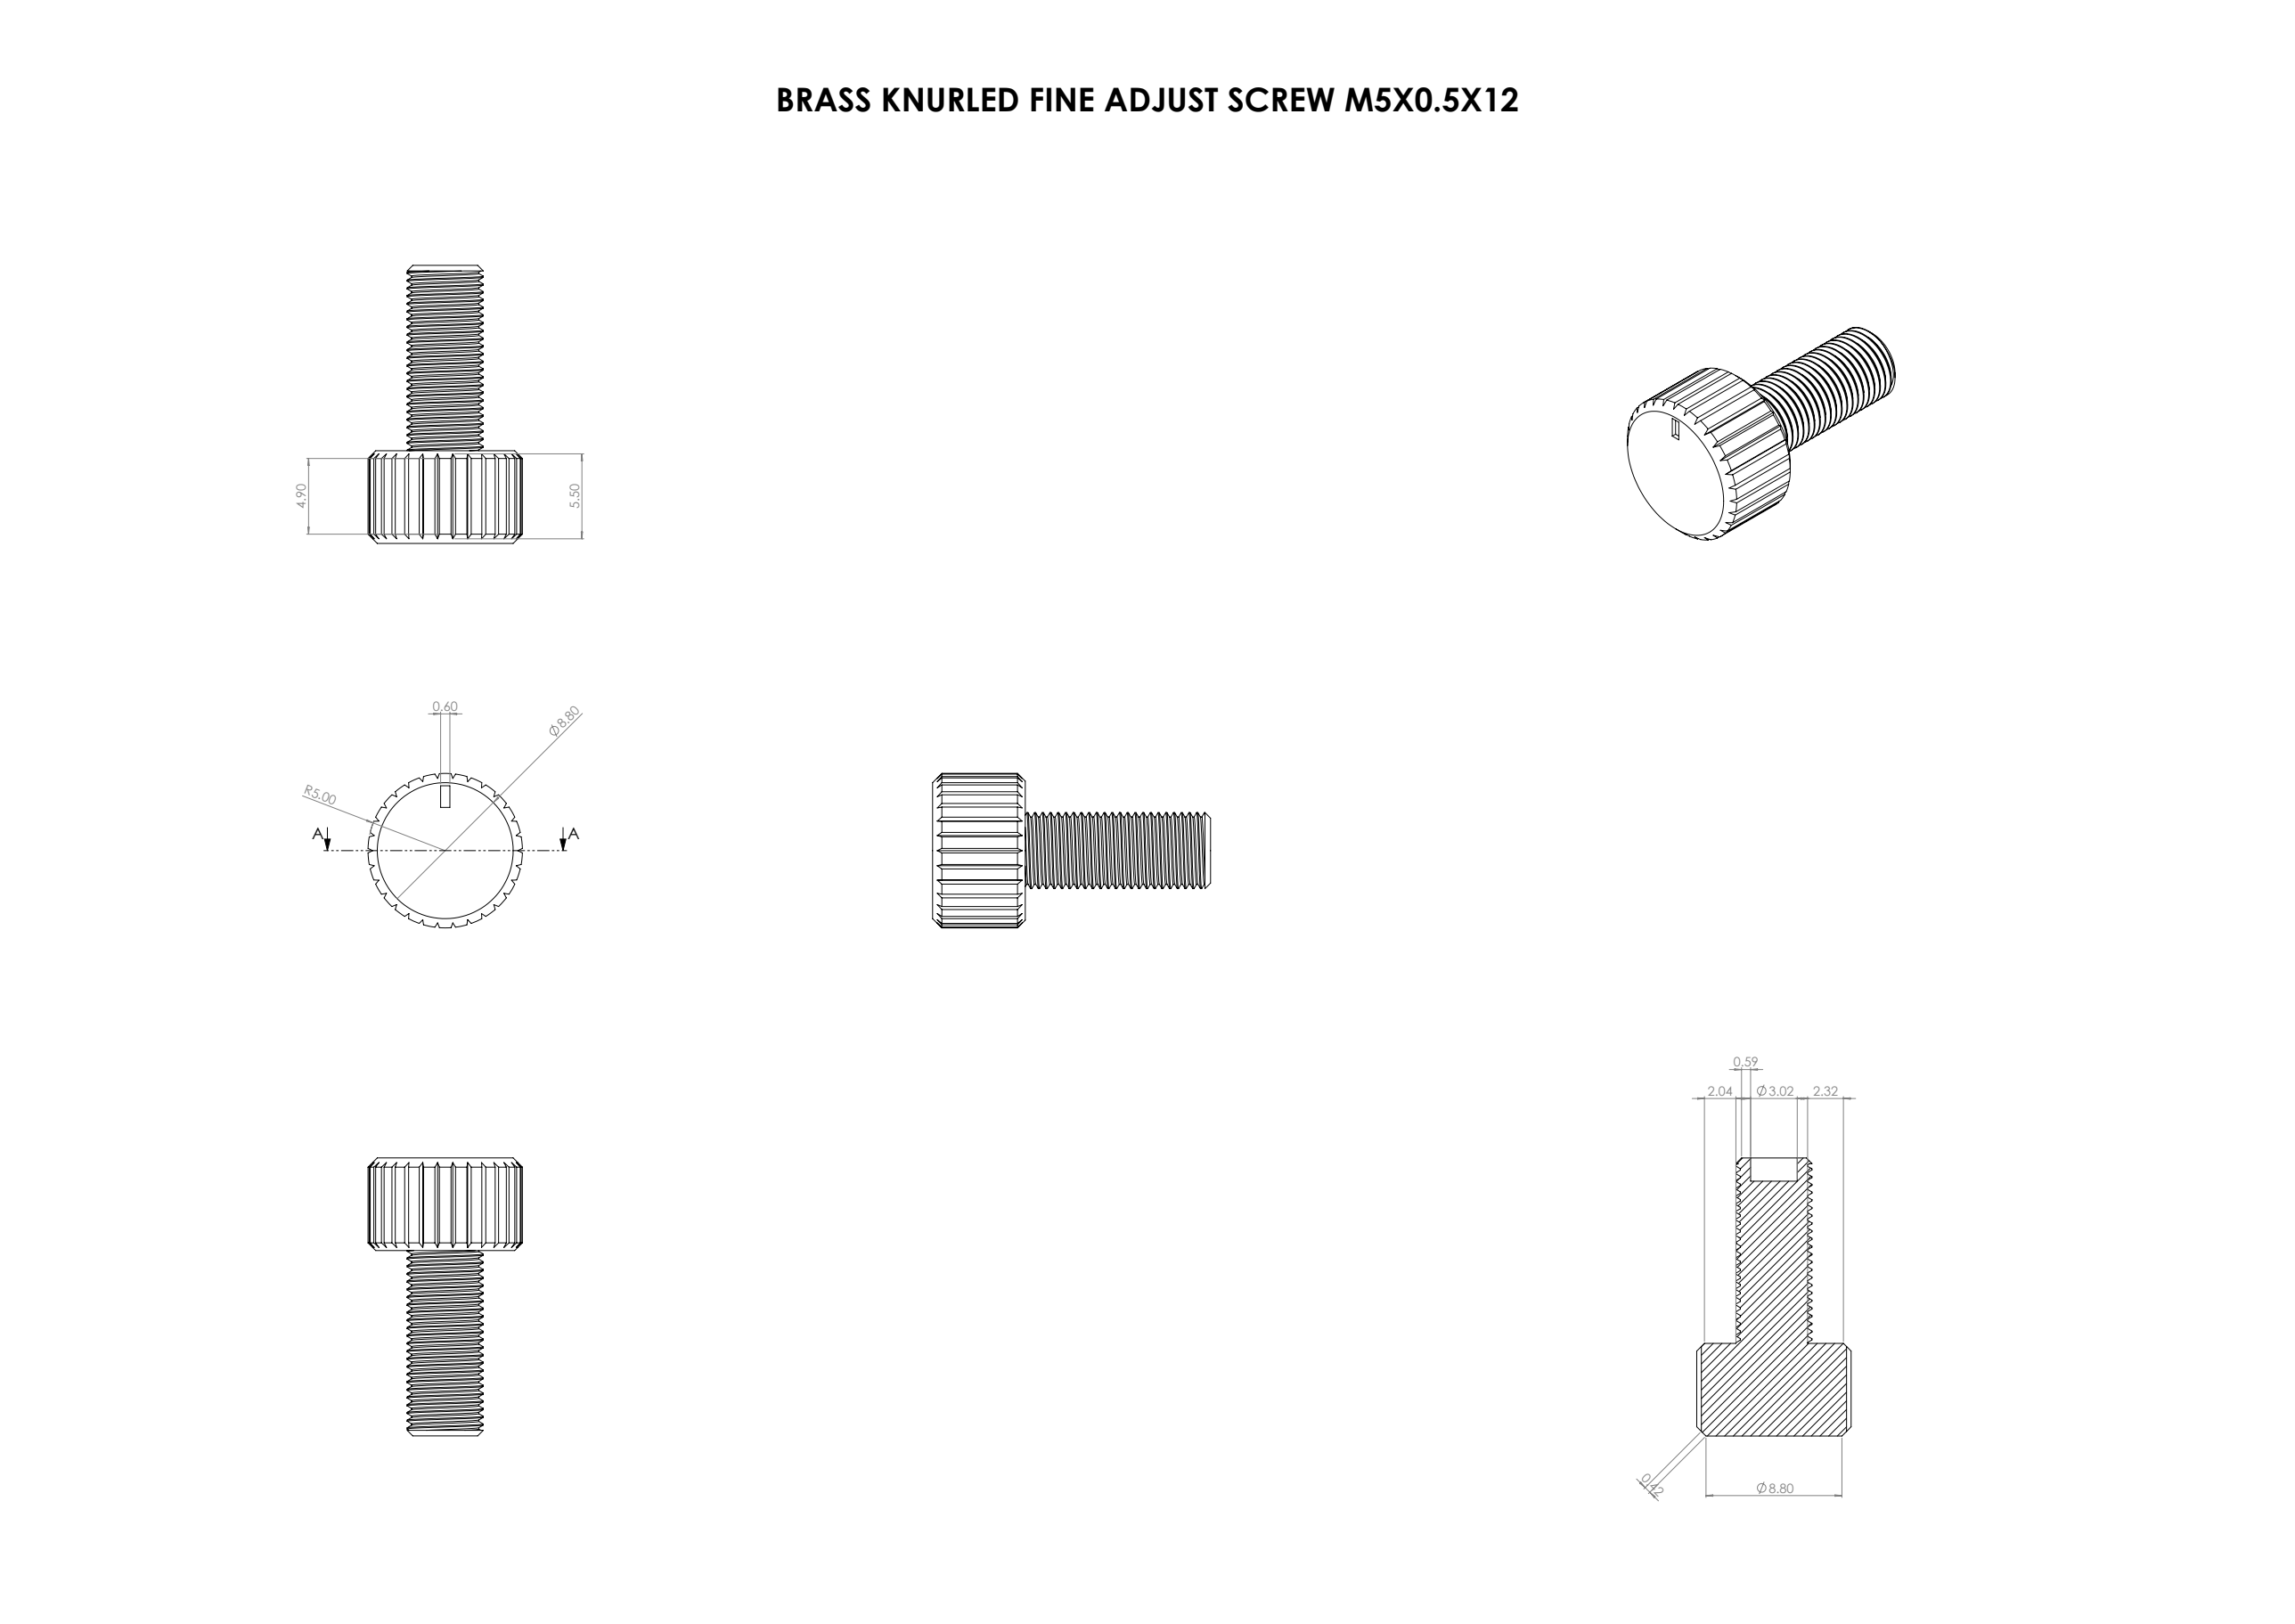
ISO-10303-21;
HEADER;
/* Generated by software containing ST-Developer
 * from STEP Tools, Inc. (www.steptools.com) 
 */

FILE_DESCRIPTION(
/* description */ (''),
/* implementation_level */ '2;1');

FILE_NAME(
/* name */ 
'08_Brass_Knurled_Fine_Adjust_Screw_M5x0.5x12.step',
/* time_stamp */ '2026-10-20T10:06:23-07:00',
/* author */ (''),
/* organization */ (''),
/* preprocessor_version */ 'ST-DEVELOPER v20.2',
/* originating_system */ 'Autodesk Translation Framework v15.15.0.0',
/* authorisation */ '');

FILE_SCHEMA (('AUTOMOTIVE_DESIGN { 1 0 10303 214 3 1 1 }'));
ENDSEC;

DATA;
#10=MECHANICAL_DESIGN_GEOMETRIC_PRESENTATION_REPRESENTATION('',(#469),#38611);
#132=(
BOUNDED_CURVE()
B_SPLINE_CURVE(2,(#30814,#30815,#30816),.UNSPECIFIED.,.F.,.F.)
B_SPLINE_CURVE_WITH_KNOTS((3,3),(0.0467199500563867,0.0898699663113549),
 .UNSPECIFIED.)
CURVE()
GEOMETRIC_REPRESENTATION_ITEM()
RATIONAL_B_SPLINE_CURVE((1.00126937543075,1.00122087809448,1.))
REPRESENTATION_ITEM('')
);
#133=(
BOUNDED_CURVE()
B_SPLINE_CURVE(2,(#30820,#30821,#30822),.UNSPECIFIED.,.F.,.F.)
B_SPLINE_CURVE_WITH_KNOTS((3,3),(0.,0.0436887632258073),.UNSPECIFIED.)
CURVE()
GEOMETRIC_REPRESENTATION_ITEM()
RATIONAL_B_SPLINE_CURVE((1.,1.00100330533763,1.00083425612165))
REPRESENTATION_ITEM('')
);
#134=(
BOUNDED_CURVE()
B_SPLINE_CURVE(2,(#30826,#30827,#30828),.UNSPECIFIED.,.F.,.F.)
B_SPLINE_CURVE_WITH_KNOTS((3,3),(0.,0.0431500162549626),.UNSPECIFIED.)
CURVE()
GEOMETRIC_REPRESENTATION_ITEM()
RATIONAL_B_SPLINE_CURVE((1.,1.00122087809439,1.00126937543066))
REPRESENTATION_ITEM('')
);
#135=(
BOUNDED_CURVE()
B_SPLINE_CURVE(2,(#30831,#30832,#30833),.UNSPECIFIED.,.F.,.F.)
B_SPLINE_CURVE_WITH_KNOTS((3,3),(0.0310892451912064,0.0747780084169829),
 .UNSPECIFIED.)
CURVE()
GEOMETRIC_REPRESENTATION_ITEM()
RATIONAL_B_SPLINE_CURVE((1.00083425612186,1.00100330533789,1.))
REPRESENTATION_ITEM('')
);
#136=(
BOUNDED_CURVE()
B_SPLINE_CURVE(2,(#30837,#30838,#30839),.UNSPECIFIED.,.F.,.F.)
B_SPLINE_CURVE_WITH_KNOTS((3,3),(0.0467199500564158,0.089869966311355),
 .UNSPECIFIED.)
CURVE()
GEOMETRIC_REPRESENTATION_ITEM()
RATIONAL_B_SPLINE_CURVE((1.00126937543096,1.00122087809468,1.))
REPRESENTATION_ITEM('')
);
#137=(
BOUNDED_CURVE()
B_SPLINE_CURVE(2,(#30843,#30844,#30845),.UNSPECIFIED.,.F.,.F.)
B_SPLINE_CURVE_WITH_KNOTS((3,3),(0.,0.043688763225805),.UNSPECIFIED.)
CURVE()
GEOMETRIC_REPRESENTATION_ITEM()
RATIONAL_B_SPLINE_CURVE((1.,1.00100330533789,1.00083425612186))
REPRESENTATION_ITEM('')
);
#138=(
BOUNDED_CURVE()
B_SPLINE_CURVE(2,(#30849,#30850,#30851),.UNSPECIFIED.,.F.,.F.)
B_SPLINE_CURVE_WITH_KNOTS((3,3),(0.,0.0431500162549483),.UNSPECIFIED.)
CURVE()
GEOMETRIC_REPRESENTATION_ITEM()
RATIONAL_B_SPLINE_CURVE((1.,1.00122087809469,1.00126937543097))
REPRESENTATION_ITEM('')
);
#139=(
BOUNDED_CURVE()
B_SPLINE_CURVE(2,(#30854,#30855,#30856),.UNSPECIFIED.,.F.,.F.)
B_SPLINE_CURVE_WITH_KNOTS((3,3),(0.0310892451911987,0.0747780084169828),
 .UNSPECIFIED.)
CURVE()
GEOMETRIC_REPRESENTATION_ITEM()
RATIONAL_B_SPLINE_CURVE((1.00083425612161,1.00100330533758,1.))
REPRESENTATION_ITEM('')
);
#140=(
BOUNDED_CURVE()
B_SPLINE_CURVE(2,(#30860,#30861,#30862),.UNSPECIFIED.,.F.,.F.)
B_SPLINE_CURVE_WITH_KNOTS((3,3),(0.0467199500563958,0.089869966311355),
 .UNSPECIFIED.)
CURVE()
GEOMETRIC_REPRESENTATION_ITEM()
RATIONAL_B_SPLINE_CURVE((1.00126937543073,1.00122087809446,1.))
REPRESENTATION_ITEM('')
);
#141=(
BOUNDED_CURVE()
B_SPLINE_CURVE(2,(#30866,#30867,#30868),.UNSPECIFIED.,.F.,.F.)
B_SPLINE_CURVE_WITH_KNOTS((3,3),(0.,0.0436887632258068),.UNSPECIFIED.)
CURVE()
GEOMETRIC_REPRESENTATION_ITEM()
RATIONAL_B_SPLINE_CURVE((1.,1.0010033053375,1.00083425612154))
REPRESENTATION_ITEM('')
);
#142=(
BOUNDED_CURVE()
B_SPLINE_CURVE(2,(#30872,#30873,#30874),.UNSPECIFIED.,.F.,.F.)
B_SPLINE_CURVE_WITH_KNOTS((3,3),(0.,0.0431500162549413),.UNSPECIFIED.)
CURVE()
GEOMETRIC_REPRESENTATION_ITEM()
RATIONAL_B_SPLINE_CURVE((1.,1.00122087809486,1.00126937543114))
REPRESENTATION_ITEM('')
);
#143=(
BOUNDED_CURVE()
B_SPLINE_CURVE(2,(#30877,#30878,#30879),.UNSPECIFIED.,.F.,.F.)
B_SPLINE_CURVE_WITH_KNOTS((3,3),(0.0310892451911471,0.0747780084169828),
 .UNSPECIFIED.)
CURVE()
GEOMETRIC_REPRESENTATION_ITEM()
RATIONAL_B_SPLINE_CURVE((1.00083425612202,1.00100330533808,1.))
REPRESENTATION_ITEM('')
);
#144=(
BOUNDED_CURVE()
B_SPLINE_CURVE(2,(#30883,#30884,#30885),.UNSPECIFIED.,.F.,.F.)
B_SPLINE_CURVE_WITH_KNOTS((3,3),(0.046719950056407,0.089869966311355),
 .UNSPECIFIED.)
CURVE()
GEOMETRIC_REPRESENTATION_ITEM()
RATIONAL_B_SPLINE_CURVE((1.00126937543088,1.0012208780946,1.))
REPRESENTATION_ITEM('')
);
#145=(
BOUNDED_CURVE()
B_SPLINE_CURVE(2,(#30889,#30890,#30891),.UNSPECIFIED.,.F.,.F.)
B_SPLINE_CURVE_WITH_KNOTS((3,3),(0.,0.0436887632257949),.UNSPECIFIED.)
CURVE()
GEOMETRIC_REPRESENTATION_ITEM()
RATIONAL_B_SPLINE_CURVE((1.,1.00100330533737,1.00083425612143))
REPRESENTATION_ITEM('')
);
#146=(
BOUNDED_CURVE()
B_SPLINE_CURVE(2,(#30895,#30896,#30897),.UNSPECIFIED.,.F.,.F.)
B_SPLINE_CURVE_WITH_KNOTS((3,3),(0.,0.0431500162549611),.UNSPECIFIED.)
CURVE()
GEOMETRIC_REPRESENTATION_ITEM()
RATIONAL_B_SPLINE_CURVE((1.,1.00122087809444,1.00126937543071))
REPRESENTATION_ITEM('')
);
#147=(
BOUNDED_CURVE()
B_SPLINE_CURVE(2,(#30900,#30901,#30902),.UNSPECIFIED.,.F.,.F.)
B_SPLINE_CURVE_WITH_KNOTS((3,3),(0.0310892451911564,0.0747780084169829),
 .UNSPECIFIED.)
CURVE()
GEOMETRIC_REPRESENTATION_ITEM()
RATIONAL_B_SPLINE_CURVE((1.00083425612184,1.00100330533786,1.))
REPRESENTATION_ITEM('')
);
#148=(
BOUNDED_CURVE()
B_SPLINE_CURVE(2,(#30906,#30907,#30908),.UNSPECIFIED.,.F.,.F.)
B_SPLINE_CURVE_WITH_KNOTS((3,3),(0.0467199500563991,0.089869966311355),
 .UNSPECIFIED.)
CURVE()
GEOMETRIC_REPRESENTATION_ITEM()
RATIONAL_B_SPLINE_CURVE((1.00126937543067,1.0012208780944,1.))
REPRESENTATION_ITEM('')
);
#149=(
BOUNDED_CURVE()
B_SPLINE_CURVE(2,(#30912,#30913,#30914),.UNSPECIFIED.,.F.,.F.)
B_SPLINE_CURVE_WITH_KNOTS((3,3),(0.,0.0436887632258358),.UNSPECIFIED.)
CURVE()
GEOMETRIC_REPRESENTATION_ITEM()
RATIONAL_B_SPLINE_CURVE((1.,1.0010033053379,1.00083425612187))
REPRESENTATION_ITEM('')
);
#150=(
BOUNDED_CURVE()
B_SPLINE_CURVE(2,(#30918,#30919,#30920),.UNSPECIFIED.,.F.,.F.)
B_SPLINE_CURVE_WITH_KNOTS((3,3),(0.,0.0431500162549541),.UNSPECIFIED.)
CURVE()
GEOMETRIC_REPRESENTATION_ITEM()
RATIONAL_B_SPLINE_CURVE((1.,1.00122087809508,1.00126937543137))
REPRESENTATION_ITEM('')
);
#151=(
BOUNDED_CURVE()
B_SPLINE_CURVE(2,(#30923,#30924,#30925),.UNSPECIFIED.,.F.,.F.)
B_SPLINE_CURVE_WITH_KNOTS((3,3),(0.0310892451911811,0.0747780084169827),
 .UNSPECIFIED.)
CURVE()
GEOMETRIC_REPRESENTATION_ITEM()
RATIONAL_B_SPLINE_CURVE((1.0008342561216,1.00100330533758,1.))
REPRESENTATION_ITEM('')
);
#152=(
BOUNDED_CURVE()
B_SPLINE_CURVE(2,(#30929,#30930,#30931),.UNSPECIFIED.,.F.,.F.)
B_SPLINE_CURVE_WITH_KNOTS((3,3),(0.0467199500563772,0.0898699663113549),
 .UNSPECIFIED.)
CURVE()
GEOMETRIC_REPRESENTATION_ITEM()
RATIONAL_B_SPLINE_CURVE((1.00126937543116,1.00122087809487,1.))
REPRESENTATION_ITEM('')
);
#153=(
BOUNDED_CURVE()
B_SPLINE_CURVE(2,(#30935,#30936,#30937),.UNSPECIFIED.,.F.,.F.)
B_SPLINE_CURVE_WITH_KNOTS((3,3),(0.,0.0436887632258276),.UNSPECIFIED.)
CURVE()
GEOMETRIC_REPRESENTATION_ITEM()
RATIONAL_B_SPLINE_CURVE((1.,1.00100330533759,1.00083425612161))
REPRESENTATION_ITEM('')
);
#154=(
BOUNDED_CURVE()
B_SPLINE_CURVE(2,(#30941,#30942,#30943),.UNSPECIFIED.,.F.,.F.)
B_SPLINE_CURVE_WITH_KNOTS((3,3),(0.,0.0431500162549563),.UNSPECIFIED.)
CURVE()
GEOMETRIC_REPRESENTATION_ITEM()
RATIONAL_B_SPLINE_CURVE((1.,1.00122087809465,1.00126937543093))
REPRESENTATION_ITEM('')
);
#155=(
BOUNDED_CURVE()
B_SPLINE_CURVE(2,(#30946,#30947,#30948),.UNSPECIFIED.,.F.,.F.)
B_SPLINE_CURVE_WITH_KNOTS((3,3),(0.0310892451911613,0.0747780084169828),
 .UNSPECIFIED.)
CURVE()
GEOMETRIC_REPRESENTATION_ITEM()
RATIONAL_B_SPLINE_CURVE((1.00083425612131,1.00100330533723,1.))
REPRESENTATION_ITEM('')
);
#156=(
BOUNDED_CURVE()
B_SPLINE_CURVE(2,(#30952,#30953,#30954),.UNSPECIFIED.,.F.,.F.)
B_SPLINE_CURVE_WITH_KNOTS((3,3),(0.0467199500563946,0.0898699663113547),
 .UNSPECIFIED.)
CURVE()
GEOMETRIC_REPRESENTATION_ITEM()
RATIONAL_B_SPLINE_CURVE((1.00126937543097,1.00122087809469,1.))
REPRESENTATION_ITEM('')
);
#157=(
BOUNDED_CURVE()
B_SPLINE_CURVE(2,(#30958,#30959,#30960),.UNSPECIFIED.,.F.,.F.)
B_SPLINE_CURVE_WITH_KNOTS((3,3),(0.,0.0436887632258045),.UNSPECIFIED.)
CURVE()
GEOMETRIC_REPRESENTATION_ITEM()
RATIONAL_B_SPLINE_CURVE((1.,1.00100330533793,1.00083425612189))
REPRESENTATION_ITEM('')
);
#158=(
BOUNDED_CURVE()
B_SPLINE_CURVE(2,(#30964,#30965,#30966),.UNSPECIFIED.,.F.,.F.)
B_SPLINE_CURVE_WITH_KNOTS((3,3),(0.,0.0431500162549573),.UNSPECIFIED.)
CURVE()
GEOMETRIC_REPRESENTATION_ITEM()
RATIONAL_B_SPLINE_CURVE((1.,1.00122087809474,1.00126937543102))
REPRESENTATION_ITEM('')
);
#159=(
BOUNDED_CURVE()
B_SPLINE_CURVE(2,(#30969,#30970,#30971),.UNSPECIFIED.,.F.,.F.)
B_SPLINE_CURVE_WITH_KNOTS((3,3),(0.0310892451911831,0.074778008416983),
 .UNSPECIFIED.)
CURVE()
GEOMETRIC_REPRESENTATION_ITEM()
RATIONAL_B_SPLINE_CURVE((1.00083425612233,1.00100330533846,1.))
REPRESENTATION_ITEM('')
);
#160=(
BOUNDED_CURVE()
B_SPLINE_CURVE(2,(#30975,#30976,#30977),.UNSPECIFIED.,.F.,.F.)
B_SPLINE_CURVE_WITH_KNOTS((3,3),(0.0467199500564136,0.0898699663113549),
 .UNSPECIFIED.)
CURVE()
GEOMETRIC_REPRESENTATION_ITEM()
RATIONAL_B_SPLINE_CURVE((1.00126937543068,1.00122087809441,1.))
REPRESENTATION_ITEM('')
);
#161=(
BOUNDED_CURVE()
B_SPLINE_CURVE(2,(#30981,#30982,#30983),.UNSPECIFIED.,.F.,.F.)
B_SPLINE_CURVE_WITH_KNOTS((3,3),(0.,0.0436887632258141),.UNSPECIFIED.)
CURVE()
GEOMETRIC_REPRESENTATION_ITEM()
RATIONAL_B_SPLINE_CURVE((1.,1.00100330533752,1.00083425612155))
REPRESENTATION_ITEM('')
);
#162=(
BOUNDED_CURVE()
B_SPLINE_CURVE(2,(#30987,#30988,#30989),.UNSPECIFIED.,.F.,.F.)
B_SPLINE_CURVE_WITH_KNOTS((3,3),(0.,0.0431500162549441),.UNSPECIFIED.)
CURVE()
GEOMETRIC_REPRESENTATION_ITEM()
RATIONAL_B_SPLINE_CURVE((1.,1.00122087809436,1.00126937543063))
REPRESENTATION_ITEM('')
);
#163=(
BOUNDED_CURVE()
B_SPLINE_CURVE(2,(#30992,#30993,#30994),.UNSPECIFIED.,.F.,.F.)
B_SPLINE_CURVE_WITH_KNOTS((3,3),(0.0310892451911682,0.0747780084169828),
 .UNSPECIFIED.)
CURVE()
GEOMETRIC_REPRESENTATION_ITEM()
RATIONAL_B_SPLINE_CURVE((1.00083425612141,1.00100330533735,1.))
REPRESENTATION_ITEM('')
);
#164=(
BOUNDED_CURVE()
B_SPLINE_CURVE(2,(#30998,#30999,#31000),.UNSPECIFIED.,.F.,.F.)
B_SPLINE_CURVE_WITH_KNOTS((3,3),(0.0467199500564218,0.0898699663113548),
 .UNSPECIFIED.)
CURVE()
GEOMETRIC_REPRESENTATION_ITEM()
RATIONAL_B_SPLINE_CURVE((1.00126937543122,1.00122087809493,1.))
REPRESENTATION_ITEM('')
);
#165=(
BOUNDED_CURVE()
B_SPLINE_CURVE(2,(#31004,#31005,#31006),.UNSPECIFIED.,.F.,.F.)
B_SPLINE_CURVE_WITH_KNOTS((3,3),(0.,0.0436887632257843),.UNSPECIFIED.)
CURVE()
GEOMETRIC_REPRESENTATION_ITEM()
RATIONAL_B_SPLINE_CURVE((1.,1.00100330533799,1.00083425612195))
REPRESENTATION_ITEM('')
);
#166=(
BOUNDED_CURVE()
B_SPLINE_CURVE(2,(#31010,#31011,#31012),.UNSPECIFIED.,.F.,.F.)
B_SPLINE_CURVE_WITH_KNOTS((3,3),(0.,0.0431500162549522),.UNSPECIFIED.)
CURVE()
GEOMETRIC_REPRESENTATION_ITEM()
RATIONAL_B_SPLINE_CURVE((1.,1.00122087809455,1.00126937543082))
REPRESENTATION_ITEM('')
);
#167=(
BOUNDED_CURVE()
B_SPLINE_CURVE(2,(#31015,#31016,#31017),.UNSPECIFIED.,.F.,.F.)
B_SPLINE_CURVE_WITH_KNOTS((3,3),(0.0310892451912127,0.0747780084169828),
 .UNSPECIFIED.)
CURVE()
GEOMETRIC_REPRESENTATION_ITEM()
RATIONAL_B_SPLINE_CURVE((1.000834256122,1.00100330533806,1.))
REPRESENTATION_ITEM('')
);
#168=(
BOUNDED_CURVE()
B_SPLINE_CURVE(2,(#31021,#31022,#31023),.UNSPECIFIED.,.F.,.F.)
B_SPLINE_CURVE_WITH_KNOTS((3,3),(0.046719950056375,0.0898699663113549),
 .UNSPECIFIED.)
CURVE()
GEOMETRIC_REPRESENTATION_ITEM()
RATIONAL_B_SPLINE_CURVE((1.00126937543081,1.00122087809453,1.))
REPRESENTATION_ITEM('')
);
#169=(
BOUNDED_CURVE()
B_SPLINE_CURVE(2,(#31027,#31028,#31029),.UNSPECIFIED.,.F.,.F.)
B_SPLINE_CURVE_WITH_KNOTS((3,3),(0.,0.043688763225798),.UNSPECIFIED.)
CURVE()
GEOMETRIC_REPRESENTATION_ITEM()
RATIONAL_B_SPLINE_CURVE((1.,1.00100330533766,1.00083425612167))
REPRESENTATION_ITEM('')
);
#170=(
BOUNDED_CURVE()
B_SPLINE_CURVE(2,(#31033,#31034,#31035),.UNSPECIFIED.,.F.,.F.)
B_SPLINE_CURVE_WITH_KNOTS((3,3),(0.,0.0431500162549388),.UNSPECIFIED.)
CURVE()
GEOMETRIC_REPRESENTATION_ITEM()
RATIONAL_B_SPLINE_CURVE((1.,1.00122087809441,1.00126937543068))
REPRESENTATION_ITEM('')
);
#171=(
BOUNDED_CURVE()
B_SPLINE_CURVE(2,(#31038,#31039,#31040),.UNSPECIFIED.,.F.,.F.)
B_SPLINE_CURVE_WITH_KNOTS((3,3),(0.031089245191172,0.0747780084169828),
 .UNSPECIFIED.)
CURVE()
GEOMETRIC_REPRESENTATION_ITEM()
RATIONAL_B_SPLINE_CURVE((1.00083425612203,1.00100330533809,1.))
REPRESENTATION_ITEM('')
);
#172=(
BOUNDED_CURVE()
B_SPLINE_CURVE(2,(#31044,#31045,#31046),.UNSPECIFIED.,.F.,.F.)
B_SPLINE_CURVE_WITH_KNOTS((3,3),(0.0467199500564012,0.0898699663113549),
 .UNSPECIFIED.)
CURVE()
GEOMETRIC_REPRESENTATION_ITEM()
RATIONAL_B_SPLINE_CURVE((1.00126937543067,1.00122087809441,1.))
REPRESENTATION_ITEM('')
);
#173=(
BOUNDED_CURVE()
B_SPLINE_CURVE(2,(#31050,#31051,#31052),.UNSPECIFIED.,.F.,.F.)
B_SPLINE_CURVE_WITH_KNOTS((3,3),(0.,0.0436887632258383),.UNSPECIFIED.)
CURVE()
GEOMETRIC_REPRESENTATION_ITEM()
RATIONAL_B_SPLINE_CURVE((1.,1.00100330533736,1.00083425612142))
REPRESENTATION_ITEM('')
);
#174=(
BOUNDED_CURVE()
B_SPLINE_CURVE(2,(#31056,#31057,#31058),.UNSPECIFIED.,.F.,.F.)
B_SPLINE_CURVE_WITH_KNOTS((3,3),(0.,0.0431500162549534),.UNSPECIFIED.)
CURVE()
GEOMETRIC_REPRESENTATION_ITEM()
RATIONAL_B_SPLINE_CURVE((1.,1.00122087809426,1.00126937543052))
REPRESENTATION_ITEM('')
);
#175=(
BOUNDED_CURVE()
B_SPLINE_CURVE(2,(#31061,#31062,#31063),.UNSPECIFIED.,.F.,.F.)
B_SPLINE_CURVE_WITH_KNOTS((3,3),(0.0310892451911742,0.074778008416983),
 .UNSPECIFIED.)
CURVE()
GEOMETRIC_REPRESENTATION_ITEM()
RATIONAL_B_SPLINE_CURVE((1.00083425612157,1.00100330533753,1.))
REPRESENTATION_ITEM('')
);
#176=(
BOUNDED_CURVE()
B_SPLINE_CURVE(2,(#31067,#31068,#31069),.UNSPECIFIED.,.F.,.F.)
B_SPLINE_CURVE_WITH_KNOTS((3,3),(0.0467199500564228,0.0898699663113548),
 .UNSPECIFIED.)
CURVE()
GEOMETRIC_REPRESENTATION_ITEM()
RATIONAL_B_SPLINE_CURVE((1.00126937543075,1.00122087809448,1.))
REPRESENTATION_ITEM('')
);
#177=(
BOUNDED_CURVE()
B_SPLINE_CURVE(2,(#31073,#31074,#31075),.UNSPECIFIED.,.F.,.F.)
B_SPLINE_CURVE_WITH_KNOTS((3,3),(0.,0.0436887632258167),.UNSPECIFIED.)
CURVE()
GEOMETRIC_REPRESENTATION_ITEM()
RATIONAL_B_SPLINE_CURVE((1.,1.0010033053373,1.00083425612137))
REPRESENTATION_ITEM('')
);
#178=(
BOUNDED_CURVE()
B_SPLINE_CURVE(2,(#31079,#31080,#31081),.UNSPECIFIED.,.F.,.F.)
B_SPLINE_CURVE_WITH_KNOTS((3,3),(0.,0.0431500162549855),.UNSPECIFIED.)
CURVE()
GEOMETRIC_REPRESENTATION_ITEM()
RATIONAL_B_SPLINE_CURVE((1.,1.00122087809442,1.00126937543069))
REPRESENTATION_ITEM('')
);
#179=(
BOUNDED_CURVE()
B_SPLINE_CURVE(2,(#31084,#31085,#31086),.UNSPECIFIED.,.F.,.F.)
B_SPLINE_CURVE_WITH_KNOTS((3,3),(0.0310892451911962,0.0747780084169828),
 .UNSPECIFIED.)
CURVE()
GEOMETRIC_REPRESENTATION_ITEM()
RATIONAL_B_SPLINE_CURVE((1.00083425612222,1.00100330533831,1.))
REPRESENTATION_ITEM('')
);
#180=(
BOUNDED_CURVE()
B_SPLINE_CURVE(2,(#31090,#31091,#31092),.UNSPECIFIED.,.F.,.F.)
B_SPLINE_CURVE_WITH_KNOTS((3,3),(0.0467199500564075,0.0898699663113548),
 .UNSPECIFIED.)
CURVE()
GEOMETRIC_REPRESENTATION_ITEM()
RATIONAL_B_SPLINE_CURVE((1.00126937543101,1.00122087809473,1.))
REPRESENTATION_ITEM('')
);
#181=(
BOUNDED_CURVE()
B_SPLINE_CURVE(2,(#31096,#31097,#31098),.UNSPECIFIED.,.F.,.F.)
B_SPLINE_CURVE_WITH_KNOTS((3,3),(0.,0.0436887632257957),.UNSPECIFIED.)
CURVE()
GEOMETRIC_REPRESENTATION_ITEM()
RATIONAL_B_SPLINE_CURVE((1.,1.00100330533777,1.00083425612177))
REPRESENTATION_ITEM('')
);
#182=(
BOUNDED_CURVE()
B_SPLINE_CURVE(2,(#31102,#31103,#31104),.UNSPECIFIED.,.F.,.F.)
B_SPLINE_CURVE_WITH_KNOTS((3,3),(0.,0.0431500162549319),.UNSPECIFIED.)
CURVE()
GEOMETRIC_REPRESENTATION_ITEM()
RATIONAL_B_SPLINE_CURVE((1.,1.00122087809489,1.00126937543118))
REPRESENTATION_ITEM('')
);
#183=(
BOUNDED_CURVE()
B_SPLINE_CURVE(2,(#31107,#31108,#31109),.UNSPECIFIED.,.F.,.F.)
B_SPLINE_CURVE_WITH_KNOTS((3,3),(0.0310892451911674,0.0747780084169828),
 .UNSPECIFIED.)
CURVE()
GEOMETRIC_REPRESENTATION_ITEM()
RATIONAL_B_SPLINE_CURVE((1.00083425612107,1.00100330533693,1.))
REPRESENTATION_ITEM('')
);
#184=(
BOUNDED_CURVE()
B_SPLINE_CURVE(2,(#31113,#31114,#31115),.UNSPECIFIED.,.F.,.F.)
B_SPLINE_CURVE_WITH_KNOTS((3,3),(0.0467199500564182,0.0898699663113548),
 .UNSPECIFIED.)
CURVE()
GEOMETRIC_REPRESENTATION_ITEM()
RATIONAL_B_SPLINE_CURVE((1.00126937543111,1.00122087809482,1.))
REPRESENTATION_ITEM('')
);
#185=(
BOUNDED_CURVE()
B_SPLINE_CURVE(2,(#31119,#31120,#31121),.UNSPECIFIED.,.F.,.F.)
B_SPLINE_CURVE_WITH_KNOTS((3,3),(0.,0.0436887632258121),.UNSPECIFIED.)
CURVE()
GEOMETRIC_REPRESENTATION_ITEM()
RATIONAL_B_SPLINE_CURVE((1.,1.00100330533764,1.00083425612165))
REPRESENTATION_ITEM('')
);
#186=(
BOUNDED_CURVE()
B_SPLINE_CURVE(2,(#31125,#31126,#31127),.UNSPECIFIED.,.F.,.F.)
B_SPLINE_CURVE_WITH_KNOTS((3,3),(0.,0.0431500162549636),.UNSPECIFIED.)
CURVE()
GEOMETRIC_REPRESENTATION_ITEM()
RATIONAL_B_SPLINE_CURVE((1.,1.0012208780943,1.00126937543056))
REPRESENTATION_ITEM('')
);
#187=(
BOUNDED_CURVE()
B_SPLINE_CURVE(2,(#31130,#31131,#31132),.UNSPECIFIED.,.F.,.F.)
B_SPLINE_CURVE_WITH_KNOTS((3,3),(0.0310892451911629,0.0747780084169827),
 .UNSPECIFIED.)
CURVE()
GEOMETRIC_REPRESENTATION_ITEM()
RATIONAL_B_SPLINE_CURVE((1.00083425612137,1.0010033053373,1.))
REPRESENTATION_ITEM('')
);
#188=(
BOUNDED_CURVE()
B_SPLINE_CURVE(2,(#31136,#31137,#31138),.UNSPECIFIED.,.F.,.F.)
B_SPLINE_CURVE_WITH_KNOTS((3,3),(0.0467199500564021,0.0898699663113548),
 .UNSPECIFIED.)
CURVE()
GEOMETRIC_REPRESENTATION_ITEM()
RATIONAL_B_SPLINE_CURVE((1.00126937543099,1.00122087809471,1.))
REPRESENTATION_ITEM('')
);
#189=(
BOUNDED_CURVE()
B_SPLINE_CURVE(2,(#31142,#31143,#31144),.UNSPECIFIED.,.F.,.F.)
B_SPLINE_CURVE_WITH_KNOTS((3,3),(0.,0.0436887632258091),.UNSPECIFIED.)
CURVE()
GEOMETRIC_REPRESENTATION_ITEM()
RATIONAL_B_SPLINE_CURVE((1.,1.00100330533755,1.00083425612158))
REPRESENTATION_ITEM('')
);
#190=(
BOUNDED_CURVE()
B_SPLINE_CURVE(2,(#31148,#31149,#31150),.UNSPECIFIED.,.F.,.F.)
B_SPLINE_CURVE_WITH_KNOTS((3,3),(0.,0.0431500162549568),.UNSPECIFIED.)
CURVE()
GEOMETRIC_REPRESENTATION_ITEM()
RATIONAL_B_SPLINE_CURVE((1.,1.00122087809472,1.00126937543101))
REPRESENTATION_ITEM('')
);
#191=(
BOUNDED_CURVE()
B_SPLINE_CURVE(2,(#31153,#31154,#31155),.UNSPECIFIED.,.F.,.F.)
B_SPLINE_CURVE_WITH_KNOTS((3,3),(0.0310892451911866,0.0747780084169829),
 .UNSPECIFIED.)
CURVE()
GEOMETRIC_REPRESENTATION_ITEM()
RATIONAL_B_SPLINE_CURVE((1.0008342561218,1.00100330533782,1.))
REPRESENTATION_ITEM('')
);
#192=(
BOUNDED_CURVE()
B_SPLINE_CURVE(2,(#31159,#31160,#31161),.UNSPECIFIED.,.F.,.F.)
B_SPLINE_CURVE_WITH_KNOTS((3,3),(0.0467199500564191,0.0898699663113548),
 .UNSPECIFIED.)
CURVE()
GEOMETRIC_REPRESENTATION_ITEM()
RATIONAL_B_SPLINE_CURVE((1.00126937543092,1.00122087809464,1.))
REPRESENTATION_ITEM('')
);
#193=(
BOUNDED_CURVE()
B_SPLINE_CURVE(2,(#31165,#31166,#31167),.UNSPECIFIED.,.F.,.F.)
B_SPLINE_CURVE_WITH_KNOTS((3,3),(0.,0.0436887632257914),.UNSPECIFIED.)
CURVE()
GEOMETRIC_REPRESENTATION_ITEM()
RATIONAL_B_SPLINE_CURVE((1.,1.00100330533698,1.0008342561211))
REPRESENTATION_ITEM('')
);
#194=(
BOUNDED_CURVE()
B_SPLINE_CURVE(2,(#31171,#31172,#31173),.UNSPECIFIED.,.F.,.F.)
B_SPLINE_CURVE_WITH_KNOTS((3,3),(0.,0.0431500162549322),.UNSPECIFIED.)
CURVE()
GEOMETRIC_REPRESENTATION_ITEM()
RATIONAL_B_SPLINE_CURVE((1.,1.00122087809449,1.00126937543076))
REPRESENTATION_ITEM('')
);
#195=(
BOUNDED_CURVE()
B_SPLINE_CURVE(2,(#31176,#31177,#31178),.UNSPECIFIED.,.F.,.F.)
B_SPLINE_CURVE_WITH_KNOTS((3,3),(0.0310892451911953,0.0747780084169828),
 .UNSPECIFIED.)
CURVE()
GEOMETRIC_REPRESENTATION_ITEM()
RATIONAL_B_SPLINE_CURVE((1.0008342561224,1.00100330533854,1.))
REPRESENTATION_ITEM('')
);
#196=(
BOUNDED_CURVE()
B_SPLINE_CURVE(2,(#31182,#31183,#31184),.UNSPECIFIED.,.F.,.F.)
B_SPLINE_CURVE_WITH_KNOTS((3,3),(0.0467199500564009,0.0898699663113548),
 .UNSPECIFIED.)
CURVE()
GEOMETRIC_REPRESENTATION_ITEM()
RATIONAL_B_SPLINE_CURVE((1.00126937543082,1.00122087809454,1.))
REPRESENTATION_ITEM('')
);
#197=(
BOUNDED_CURVE()
B_SPLINE_CURVE(2,(#31188,#31189,#31190),.UNSPECIFIED.,.F.,.F.)
B_SPLINE_CURVE_WITH_KNOTS((3,3),(0.,0.04368876322581),.UNSPECIFIED.)
CURVE()
GEOMETRIC_REPRESENTATION_ITEM()
RATIONAL_B_SPLINE_CURVE((1.,1.00100330533771,1.00083425612171))
REPRESENTATION_ITEM('')
);
#198=(
BOUNDED_CURVE()
B_SPLINE_CURVE(2,(#31194,#31195,#31196),.UNSPECIFIED.,.F.,.F.)
B_SPLINE_CURVE_WITH_KNOTS((3,3),(0.,0.0431500162549717),.UNSPECIFIED.)
CURVE()
GEOMETRIC_REPRESENTATION_ITEM()
RATIONAL_B_SPLINE_CURVE((1.,1.00122087809461,1.00126937543088))
REPRESENTATION_ITEM('')
);
#199=(
BOUNDED_CURVE()
B_SPLINE_CURVE(2,(#31199,#31200,#31201),.UNSPECIFIED.,.F.,.F.)
B_SPLINE_CURVE_WITH_KNOTS((3,3),(0.0310892451911806,0.0747780084169829),
 .UNSPECIFIED.)
CURVE()
GEOMETRIC_REPRESENTATION_ITEM()
RATIONAL_B_SPLINE_CURVE((1.00083425612159,1.00100330533756,1.))
REPRESENTATION_ITEM('')
);
#200=(
BOUNDED_CURVE()
B_SPLINE_CURVE(2,(#31205,#31206,#31207),.UNSPECIFIED.,.F.,.F.)
B_SPLINE_CURVE_WITH_KNOTS((3,3),(0.0467199500564204,0.0898699663113548),
 .UNSPECIFIED.)
CURVE()
GEOMETRIC_REPRESENTATION_ITEM()
RATIONAL_B_SPLINE_CURVE((1.00126937543083,1.00122087809455,1.))
REPRESENTATION_ITEM('')
);
#201=(
BOUNDED_CURVE()
B_SPLINE_CURVE(2,(#31211,#31212,#31213),.UNSPECIFIED.,.F.,.F.)
B_SPLINE_CURVE_WITH_KNOTS((3,3),(0.,0.0436887632258064),.UNSPECIFIED.)
CURVE()
GEOMETRIC_REPRESENTATION_ITEM()
RATIONAL_B_SPLINE_CURVE((1.,1.00100330533703,1.00083425612115))
REPRESENTATION_ITEM('')
);
#202=(
BOUNDED_CURVE()
B_SPLINE_CURVE(2,(#31217,#31218,#31219),.UNSPECIFIED.,.F.,.F.)
B_SPLINE_CURVE_WITH_KNOTS((3,3),(0.,0.0431500162549232),.UNSPECIFIED.)
CURVE()
GEOMETRIC_REPRESENTATION_ITEM()
RATIONAL_B_SPLINE_CURVE((1.,1.00122087809502,1.00126937543132))
REPRESENTATION_ITEM('')
);
#203=(
BOUNDED_CURVE()
B_SPLINE_CURVE(2,(#31222,#31223,#31224),.UNSPECIFIED.,.F.,.F.)
B_SPLINE_CURVE_WITH_KNOTS((3,3),(0.0310892451911708,0.0747780084169828),
 .UNSPECIFIED.)
CURVE()
GEOMETRIC_REPRESENTATION_ITEM()
RATIONAL_B_SPLINE_CURVE((1.00083425612115,1.00100330533704,1.))
REPRESENTATION_ITEM('')
);
#204=(
BOUNDED_CURVE()
B_SPLINE_CURVE(2,(#31228,#31229,#31230),.UNSPECIFIED.,.F.,.F.)
B_SPLINE_CURVE_WITH_KNOTS((3,3),(0.04671995005641,0.0898699663113547),
 .UNSPECIFIED.)
CURVE()
GEOMETRIC_REPRESENTATION_ITEM()
RATIONAL_B_SPLINE_CURVE((1.00126937543045,1.00122087809419,1.))
REPRESENTATION_ITEM('')
);
#205=(
BOUNDED_CURVE()
B_SPLINE_CURVE(2,(#31234,#31235,#31236),.UNSPECIFIED.,.F.,.F.)
B_SPLINE_CURVE_WITH_KNOTS((3,3),(0.,0.0436887632258215),.UNSPECIFIED.)
CURVE()
GEOMETRIC_REPRESENTATION_ITEM()
RATIONAL_B_SPLINE_CURVE((1.,1.00100330533736,1.00083425612143))
REPRESENTATION_ITEM('')
);
#206=(
BOUNDED_CURVE()
B_SPLINE_CURVE(2,(#31240,#31241,#31242),.UNSPECIFIED.,.F.,.F.)
B_SPLINE_CURVE_WITH_KNOTS((3,3),(0.,0.0431500162549405),.UNSPECIFIED.)
CURVE()
GEOMETRIC_REPRESENTATION_ITEM()
RATIONAL_B_SPLINE_CURVE((1.,1.00122087809483,1.00126937543112))
REPRESENTATION_ITEM('')
);
#207=(
BOUNDED_CURVE()
B_SPLINE_CURVE(2,(#31245,#31246,#31247),.UNSPECIFIED.,.F.,.F.)
B_SPLINE_CURVE_WITH_KNOTS((3,3),(0.0310892451911933,0.0747780084169829),
 .UNSPECIFIED.)
CURVE()
GEOMETRIC_REPRESENTATION_ITEM()
RATIONAL_B_SPLINE_CURVE((1.00083425612156,1.00100330533752,1.))
REPRESENTATION_ITEM('')
);
#208=(
BOUNDED_CURVE()
B_SPLINE_CURVE(2,(#31251,#31252,#31253),.UNSPECIFIED.,.F.,.F.)
B_SPLINE_CURVE_WITH_KNOTS((3,3),(0.0467199500564031,0.0898699663113549),
 .UNSPECIFIED.)
CURVE()
GEOMETRIC_REPRESENTATION_ITEM()
RATIONAL_B_SPLINE_CURVE((1.00126937543121,1.00122087809492,1.))
REPRESENTATION_ITEM('')
);
#209=(
BOUNDED_CURVE()
B_SPLINE_CURVE(2,(#31257,#31258,#31259),.UNSPECIFIED.,.F.,.F.)
B_SPLINE_CURVE_WITH_KNOTS((3,3),(0.,0.0436887632258158),.UNSPECIFIED.)
CURVE()
GEOMETRIC_REPRESENTATION_ITEM()
RATIONAL_B_SPLINE_CURVE((1.,1.0010033053384,1.00083425612229))
REPRESENTATION_ITEM('')
);
#210=(
BOUNDED_CURVE()
B_SPLINE_CURVE(2,(#31263,#31264,#31265),.UNSPECIFIED.,.F.,.F.)
B_SPLINE_CURVE_WITH_KNOTS((3,3),(0.,0.0431500162549452),.UNSPECIFIED.)
CURVE()
GEOMETRIC_REPRESENTATION_ITEM()
RATIONAL_B_SPLINE_CURVE((1.,1.00122087809455,1.00126937543082))
REPRESENTATION_ITEM('')
);
#211=(
BOUNDED_CURVE()
B_SPLINE_CURVE(2,(#31268,#31269,#31270),.UNSPECIFIED.,.F.,.F.)
B_SPLINE_CURVE_WITH_KNOTS((3,3),(0.0310892451911938,0.0747780084169828),
 .UNSPECIFIED.)
CURVE()
GEOMETRIC_REPRESENTATION_ITEM()
RATIONAL_B_SPLINE_CURVE((1.00083425612169,1.00100330533769,1.))
REPRESENTATION_ITEM('')
);
#212=(
BOUNDED_CURVE()
B_SPLINE_CURVE(2,(#31274,#31275,#31276),.UNSPECIFIED.,.F.,.F.)
B_SPLINE_CURVE_WITH_KNOTS((3,3),(0.0467199500564215,0.0898699663113548),
 .UNSPECIFIED.)
CURVE()
GEOMETRIC_REPRESENTATION_ITEM()
RATIONAL_B_SPLINE_CURVE((1.00126937543076,1.00122087809448,1.))
REPRESENTATION_ITEM('')
);
#213=(
BOUNDED_CURVE()
B_SPLINE_CURVE(2,(#31280,#31281,#31282),.UNSPECIFIED.,.F.,.F.)
B_SPLINE_CURVE_WITH_KNOTS((3,3),(0.,0.0436887632258074),.UNSPECIFIED.)
CURVE()
GEOMETRIC_REPRESENTATION_ITEM()
RATIONAL_B_SPLINE_CURVE((1.,1.00100330533774,1.00083425612174))
REPRESENTATION_ITEM('')
);
#214=(
BOUNDED_CURVE()
B_SPLINE_CURVE(2,(#31286,#31287,#31288),.UNSPECIFIED.,.F.,.F.)
B_SPLINE_CURVE_WITH_KNOTS((3,3),(0.,0.0431500162549509),.UNSPECIFIED.)
CURVE()
GEOMETRIC_REPRESENTATION_ITEM()
RATIONAL_B_SPLINE_CURVE((1.,1.00122087809425,1.00126937543051))
REPRESENTATION_ITEM('')
);
#215=(
BOUNDED_CURVE()
B_SPLINE_CURVE(2,(#31291,#31292,#31293),.UNSPECIFIED.,.F.,.F.)
B_SPLINE_CURVE_WITH_KNOTS((3,3),(0.0310892451912129,0.0747780084169828),
 .UNSPECIFIED.)
CURVE()
GEOMETRIC_REPRESENTATION_ITEM()
RATIONAL_B_SPLINE_CURVE((1.00083425612163,1.00100330533761,1.))
REPRESENTATION_ITEM('')
);
#216=(
BOUNDED_CURVE()
B_SPLINE_CURVE(2,(#31297,#31298,#31299),.UNSPECIFIED.,.F.,.F.)
B_SPLINE_CURVE_WITH_KNOTS((3,3),(0.0467199500564181,0.0898699663113547),
 .UNSPECIFIED.)
CURVE()
GEOMETRIC_REPRESENTATION_ITEM()
RATIONAL_B_SPLINE_CURVE((1.00126937543066,1.0012208780944,1.))
REPRESENTATION_ITEM('')
);
#217=(
BOUNDED_CURVE()
B_SPLINE_CURVE(2,(#31303,#31304,#31305),.UNSPECIFIED.,.F.,.F.)
B_SPLINE_CURVE_WITH_KNOTS((3,3),(0.,0.0436887632258064),.UNSPECIFIED.)
CURVE()
GEOMETRIC_REPRESENTATION_ITEM()
RATIONAL_B_SPLINE_CURVE((1.,1.00100330533711,1.00083425612121))
REPRESENTATION_ITEM('')
);
#218=(
BOUNDED_CURVE()
B_SPLINE_CURVE(2,(#31309,#31310,#31311),.UNSPECIFIED.,.F.,.F.)
B_SPLINE_CURVE_WITH_KNOTS((3,3),(0.,0.0431500162549468),.UNSPECIFIED.)
CURVE()
GEOMETRIC_REPRESENTATION_ITEM()
RATIONAL_B_SPLINE_CURVE((1.,1.00122087809451,1.00126937543078))
REPRESENTATION_ITEM('')
);
#219=(
BOUNDED_CURVE()
B_SPLINE_CURVE(2,(#31314,#31315,#31316),.UNSPECIFIED.,.F.,.F.)
B_SPLINE_CURVE_WITH_KNOTS((3,3),(0.0310892451911651,0.0747780084169829),
 .UNSPECIFIED.)
CURVE()
GEOMETRIC_REPRESENTATION_ITEM()
RATIONAL_B_SPLINE_CURVE((1.00083425612205,1.00100330533812,1.))
REPRESENTATION_ITEM('')
);
#220=(
BOUNDED_CURVE()
B_SPLINE_CURVE(2,(#31320,#31321,#31322),.UNSPECIFIED.,.F.,.F.)
B_SPLINE_CURVE_WITH_KNOTS((3,3),(0.0467199500563987,0.0898699663113548),
 .UNSPECIFIED.)
CURVE()
GEOMETRIC_REPRESENTATION_ITEM()
RATIONAL_B_SPLINE_CURVE((1.00126937543082,1.00122087809454,1.))
REPRESENTATION_ITEM('')
);
#221=(
BOUNDED_CURVE()
B_SPLINE_CURVE(2,(#31326,#31327,#31328),.UNSPECIFIED.,.F.,.F.)
B_SPLINE_CURVE_WITH_KNOTS((3,3),(0.,0.0436887632257942),.UNSPECIFIED.)
CURVE()
GEOMETRIC_REPRESENTATION_ITEM()
RATIONAL_B_SPLINE_CURVE((1.,1.0010033053377,1.0008342561217))
REPRESENTATION_ITEM('')
);
#222=(
BOUNDED_CURVE()
B_SPLINE_CURVE(2,(#31332,#31333,#31334),.UNSPECIFIED.,.F.,.F.)
B_SPLINE_CURVE_WITH_KNOTS((3,3),(0.,0.0431500162549576),.UNSPECIFIED.)
CURVE()
GEOMETRIC_REPRESENTATION_ITEM()
RATIONAL_B_SPLINE_CURVE((1.,1.00122087809465,1.00126937543093))
REPRESENTATION_ITEM('')
);
#223=(
BOUNDED_CURVE()
B_SPLINE_CURVE(2,(#31337,#31338,#31339),.UNSPECIFIED.,.F.,.F.)
B_SPLINE_CURVE_WITH_KNOTS((3,3),(0.0310892451911712,0.0747780084169828),
 .UNSPECIFIED.)
CURVE()
GEOMETRIC_REPRESENTATION_ITEM()
RATIONAL_B_SPLINE_CURVE((1.00083425612158,1.00100330533755,1.))
REPRESENTATION_ITEM('')
);
#224=(
BOUNDED_CURVE()
B_SPLINE_CURVE(2,(#31343,#31344,#31345),.UNSPECIFIED.,.F.,.F.)
B_SPLINE_CURVE_WITH_KNOTS((3,3),(0.0467199500563997,0.0898699663113548),
 .UNSPECIFIED.)
CURVE()
GEOMETRIC_REPRESENTATION_ITEM()
RATIONAL_B_SPLINE_CURVE((1.00126937543088,1.0012208780946,1.))
REPRESENTATION_ITEM('')
);
#225=(
BOUNDED_CURVE()
B_SPLINE_CURVE(2,(#31349,#31350,#31351),.UNSPECIFIED.,.F.,.F.)
B_SPLINE_CURVE_WITH_KNOTS((3,3),(0.,0.0436887632257912),.UNSPECIFIED.)
CURVE()
GEOMETRIC_REPRESENTATION_ITEM()
RATIONAL_B_SPLINE_CURVE((1.,1.00100330533807,1.00083425612201))
REPRESENTATION_ITEM('')
);
#226=(
BOUNDED_CURVE()
B_SPLINE_CURVE(2,(#31355,#31356,#31357),.UNSPECIFIED.,.F.,.F.)
B_SPLINE_CURVE_WITH_KNOTS((3,3),(0.,0.0431500162549322),.UNSPECIFIED.)
CURVE()
GEOMETRIC_REPRESENTATION_ITEM()
RATIONAL_B_SPLINE_CURVE((1.,1.00122087809449,1.00126937543076))
REPRESENTATION_ITEM('')
);
#227=(
BOUNDED_CURVE()
B_SPLINE_CURVE(2,(#31360,#31361,#31362),.UNSPECIFIED.,.F.,.F.)
B_SPLINE_CURVE_WITH_KNOTS((3,3),(0.0310892451911953,0.0747780084169828),
 .UNSPECIFIED.)
CURVE()
GEOMETRIC_REPRESENTATION_ITEM()
RATIONAL_B_SPLINE_CURVE((1.0008342561224,1.00100330533854,1.))
REPRESENTATION_ITEM('')
);
#228=(
BOUNDED_CURVE()
B_SPLINE_CURVE(2,(#31366,#31367,#31368),.UNSPECIFIED.,.F.,.F.)
B_SPLINE_CURVE_WITH_KNOTS((3,3),(0.0467199500563888,0.0898699663113548),
 .UNSPECIFIED.)
CURVE()
GEOMETRIC_REPRESENTATION_ITEM()
RATIONAL_B_SPLINE_CURVE((1.0012693754306,1.00122087809433,1.))
REPRESENTATION_ITEM('')
);
#229=(
BOUNDED_CURVE()
B_SPLINE_CURVE(2,(#31372,#31373,#31374),.UNSPECIFIED.,.F.,.F.)
B_SPLINE_CURVE_WITH_KNOTS((3,3),(0.,0.0436887632258443),.UNSPECIFIED.)
CURVE()
GEOMETRIC_REPRESENTATION_ITEM()
RATIONAL_B_SPLINE_CURVE((1.,1.00100330533721,1.0008342561213))
REPRESENTATION_ITEM('')
);
#230=(
BOUNDED_CURVE()
B_SPLINE_CURVE(2,(#31378,#31379,#31380),.UNSPECIFIED.,.F.,.F.)
B_SPLINE_CURVE_WITH_KNOTS((3,3),(0.,0.0431500162549717),.UNSPECIFIED.)
CURVE()
GEOMETRIC_REPRESENTATION_ITEM()
RATIONAL_B_SPLINE_CURVE((1.,1.00122087809461,1.00126937543088))
REPRESENTATION_ITEM('')
);
#231=(
BOUNDED_CURVE()
B_SPLINE_CURVE(2,(#31383,#31384,#31385),.UNSPECIFIED.,.F.,.F.)
B_SPLINE_CURVE_WITH_KNOTS((3,3),(0.0310892451911806,0.0747780084169829),
 .UNSPECIFIED.)
CURVE()
GEOMETRIC_REPRESENTATION_ITEM()
RATIONAL_B_SPLINE_CURVE((1.00083425612159,1.00100330533756,1.))
REPRESENTATION_ITEM('')
);
#232=(
BOUNDED_CURVE()
B_SPLINE_CURVE(2,(#31389,#31390,#31391),.UNSPECIFIED.,.F.,.F.)
B_SPLINE_CURVE_WITH_KNOTS((3,3),(0.0467199500563954,0.0898699663113548),
 .UNSPECIFIED.)
CURVE()
GEOMETRIC_REPRESENTATION_ITEM()
RATIONAL_B_SPLINE_CURVE((1.00126937543089,1.00122087809461,1.))
REPRESENTATION_ITEM('')
);
#233=(
BOUNDED_CURVE()
B_SPLINE_CURVE(2,(#31395,#31396,#31397),.UNSPECIFIED.,.F.,.F.)
B_SPLINE_CURVE_WITH_KNOTS((3,3),(0.,0.0436887632258089),.UNSPECIFIED.)
CURVE()
GEOMETRIC_REPRESENTATION_ITEM()
RATIONAL_B_SPLINE_CURVE((1.,1.00100330533773,1.00083425612173))
REPRESENTATION_ITEM('')
);
#234=(
BOUNDED_CURVE()
B_SPLINE_CURVE(2,(#31401,#31402,#31403),.UNSPECIFIED.,.F.,.F.)
B_SPLINE_CURVE_WITH_KNOTS((3,3),(0.,0.0431500162549499),.UNSPECIFIED.)
CURVE()
GEOMETRIC_REPRESENTATION_ITEM()
RATIONAL_B_SPLINE_CURVE((1.,1.00122087809471,1.00126937543099))
REPRESENTATION_ITEM('')
);
#235=(
BOUNDED_CURVE()
B_SPLINE_CURVE(2,(#31406,#31407,#31408),.UNSPECIFIED.,.F.,.F.)
B_SPLINE_CURVE_WITH_KNOTS((3,3),(0.0310892451911691,0.0747780084169828),
 .UNSPECIFIED.)
CURVE()
GEOMETRIC_REPRESENTATION_ITEM()
RATIONAL_B_SPLINE_CURVE((1.0008342561213,1.00100330533722,1.))
REPRESENTATION_ITEM('')
);
#236=(
BOUNDED_CURVE()
B_SPLINE_CURVE(2,(#31412,#31413,#31414),.UNSPECIFIED.,.F.,.F.)
B_SPLINE_CURVE_WITH_KNOTS((3,3),(0.0467199500563946,0.0898699663113549),
 .UNSPECIFIED.)
CURVE()
GEOMETRIC_REPRESENTATION_ITEM()
RATIONAL_B_SPLINE_CURVE((1.00126937543091,1.00122087809463,1.))
REPRESENTATION_ITEM('')
);
#237=(
BOUNDED_CURVE()
B_SPLINE_CURVE(2,(#31418,#31419,#31420),.UNSPECIFIED.,.F.,.F.)
B_SPLINE_CURVE_WITH_KNOTS((3,3),(0.,0.0436887632258018),.UNSPECIFIED.)
CURVE()
GEOMETRIC_REPRESENTATION_ITEM()
RATIONAL_B_SPLINE_CURVE((1.,1.00100330533801,1.00083425612196))
REPRESENTATION_ITEM('')
);
#238=(
BOUNDED_CURVE()
B_SPLINE_CURVE(2,(#31424,#31425,#31426),.UNSPECIFIED.,.F.,.F.)
B_SPLINE_CURVE_WITH_KNOTS((3,3),(0.,0.0431500162549446),.UNSPECIFIED.)
CURVE()
GEOMETRIC_REPRESENTATION_ITEM()
RATIONAL_B_SPLINE_CURVE((1.,1.00122087809491,1.00126937543119))
REPRESENTATION_ITEM('')
);
#239=(
BOUNDED_CURVE()
B_SPLINE_CURVE(2,(#31429,#31430,#31431),.UNSPECIFIED.,.F.,.F.)
B_SPLINE_CURVE_WITH_KNOTS((3,3),(0.0310892451912006,0.0747780084169829),
 .UNSPECIFIED.)
CURVE()
GEOMETRIC_REPRESENTATION_ITEM()
RATIONAL_B_SPLINE_CURVE((1.00083425612167,1.00100330533765,1.))
REPRESENTATION_ITEM('')
);
#240=(
BOUNDED_CURVE()
B_SPLINE_CURVE(2,(#31435,#31436,#31437),.UNSPECIFIED.,.F.,.F.)
B_SPLINE_CURVE_WITH_KNOTS((3,3),(0.0467199500564005,0.0898699663113549),
 .UNSPECIFIED.)
CURVE()
GEOMETRIC_REPRESENTATION_ITEM()
RATIONAL_B_SPLINE_CURVE((1.00126937543091,1.00122087809463,1.))
REPRESENTATION_ITEM('')
);
#241=(
BOUNDED_CURVE()
B_SPLINE_CURVE(2,(#31441,#31442,#31443),.UNSPECIFIED.,.F.,.F.)
B_SPLINE_CURVE_WITH_KNOTS((3,3),(0.,0.0436887632257904),.UNSPECIFIED.)
CURVE()
GEOMETRIC_REPRESENTATION_ITEM()
RATIONAL_B_SPLINE_CURVE((1.,1.00100330533768,1.00083425612169))
REPRESENTATION_ITEM('')
);
#242=(
BOUNDED_CURVE()
B_SPLINE_CURVE(2,(#31447,#31448,#31449),.UNSPECIFIED.,.F.,.F.)
B_SPLINE_CURVE_WITH_KNOTS((3,3),(0.,0.0431500162549576),.UNSPECIFIED.)
CURVE()
GEOMETRIC_REPRESENTATION_ITEM()
RATIONAL_B_SPLINE_CURVE((1.,1.00122087809446,1.00126937543073))
REPRESENTATION_ITEM('')
);
#243=(
BOUNDED_CURVE()
B_SPLINE_CURVE(2,(#31452,#31453,#31454),.UNSPECIFIED.,.F.,.F.)
B_SPLINE_CURVE_WITH_KNOTS((3,3),(0.0310892451911633,0.0747780084169828),
 .UNSPECIFIED.)
CURVE()
GEOMETRIC_REPRESENTATION_ITEM()
RATIONAL_B_SPLINE_CURVE((1.00083425612268,1.00100330533887,1.))
REPRESENTATION_ITEM('')
);
#244=(
BOUNDED_CURVE()
B_SPLINE_CURVE(2,(#31458,#31459,#31460),.UNSPECIFIED.,.F.,.F.)
B_SPLINE_CURVE_WITH_KNOTS((3,3),(0.0467199500564166,0.089869966311355),
 .UNSPECIFIED.)
CURVE()
GEOMETRIC_REPRESENTATION_ITEM()
RATIONAL_B_SPLINE_CURVE((1.00126937543126,1.00122087809497,1.))
REPRESENTATION_ITEM('')
);
#245=(
BOUNDED_CURVE()
B_SPLINE_CURVE(2,(#31464,#31465,#31466),.UNSPECIFIED.,.F.,.F.)
B_SPLINE_CURVE_WITH_KNOTS((3,3),(0.,0.0436887632258151),.UNSPECIFIED.)
CURVE()
GEOMETRIC_REPRESENTATION_ITEM()
RATIONAL_B_SPLINE_CURVE((1.,1.00100330533817,1.00083425612209))
REPRESENTATION_ITEM('')
);
#246=(
BOUNDED_CURVE()
B_SPLINE_CURVE(2,(#31470,#31471,#31472),.UNSPECIFIED.,.F.,.F.)
B_SPLINE_CURVE_WITH_KNOTS((3,3),(0.,0.0431500162549457),.UNSPECIFIED.)
CURVE()
GEOMETRIC_REPRESENTATION_ITEM()
RATIONAL_B_SPLINE_CURVE((1.,1.00122087809449,1.00126937543076))
REPRESENTATION_ITEM('')
);
#247=(
BOUNDED_CURVE()
B_SPLINE_CURVE(2,(#31475,#31476,#31477),.UNSPECIFIED.,.F.,.F.)
B_SPLINE_CURVE_WITH_KNOTS((3,3),(0.0310892451911691,0.0747780084169829),
 .UNSPECIFIED.)
CURVE()
GEOMETRIC_REPRESENTATION_ITEM()
RATIONAL_B_SPLINE_CURVE((1.00083425612148,1.00100330533743,1.))
REPRESENTATION_ITEM('')
);
#248=(
BOUNDED_CURVE()
B_SPLINE_CURVE(2,(#31481,#31482,#31483),.UNSPECIFIED.,.F.,.F.)
B_SPLINE_CURVE_WITH_KNOTS((3,3),(0.0467199500564313,0.089869966311355),
 .UNSPECIFIED.)
CURVE()
GEOMETRIC_REPRESENTATION_ITEM()
RATIONAL_B_SPLINE_CURVE((1.00126937543075,1.00122087809448,1.))
REPRESENTATION_ITEM('')
);
#249=(
BOUNDED_CURVE()
B_SPLINE_CURVE(2,(#31487,#31488,#31489),.UNSPECIFIED.,.F.,.F.)
B_SPLINE_CURVE_WITH_KNOTS((3,3),(0.,0.0436887632257837),.UNSPECIFIED.)
CURVE()
GEOMETRIC_REPRESENTATION_ITEM()
RATIONAL_B_SPLINE_CURVE((1.,1.00100330533754,1.00083425612157))
REPRESENTATION_ITEM('')
);
#250=(
BOUNDED_CURVE()
B_SPLINE_CURVE(2,(#31493,#31494,#31495),.UNSPECIFIED.,.F.,.F.)
B_SPLINE_CURVE_WITH_KNOTS((3,3),(0.,0.043150016254948),.UNSPECIFIED.)
CURVE()
GEOMETRIC_REPRESENTATION_ITEM()
RATIONAL_B_SPLINE_CURVE((1.,1.00122087809439,1.00126937543066))
REPRESENTATION_ITEM('')
);
#251=(
BOUNDED_CURVE()
B_SPLINE_CURVE(2,(#31498,#31499,#31500),.UNSPECIFIED.,.F.,.F.)
B_SPLINE_CURVE_WITH_KNOTS((3,3),(0.0310892451912077,0.0747780084169828),
 .UNSPECIFIED.)
CURVE()
GEOMETRIC_REPRESENTATION_ITEM()
RATIONAL_B_SPLINE_CURVE((1.00083425612152,1.00100330533748,1.))
REPRESENTATION_ITEM('')
);
#441=SHAPE_REPRESENTATION_RELATIONSHIP('SRR','None',#38677,#455);
#455=ADVANCED_BREP_SHAPE_REPRESENTATION('',(#483),#38606);
#469=STYLED_ITEM('',(#38885),#483);
#483=MANIFOLD_SOLID_BREP('Adjuster',#16243);
#503=B_SPLINE_SURFACE_WITH_KNOTS('',3,3,((#29345,#29346,#29347,#29348,#29349,
#29350,#29351,#29352,#29353,#29354,#29355,#29356,#29357,#29358,#29359,#29360,
#29361,#29362,#29363,#29364,#29365,#29366,#29367,#29368,#29369,#29370,#29371,
#29372,#29373,#29374,#29375,#29376,#29377,#29378,#29379,#29380,#29381,#29382,
#29383,#29384,#29385,#29386,#29387,#29388,#29389,#29390,#29391,#29392,#29393,
#29394,#29395,#29396,#29397,#29398,#29399,#29400,#29401,#29402,#29403,#29404,
#29405,#29406,#29407,#29408,#29409,#29410,#29411,#29412,#29413,#29414,#29415,
#29416,#29417,#29418,#29419,#29420,#29421,#29422,#29423,#29424,#29425,#29426,
#29427,#29428,#29429,#29430,#29431,#29432,#29433,#29434,#29435,#29436,#29437,
#29438,#29439,#29440,#29441,#29442,#29443,#29444,#29445,#29446,#29447,#29448,
#29449,#29450,#29451,#29452,#29453,#29454,#29455,#29456,#29457,#29458,#29459,
#29460,#29461,#29462,#29463,#29464,#29465,#29466,#29467,#29468,#29469,#29470,
#29471,#29472,#29473,#29474,#29475,#29476,#29477,#29478,#29479,#29480,#29481,
#29482,#29483,#29484,#29485,#29486,#29487,#29488,#29489,#29490,#29491,#29492,
#29493,#29494,#29495,#29496),(#29497,#29498,#29499,#29500,#29501,#29502,
#29503,#29504,#29505,#29506,#29507,#29508,#29509,#29510,#29511,#29512,#29513,
#29514,#29515,#29516,#29517,#29518,#29519,#29520,#29521,#29522,#29523,#29524,
#29525,#29526,#29527,#29528,#29529,#29530,#29531,#29532,#29533,#29534,#29535,
#29536,#29537,#29538,#29539,#29540,#29541,#29542,#29543,#29544,#29545,#29546,
#29547,#29548,#29549,#29550,#29551,#29552,#29553,#29554,#29555,#29556,#29557,
#29558,#29559,#29560,#29561,#29562,#29563,#29564,#29565,#29566,#29567,#29568,
#29569,#29570,#29571,#29572,#29573,#29574,#29575,#29576,#29577,#29578,#29579,
#29580,#29581,#29582,#29583,#29584,#29585,#29586,#29587,#29588,#29589,#29590,
#29591,#29592,#29593,#29594,#29595,#29596,#29597,#29598,#29599,#29600,#29601,
#29602,#29603,#29604,#29605,#29606,#29607,#29608,#29609,#29610,#29611,#29612,
#29613,#29614,#29615,#29616,#29617,#29618,#29619,#29620,#29621,#29622,#29623,
#29624,#29625,#29626,#29627,#29628,#29629,#29630,#29631,#29632,#29633,#29634,
#29635,#29636,#29637,#29638,#29639,#29640,#29641,#29642,#29643,#29644,#29645,
#29646,#29647,#29648),(#29649,#29650,#29651,#29652,#29653,#29654,#29655,
#29656,#29657,#29658,#29659,#29660,#29661,#29662,#29663,#29664,#29665,#29666,
#29667,#29668,#29669,#29670,#29671,#29672,#29673,#29674,#29675,#29676,#29677,
#29678,#29679,#29680,#29681,#29682,#29683,#29684,#29685,#29686,#29687,#29688,
#29689,#29690,#29691,#29692,#29693,#29694,#29695,#29696,#29697,#29698,#29699,
#29700,#29701,#29702,#29703,#29704,#29705,#29706,#29707,#29708,#29709,#29710,
#29711,#29712,#29713,#29714,#29715,#29716,#29717,#29718,#29719,#29720,#29721,
#29722,#29723,#29724,#29725,#29726,#29727,#29728,#29729,#29730,#29731,#29732,
#29733,#29734,#29735,#29736,#29737,#29738,#29739,#29740,#29741,#29742,#29743,
#29744,#29745,#29746,#29747,#29748,#29749,#29750,#29751,#29752,#29753,#29754,
#29755,#29756,#29757,#29758,#29759,#29760,#29761,#29762,#29763,#29764,#29765,
#29766,#29767,#29768,#29769,#29770,#29771,#29772,#29773,#29774,#29775,#29776,
#29777,#29778,#29779,#29780,#29781,#29782,#29783,#29784,#29785,#29786,#29787,
#29788,#29789,#29790,#29791,#29792,#29793,#29794,#29795,#29796,#29797,#29798,
#29799,#29800),(#29801,#29802,#29803,#29804,#29805,#29806,#29807,#29808,
#29809,#29810,#29811,#29812,#29813,#29814,#29815,#29816,#29817,#29818,#29819,
#29820,#29821,#29822,#29823,#29824,#29825,#29826,#29827,#29828,#29829,#29830,
#29831,#29832,#29833,#29834,#29835,#29836,#29837,#29838,#29839,#29840,#29841,
#29842,#29843,#29844,#29845,#29846,#29847,#29848,#29849,#29850,#29851,#29852,
#29853,#29854,#29855,#29856,#29857,#29858,#29859,#29860,#29861,#29862,#29863,
#29864,#29865,#29866,#29867,#29868,#29869,#29870,#29871,#29872,#29873,#29874,
#29875,#29876,#29877,#29878,#29879,#29880,#29881,#29882,#29883,#29884,#29885,
#29886,#29887,#29888,#29889,#29890,#29891,#29892,#29893,#29894,#29895,#29896,
#29897,#29898,#29899,#29900,#29901,#29902,#29903,#29904,#29905,#29906,#29907,
#29908,#29909,#29910,#29911,#29912,#29913,#29914,#29915,#29916,#29917,#29918,
#29919,#29920,#29921,#29922,#29923,#29924,#29925,#29926,#29927,#29928,#29929,
#29930,#29931,#29932,#29933,#29934,#29935,#29936,#29937,#29938,#29939,#29940,
#29941,#29942,#29943,#29944,#29945,#29946,#29947,#29948,#29949,#29950,#29951,
#29952)),.UNSPECIFIED.,.F.,.F.,.F.,(4,4),(4,1,1,1,1,1,1,1,1,1,1,1,1,1,1,
1,1,1,1,1,1,1,1,1,1,1,1,1,1,1,1,1,1,1,1,1,1,1,1,1,1,1,1,1,1,1,1,1,1,1,1,
1,1,1,1,1,1,1,1,1,1,1,1,1,1,1,1,1,1,1,1,1,1,1,1,1,1,1,1,1,1,1,1,1,1,1,1,
1,1,1,1,1,1,1,1,1,1,1,1,1,1,1,1,1,1,1,1,1,1,1,1,1,1,1,1,1,1,1,1,1,1,1,1,
1,1,1,1,1,1,1,1,1,1,1,1,1,1,1,1,1,1,1,1,1,1,1,1,1,1,4),(0.,0.0329955678841871),
(8.30276167405409,9.29807539437161,10.2933891146891,11.2887028350066,12.2840165553242,
13.2793302756417,14.2746439959592,15.2699577162767,16.2652714365942,17.2605851569118,
18.2558988772293,19.2512125975468,20.2465263178643,21.2418400381818,22.2371537584993,
23.2324674788169,24.2277811991344,25.2230949194519,26.2184086397694,27.2137223600869,
28.2090360804045,29.204349800722,30.1996635210395,31.194977241357,32.1902909616745,
33.185604681992,34.1809184023096,35.1762321226271,36.1715458429446,37.1668595632621,
38.1621732835796,39.1574870038972,40.1528007242147,41.1481144445322,42.1434281648497,
43.1387418851672,44.1340556054847,45.1293693258023,46.1246830461198,47.1199967664373,
48.1153104867548,49.1106242070723,50.1059379273898,51.1012516477074,52.0965653680249,
53.0918790883424,54.0871928086599,55.0825065289774,56.077820249295,57.0731339696125,
58.06844768993,59.0637614102475,60.059075130565,61.0543888508825,62.0497025712001,
63.0450162915176,64.0403300118351,65.0356437321526,66.0309574524701,67.0262711727877,
68.0215848931052,69.0168986134227,70.0122123337402,71.0075260540577,72.0028397743752,
72.9981534946928,73.9934672150103,74.9887809353278,75.9840946556453,76.9794083759628,
77.9747220962804,78.9700358165979,79.9653495369154,80.9606632572329,81.9559769775504,
82.9512906978679,83.9466044181855,84.941918138503,85.9372318588205,86.932545579138,
87.9278592994555,88.9231730197731,89.9184867400906,90.9138004604081,91.9091141807256,
92.9044279010431,93.8997416213606,94.8950553416782,95.8903690619957,96.8856827823132,
97.8809965026307,98.8763102229482,99.8716239432658,100.866937663583,101.862251383901,
102.857565104218,103.852878824536,104.848192544853,105.843506265171,106.838819985488,
107.834133705806,108.829447426123,109.824761146441,110.820074866758,111.815388587076,
112.810702307393,113.806016027711,114.801329748029,115.796643468346,116.791957188664,
117.787270908981,118.782584629299,119.777898349616,120.773212069934,121.768525790251,
122.763839510569,123.759153230886,124.754466951204,125.749780671521,126.745094391839,
127.740408112156,128.735721832474,129.731035552791,130.726349273109,131.721662993426,
132.716976713744,133.712290434061,134.707604154379,135.702917874696,136.698231595014,
137.693545315331,138.688859035649,139.684172755966,140.679486476284,141.674800196602,
142.670113916919,143.665427637237,144.660741357554,145.656055077872,146.651368798189,
147.646682518507,148.641996238824,149.637309959142,150.632623679459,151.627937399777,
152.623251120094,153.618564840412,154.613878560729,155.609192281047,156.604506001364),
 .UNSPECIFIED.);
#504=B_SPLINE_SURFACE_WITH_KNOTS('',3,3,((#30148,#30149,#30150,#30151,#30152,
#30153,#30154,#30155,#30156,#30157,#30158,#30159,#30160,#30161,#30162,#30163,
#30164,#30165,#30166,#30167,#30168,#30169,#30170,#30171,#30172,#30173,#30174,
#30175,#30176,#30177,#30178,#30179,#30180,#30181,#30182,#30183,#30184,#30185,
#30186,#30187,#30188,#30189,#30190,#30191,#30192,#30193,#30194,#30195,#30196,
#30197,#30198,#30199,#30200,#30201,#30202,#30203,#30204,#30205,#30206,#30207,
#30208,#30209,#30210,#30211,#30212,#30213,#30214,#30215,#30216,#30217,#30218,
#30219,#30220,#30221,#30222,#30223,#30224,#30225,#30226,#30227,#30228,#30229,
#30230,#30231,#30232,#30233,#30234,#30235,#30236,#30237,#30238,#30239,#30240,
#30241,#30242,#30243,#30244,#30245,#30246,#30247,#30248,#30249,#30250,#30251,
#30252,#30253,#30254,#30255,#30256,#30257,#30258,#30259,#30260,#30261,#30262,
#30263,#30264,#30265,#30266,#30267,#30268,#30269,#30270,#30271,#30272,#30273,
#30274,#30275,#30276,#30277,#30278,#30279,#30280,#30281,#30282,#30283,#30284,
#30285,#30286,#30287,#30288,#30289,#30290,#30291,#30292,#30293,#30294,#30295,
#30296,#30297,#30298,#30299),(#30300,#30301,#30302,#30303,#30304,#30305,
#30306,#30307,#30308,#30309,#30310,#30311,#30312,#30313,#30314,#30315,#30316,
#30317,#30318,#30319,#30320,#30321,#30322,#30323,#30324,#30325,#30326,#30327,
#30328,#30329,#30330,#30331,#30332,#30333,#30334,#30335,#30336,#30337,#30338,
#30339,#30340,#30341,#30342,#30343,#30344,#30345,#30346,#30347,#30348,#30349,
#30350,#30351,#30352,#30353,#30354,#30355,#30356,#30357,#30358,#30359,#30360,
#30361,#30362,#30363,#30364,#30365,#30366,#30367,#30368,#30369,#30370,#30371,
#30372,#30373,#30374,#30375,#30376,#30377,#30378,#30379,#30380,#30381,#30382,
#30383,#30384,#30385,#30386,#30387,#30388,#30389,#30390,#30391,#30392,#30393,
#30394,#30395,#30396,#30397,#30398,#30399,#30400,#30401,#30402,#30403,#30404,
#30405,#30406,#30407,#30408,#30409,#30410,#30411,#30412,#30413,#30414,#30415,
#30416,#30417,#30418,#30419,#30420,#30421,#30422,#30423,#30424,#30425,#30426,
#30427,#30428,#30429,#30430,#30431,#30432,#30433,#30434,#30435,#30436,#30437,
#30438,#30439,#30440,#30441,#30442,#30443,#30444,#30445,#30446,#30447,#30448,
#30449,#30450,#30451),(#30452,#30453,#30454,#30455,#30456,#30457,#30458,
#30459,#30460,#30461,#30462,#30463,#30464,#30465,#30466,#30467,#30468,#30469,
#30470,#30471,#30472,#30473,#30474,#30475,#30476,#30477,#30478,#30479,#30480,
#30481,#30482,#30483,#30484,#30485,#30486,#30487,#30488,#30489,#30490,#30491,
#30492,#30493,#30494,#30495,#30496,#30497,#30498,#30499,#30500,#30501,#30502,
#30503,#30504,#30505,#30506,#30507,#30508,#30509,#30510,#30511,#30512,#30513,
#30514,#30515,#30516,#30517,#30518,#30519,#30520,#30521,#30522,#30523,#30524,
#30525,#30526,#30527,#30528,#30529,#30530,#30531,#30532,#30533,#30534,#30535,
#30536,#30537,#30538,#30539,#30540,#30541,#30542,#30543,#30544,#30545,#30546,
#30547,#30548,#30549,#30550,#30551,#30552,#30553,#30554,#30555,#30556,#30557,
#30558,#30559,#30560,#30561,#30562,#30563,#30564,#30565,#30566,#30567,#30568,
#30569,#30570,#30571,#30572,#30573,#30574,#30575,#30576,#30577,#30578,#30579,
#30580,#30581,#30582,#30583,#30584,#30585,#30586,#30587,#30588,#30589,#30590,
#30591,#30592,#30593,#30594,#30595,#30596,#30597,#30598,#30599,#30600,#30601,
#30602,#30603),(#30604,#30605,#30606,#30607,#30608,#30609,#30610,#30611,
#30612,#30613,#30614,#30615,#30616,#30617,#30618,#30619,#30620,#30621,#30622,
#30623,#30624,#30625,#30626,#30627,#30628,#30629,#30630,#30631,#30632,#30633,
#30634,#30635,#30636,#30637,#30638,#30639,#30640,#30641,#30642,#30643,#30644,
#30645,#30646,#30647,#30648,#30649,#30650,#30651,#30652,#30653,#30654,#30655,
#30656,#30657,#30658,#30659,#30660,#30661,#30662,#30663,#30664,#30665,#30666,
#30667,#30668,#30669,#30670,#30671,#30672,#30673,#30674,#30675,#30676,#30677,
#30678,#30679,#30680,#30681,#30682,#30683,#30684,#30685,#30686,#30687,#30688,
#30689,#30690,#30691,#30692,#30693,#30694,#30695,#30696,#30697,#30698,#30699,
#30700,#30701,#30702,#30703,#30704,#30705,#30706,#30707,#30708,#30709,#30710,
#30711,#30712,#30713,#30714,#30715,#30716,#30717,#30718,#30719,#30720,#30721,
#30722,#30723,#30724,#30725,#30726,#30727,#30728,#30729,#30730,#30731,#30732,
#30733,#30734,#30735,#30736,#30737,#30738,#30739,#30740,#30741,#30742,#30743,
#30744,#30745,#30746,#30747,#30748,#30749,#30750,#30751,#30752,#30753,#30754,
#30755)),.UNSPECIFIED.,.F.,.F.,.F.,(4,4),(4,1,1,1,1,1,1,1,1,1,1,1,1,1,1,
1,1,1,1,1,1,1,1,1,1,1,1,1,1,1,1,1,1,1,1,1,1,1,1,1,1,1,1,1,1,1,1,1,1,1,1,
1,1,1,1,1,1,1,1,1,1,1,1,1,1,1,1,1,1,1,1,1,1,1,1,1,1,1,1,1,1,1,1,1,1,1,1,
1,1,1,1,1,1,1,1,1,1,1,1,1,1,1,1,1,1,1,1,1,1,1,1,1,1,1,1,1,1,1,1,1,1,1,1,
1,1,1,1,1,1,1,1,1,1,1,1,1,1,1,1,1,1,1,1,1,1,1,1,1,1,4),(0.,0.0329955678841871),
(11.6152142277548,12.6105279480723,13.6058416683898,14.6011553887073,15.5964691090248,
16.5917828293423,17.5870965496599,18.5824102699774,19.5777239902949,20.5730377106124,
21.5683514309299,22.5636651512475,23.558978871565,24.5542925918825,25.5496063122,
26.5449200325175,27.540233752835,28.5355474731526,29.5308611934701,30.5261749137876,
31.5214886341051,32.5168023544226,33.5121160747401,34.5074297950577,35.5027435153752,
36.4980572356927,37.4933709560102,38.4886846763277,39.4839983966453,40.4793121169628,
41.4746258372803,42.4699395575978,43.4652532779153,44.4605669982328,45.4558807185504,
46.4511944388679,47.4465081591854,48.4418218795029,49.4371355998204,50.432449320138,
51.4277630404555,52.423076760773,53.4183904810905,54.413704201408,55.4090179217255,
56.4043316420431,57.3996453623606,58.3949590826781,59.3902728029956,60.3855865233131,
61.3809002436307,62.3762139639482,63.3715276842657,64.3668414045832,65.3621551249007,
66.3574688452182,67.3527825655358,68.3480962858533,69.3434100061708,70.3387237264883,
71.3340374468058,72.3293511671233,73.3246648874409,74.3199786077584,75.3152923280759,
76.3106060483934,77.3059197687109,78.3012334890285,79.296547209346,80.2918609296635,
81.287174649981,82.2824883702986,83.2778020906161,84.2731158109336,85.2684295312511,
86.2637432515686,87.2590569718861,88.2543706922037,89.2496844125212,90.2449981328387,
91.2403118531562,92.2356255734737,93.2309392937912,94.2262530141087,95.2215667344263,
96.2168804547438,97.2121941750613,98.2075078953788,99.2028216156963,100.198135336014,
101.193449056331,102.188762776649,103.184076496966,104.179390217284,105.174703937601,
106.170017657919,107.165331378236,108.160645098554,109.155958818872,110.151272539189,
111.146586259507,112.141899979824,113.137213700142,114.132527420459,115.127841140777,
116.123154861094,117.118468581412,118.113782301729,119.109096022047,120.104409742364,
121.099723462682,122.095037182999,123.090350903317,124.085664623634,125.080978343952,
126.076292064269,127.071605784587,128.066919504904,129.062233225222,130.057546945539,
131.052860665857,132.048174386174,133.043488106492,134.038801826809,135.034115547127,
136.029429267445,137.024742987762,138.02005670808,139.015370428397,140.010684148715,
141.005997869032,142.00131158935,142.996625309667,143.991939029985,144.987252750302,
145.98256647062,146.977880190937,147.973193911255,148.968507631572,149.96382135189,
150.959135072207,151.954448792525,152.949762512842,153.94507623316,154.940389953477,
155.935703673795,156.931017394112,157.92633111443,158.921644834747,159.916958555065),
 .UNSPECIFIED.);
#627=B_SPLINE_CURVE_WITH_KNOTS('',3,(#27590,#27591,#27592,#27593,#27594,
#27595,#27596,#27597,#27598,#27599),.UNSPECIFIED.,.F.,.F.,(4,3,3,4),(-4.09274904019421,
-3.98125488127007,-2.98594116095255,-2.07317267331972),.UNSPECIFIED.);
#628=B_SPLINE_CURVE_WITH_KNOTS('',3,(#27602,#27603,#27604,#27605,#27606,
#27607,#27608),.UNSPECIFIED.,.F.,.F.,(4,3,4),(0.,0.995313720317508,1.12201628671524),
 .UNSPECIFIED.);
#629=B_SPLINE_CURVE_WITH_KNOTS('',3,(#27613,#27614,#27615,#27616,#27617,
#27618,#27619,#27620,#27621,#27622,#27623,#27624,#27625,#27626,#27627,#27628,
#27629,#27630,#27631,#27632,#27633,#27634),.UNSPECIFIED.,.F.,.F.,(4,3,3,
3,3,3,3,4),(-10.3759343473738,-9.95313720317518,-8.95782348285766,-7.96250976254015,
-6.96719604222263,-5.97188232190511,-4.9765686015876,-4.09274904019421),
 .UNSPECIFIED.);
#630=B_SPLINE_CURVE_WITH_KNOTS('',3,(#27635,#27636,#27637,#27638,#27639,
#27640,#27641,#27642,#27643,#27644,#27645,#27646,#27647,#27648,#27649,#27650,
#27651,#27652,#27653,#27654,#27655,#27656),.UNSPECIFIED.,.F.,.F.,(4,3,3,
3,3,3,3,4),(1.12201628671524,1.99062744063502,2.98594116095254,3.98125488127006,
4.97656860158758,5.9718823219051,6.96719604222262,7.40520159389483),
 .UNSPECIFIED.);
#631=B_SPLINE_CURVE_WITH_KNOTS('',3,(#27661,#27662,#27663,#27664,#27665,
#27666,#27667,#27668,#27669,#27670,#27671,#27672,#27673,#27674,#27675,#27676,
#27677,#27678,#27679,#27680,#27681,#27682),.UNSPECIFIED.,.F.,.F.,(4,3,3,
3,3,3,3,4),(-16.6591196545534,-15.9250195250803,-14.9297058047628,-13.9343920844453,
-12.9390783641277,-11.9437646438102,-10.9484509234927,-10.3759343473738),
 .UNSPECIFIED.);
#632=B_SPLINE_CURVE_WITH_KNOTS('',3,(#27683,#27684,#27685,#27686,#27687,
#27688,#27689,#27690,#27691,#27692,#27693,#27694,#27695,#27696,#27697,#27698,
#27699,#27700,#27701,#27702,#27703,#27704),.UNSPECIFIED.,.F.,.F.,(4,3,3,
3,3,3,3,4),(7.40520159389483,7.96250976254014,8.95782348285766,9.95313720317518,
10.9484509234927,11.9437646438102,12.9390783641277,13.6883869010744),
 .UNSPECIFIED.);
#633=B_SPLINE_CURVE_WITH_KNOTS('',3,(#27709,#27710,#27711,#27712,#27713,
#27714,#27715,#27716,#27717,#27718,#27719,#27720,#27721,#27722,#27723,#27724,
#27725,#27726,#27727,#27728,#27729,#27730,#27731,#27732,#27733),
 .UNSPECIFIED.,.F.,.F.,(4,3,3,3,3,3,3,3,4),(-22.942304961733,-22.8922155673029,
-21.8969018469854,-20.9015881266679,-19.9062744063504,-18.9109606860328,
-17.9156469657153,-16.9203332453978,-16.6591196545534),.UNSPECIFIED.);
#634=B_SPLINE_CURVE_WITH_KNOTS('',3,(#27734,#27735,#27736,#27737,#27738,
#27739,#27740,#27741,#27742,#27743,#27744,#27745,#27746,#27747,#27748,#27749,
#27750,#27751,#27752,#27753,#27754,#27755,#27756,#27757,#27758),
 .UNSPECIFIED.,.F.,.F.,(4,3,3,3,3,3,3,3,4),(13.6883869010744,13.9343920844453,
14.9297058047628,15.9250195250803,16.9203332453978,17.9156469657153,18.9109606860329,
19.9062744063504,19.971572208254),.UNSPECIFIED.);
#635=B_SPLINE_CURVE_WITH_KNOTS('',3,(#27763,#27764,#27765,#27766,#27767,
#27768,#27769,#27770,#27771,#27772,#27773,#27774,#27775,#27776,#27777,#27778,
#27779,#27780,#27781,#27782,#27783,#27784),.UNSPECIFIED.,.F.,.F.,(4,3,3,
3,3,3,3,4),(-29.2254902689126,-28.864097889208,-27.8687841688905,-26.873470448573,
-25.8781567282555,-24.882843007938,-23.8875292876204,-22.942304961733),
 .UNSPECIFIED.);
#636=B_SPLINE_CURVE_WITH_KNOTS('',3,(#27785,#27786,#27787,#27788,#27789,
#27790,#27791,#27792,#27793,#27794,#27795,#27796,#27797,#27798,#27799,#27800,
#27801,#27802,#27803,#27804,#27805,#27806),.UNSPECIFIED.,.F.,.F.,(4,3,3,
3,3,3,3,4),(19.971572208254,20.9015881266679,21.8969018469854,22.8922155673029,
23.8875292876204,24.882843007938,25.8781567282555,26.2547575154336),
 .UNSPECIFIED.);
#637=B_SPLINE_CURVE_WITH_KNOTS('',3,(#27811,#27812,#27813,#27814,#27815,
#27816,#27817,#27818,#27819,#27820,#27821,#27822,#27823,#27824,#27825,#27826,
#27827,#27828,#27829,#27830,#27831,#27832),.UNSPECIFIED.,.F.,.F.,(4,3,3,
3,3,3,3,4),(-35.5086755760921,-34.8359802111131,-33.8406664907956,-32.8453527704781,
-31.8500390501606,-30.8547253298431,-29.8594116095255,-29.2254902689126),
 .UNSPECIFIED.);
#638=B_SPLINE_CURVE_WITH_KNOTS('',3,(#27833,#27834,#27835,#27836,#27837,
#27838,#27839,#27840,#27841,#27842,#27843,#27844,#27845,#27846,#27847,#27848,
#27849,#27850,#27851,#27852,#27853,#27854),.UNSPECIFIED.,.F.,.F.,(4,3,3,
3,3,3,3,4),(26.2547575154336,26.873470448573,27.8687841688905,28.864097889208,
29.8594116095256,30.8547253298431,31.8500390501606,32.5379428226132),
 .UNSPECIFIED.);
#639=B_SPLINE_CURVE_WITH_KNOTS('',3,(#27859,#27860,#27861,#27862,#27863,
#27864,#27865,#27866,#27867,#27868,#27869,#27870,#27871,#27872,#27873,#27874,
#27875,#27876,#27877,#27878,#27879,#27880),.UNSPECIFIED.,.F.,.F.,(4,3,3,
3,3,3,3,4),(-41.7918608832717,-40.8078625330182,-39.8125488127007,-38.8172350923832,
-37.8219213720657,-36.8266076517482,-35.8312939314307,-35.5086755760921),
 .UNSPECIFIED.);
#640=B_SPLINE_CURVE_WITH_KNOTS('',3,(#27881,#27882,#27883,#27884,#27885,
#27886,#27887,#27888,#27889,#27890,#27891,#27892,#27893,#27894,#27895,#27896,
#27897,#27898,#27899,#27900,#27901,#27902),.UNSPECIFIED.,.F.,.F.,(4,3,3,
3,3,3,3,4),(32.5379428226132,32.8453527704781,33.8406664907956,34.8359802111131,
35.8312939314307,36.8266076517482,37.8219213720657,38.8211281297928),
 .UNSPECIFIED.);
#641=B_SPLINE_CURVE_WITH_KNOTS('',3,(#27907,#27908,#27909,#27910,#27911,
#27912,#27913,#27914,#27915,#27916,#27917,#27918,#27919,#27920,#27921,#27922,
#27923,#27924,#27925,#27926,#27927,#27928,#27929,#27930,#27931),
 .UNSPECIFIED.,.F.,.F.,(4,3,3,3,3,3,3,3,4),(-48.0750461904513,-47.7750585752409,
-46.7797448549234,-45.7844311346058,-44.7891174142883,-43.7938036939708,
-42.7984899736533,-41.8031762533358,-41.7918608832717),.UNSPECIFIED.);
#642=B_SPLINE_CURVE_WITH_KNOTS('',3,(#27932,#27933,#27934,#27935,#27936,
#27937,#27938,#27939,#27940,#27941,#27942,#27943,#27944,#27945,#27946,#27947,
#27948,#27949,#27950,#27951,#27952,#27953),.UNSPECIFIED.,.F.,.F.,(4,3,3,
3,3,3,3,4),(38.8211281297928,39.8125488127007,40.8078625330182,41.8031762533358,
42.7984899736533,43.7938036939708,44.7891174142883,45.1043134369724),
 .UNSPECIFIED.);
#643=B_SPLINE_CURVE_WITH_KNOTS('',3,(#27958,#27959,#27960,#27961,#27962,
#27963,#27964,#27965,#27966,#27967,#27968,#27969,#27970,#27971,#27972,#27973,
#27974,#27975,#27976,#27977,#27978,#27979),.UNSPECIFIED.,.F.,.F.,(4,3,3,
3,3,3,3,4),(-54.3582314976309,-53.746940897146,-52.7516271768285,-51.7563134565109,
-50.7609997361934,-49.7656860158759,-48.7703722955584,-48.0750461904513),
 .UNSPECIFIED.);
#644=B_SPLINE_CURVE_WITH_KNOTS('',3,(#27980,#27981,#27982,#27983,#27984,
#27985,#27986,#27987,#27988,#27989,#27990,#27991,#27992,#27993,#27994,#27995,
#27996,#27997,#27998,#27999,#28000,#28001),.UNSPECIFIED.,.F.,.F.,(4,3,3,
3,3,3,3,4),(45.1043134369724,45.7844311346058,46.7797448549234,47.7750585752409,
48.7703722955584,49.7656860158759,50.7609997361934,51.3874987441519),
 .UNSPECIFIED.);
#645=B_SPLINE_CURVE_WITH_KNOTS('',3,(#28006,#28007,#28008,#28009,#28010,
#28011,#28012,#28013,#28014,#28015,#28016,#28017,#28018,#28019,#28020,#28021,
#28022,#28023,#28024,#28025,#28026,#28027),.UNSPECIFIED.,.F.,.F.,(4,3,3,
3,3,3,3,4),(-60.6414168048105,-59.7188232190511,-58.7235094987336,-57.7281957784161,
-56.7328820580985,-55.737568337781,-54.7422546174635,-54.3582314976309),
 .UNSPECIFIED.);
#646=B_SPLINE_CURVE_WITH_KNOTS('',3,(#28028,#28029,#28030,#28031,#28032,
#28033,#28034,#28035,#28036,#28037,#28038,#28039,#28040,#28041,#28042,#28043,
#28044,#28045,#28046,#28047,#28048,#28049),.UNSPECIFIED.,.F.,.F.,(4,3,3,
3,3,3,3,4),(51.3874987441519,51.7563134565109,52.7516271768285,53.746940897146,
54.7422546174635,55.737568337781,56.7328820580986,57.6706840513315),
 .UNSPECIFIED.);
#647=B_SPLINE_CURVE_WITH_KNOTS('',3,(#28054,#28055,#28056,#28057,#28058,
#28059,#28060,#28061,#28062,#28063,#28064,#28065,#28066,#28067,#28068,#28069,
#28070,#28071,#28072,#28073,#28074,#28075,#28076,#28077,#28078),
 .UNSPECIFIED.,.F.,.F.,(4,3,3,3,3,3,3,3,4),(-66.9246021119901,-66.6860192612737,
-65.6907055409562,-64.6953918206387,-63.7000781003212,-62.7047643800036,
-61.7094506596861,-60.7141369393686,-60.6414168048105),.UNSPECIFIED.);
#648=B_SPLINE_CURVE_WITH_KNOTS('',3,(#28079,#28080,#28081,#28082,#28083,
#28084,#28085,#28086,#28087,#28088,#28089,#28090,#28091,#28092,#28093,#28094,
#28095,#28096,#28097,#28098,#28099,#28100,#28101,#28102,#28103),
 .UNSPECIFIED.,.F.,.F.,(4,3,3,3,3,3,3,3,4),(57.6706840513315,57.7281957784161,
58.7235094987336,59.7188232190511,60.7141369393686,61.7094506596861,62.7047643800037,
63.7000781003212,63.9538693585111),.UNSPECIFIED.);
#649=B_SPLINE_CURVE_WITH_KNOTS('',3,(#28108,#28109,#28110,#28111,#28112,
#28113,#28114,#28115,#28116,#28117,#28118,#28119,#28120,#28121,#28122,#28123,
#28124,#28125,#28126,#28127,#28128,#28129),.UNSPECIFIED.,.F.,.F.,(4,3,3,
3,3,3,3,4),(-73.2077874191697,-72.6579015831788,-71.6625878628613,-70.6672741425438,
-69.6719604222263,-68.6766467019087,-67.6813329815912,-66.9246021119901),
 .UNSPECIFIED.);
#650=B_SPLINE_CURVE_WITH_KNOTS('',3,(#28130,#28131,#28132,#28133,#28134,
#28135,#28136,#28137,#28138,#28139,#28140,#28141,#28142,#28143,#28144,#28145,
#28146,#28147,#28148,#28149,#28150,#28151),.UNSPECIFIED.,.F.,.F.,(4,3,3,
3,3,3,3,4),(63.9538693585111,64.6953918206387,65.6907055409562,66.6860192612737,
67.6813329815912,68.6766467019088,69.6719604222263,70.2370546656907),
 .UNSPECIFIED.);
#651=B_SPLINE_CURVE_WITH_KNOTS('',3,(#28156,#28157,#28158,#28159,#28160,
#28161,#28162,#28163,#28164,#28165,#28166,#28167,#28168,#28169,#28170,#28171,
#28172,#28173,#28174,#28175,#28176,#28177),.UNSPECIFIED.,.F.,.F.,(4,3,3,
3,3,3,3,4),(-79.4909727263493,-78.6297839050839,-77.6344701847664,-76.6391564644489,
-75.6438427441314,-74.6485290238139,-73.6532153034963,-73.2077874191697),
 .UNSPECIFIED.);
#652=B_SPLINE_CURVE_WITH_KNOTS('',3,(#28178,#28179,#28180,#28181,#28182,
#28183,#28184,#28185,#28186,#28187,#28188,#28189,#28190,#28191,#28192,#28193,
#28194,#28195,#28196,#28197,#28198,#28199),.UNSPECIFIED.,.F.,.F.,(4,3,3,
3,3,3,3,4),(70.2370546656907,70.6672741425438,71.6625878628613,72.6579015831788,
73.6532153034963,74.6485290238139,75.6438427441314,76.5202399728703),
 .UNSPECIFIED.);
#653=B_SPLINE_CURVE_WITH_KNOTS('',3,(#28204,#28205,#28206,#28207,#28208,
#28209,#28210,#28211,#28212,#28213,#28214,#28215,#28216,#28217,#28218,#28219,
#28220,#28221,#28222,#28223,#28224,#28225,#28226,#28227,#28228),
 .UNSPECIFIED.,.F.,.F.,(4,3,3,3,3,3,3,3,4),(-85.7741580335289,-85.5969799473066,
-84.601666226989,-83.6063525066715,-82.611038786354,-81.6157250660365,-80.620411345719,
-79.6250976254015,-79.4909727263493),.UNSPECIFIED.);
#654=B_SPLINE_CURVE_WITH_KNOTS('',3,(#28229,#28230,#28231,#28232,#28233,
#28234,#28235,#28236,#28237,#28238,#28239,#28240,#28241,#28242,#28243,#28244,
#28245,#28246,#28247,#28248,#28249,#28250,#28251,#28252,#28253),
 .UNSPECIFIED.,.F.,.F.,(4,3,3,3,3,3,3,3,4),(76.5202399728703,76.6391564644489,
77.6344701847664,78.6297839050839,79.6250976254015,80.620411345719,81.6157250660365,
82.611038786354,82.8034252800499),.UNSPECIFIED.);
#655=B_SPLINE_CURVE_WITH_KNOTS('',3,(#28258,#28259,#28260,#28261,#28262,
#28263,#28264,#28265,#28266,#28267,#28268,#28269,#28270,#28271,#28272,#28273,
#28274,#28275,#28276,#28277,#28278,#28279),.UNSPECIFIED.,.F.,.F.,(4,3,3,
3,3,3,3,4),(-92.0573433407085,-91.5688622692116,-90.5735485488942,-89.5782348285766,
-88.5829211082591,-87.5876073879416,-86.5922936676241,-85.7741580335289),
 .UNSPECIFIED.);
#656=B_SPLINE_CURVE_WITH_KNOTS('',3,(#28280,#28281,#28282,#28283,#28284,
#28285,#28286,#28287,#28288,#28289,#28290,#28291,#28292,#28293,#28294,#28295,
#28296,#28297,#28298,#28299,#28300,#28301),.UNSPECIFIED.,.F.,.F.,(4,3,3,
3,3,3,3,4),(82.8034252800499,83.6063525066715,84.6016662269891,85.5969799473066,
86.5922936676241,87.5876073879416,88.5829211082591,89.0866105872295),
 .UNSPECIFIED.);
#657=B_SPLINE_CURVE_WITH_KNOTS('',3,(#28306,#28307,#28308,#28309,#28310,
#28311,#28312,#28313,#28314,#28315,#28316,#28317,#28318,#28319,#28320,#28321,
#28322,#28323,#28324,#28325,#28326,#28327),.UNSPECIFIED.,.F.,.F.,(4,3,3,
3,3,3,3,4),(-98.3405286478881,-97.5407445911168,-96.5454308707993,-95.5501171504817,
-94.5548034301642,-93.5594897098467,-92.5641759895292,-92.0573433407085),
 .UNSPECIFIED.);
#658=B_SPLINE_CURVE_WITH_KNOTS('',3,(#28328,#28329,#28330,#28331,#28332,
#28333,#28334,#28335,#28336,#28337,#28338,#28339,#28340,#28341,#28342,#28343,
#28344,#28345,#28346,#28347,#28348,#28349),.UNSPECIFIED.,.F.,.F.,(4,3,3,
3,3,3,3,4),(89.0866105872295,89.5782348285766,90.5735485488942,91.5688622692117,
92.5641759895292,93.5594897098467,94.5548034301642,95.3697958944091),
 .UNSPECIFIED.);
#659=B_SPLINE_CURVE_WITH_KNOTS('',3,(#28354,#28355,#28356,#28357,#28358,
#28359,#28360,#28361,#28362,#28363,#28364,#28365,#28366,#28367,#28368,#28369,
#28370,#28371,#28372,#28373,#28374,#28375,#28376,#28377,#28378),
 .UNSPECIFIED.,.F.,.F.,(4,3,3,3,3,3,3,3,4),(-104.623713955068,-104.507940633339,
-103.512626913022,-102.517313192704,-101.521999472387,-100.526685752069,
-99.5313720317518,-98.5360583114343,-98.3405286478881),.UNSPECIFIED.);
#660=B_SPLINE_CURVE_WITH_KNOTS('',3,(#28379,#28380,#28381,#28382,#28383,
#28384,#28385,#28386,#28387,#28388,#28389,#28390,#28391,#28392,#28393,#28394,
#28395,#28396,#28397,#28398,#28399,#28400,#28401,#28402,#28403),
 .UNSPECIFIED.,.F.,.F.,(4,3,3,3,3,3,3,3,4),(95.3697958944091,95.5501171504818,
96.5454308707993,97.5407445911168,98.5360583114343,99.5313720317518,100.526685752069,
101.521999472387,101.652981201589),.UNSPECIFIED.);
#661=B_SPLINE_CURVE_WITH_KNOTS('',3,(#28408,#28409,#28410,#28411,#28412,
#28413,#28414,#28415,#28416,#28417,#28418,#28419,#28420,#28421,#28422,#28423,
#28424,#28425,#28426,#28427,#28428,#28429),.UNSPECIFIED.,.F.,.F.,(4,3,3,
3,3,3,3,4),(-110.906899262247,-110.479822955245,-109.484509234927,-108.489195514609,
-107.493881794292,-106.498568073974,-105.503254353657,-104.623713955068),
 .UNSPECIFIED.);
#662=B_SPLINE_CURVE_WITH_KNOTS('',3,(#28430,#28431,#28432,#28433,#28434,
#28435,#28436,#28437,#28438,#28439,#28440,#28441,#28442,#28443,#28444,#28445,
#28446,#28447,#28448,#28449,#28450,#28451),.UNSPECIFIED.,.F.,.F.,(4,3,3,
3,3,3,3,4),(101.652981201589,102.517313192704,103.512626913022,104.507940633339,
105.503254353657,106.498568073974,107.493881794292,107.936166508768),
 .UNSPECIFIED.);
#663=B_SPLINE_CURVE_WITH_KNOTS('',3,(#28456,#28457,#28458,#28459,#28460,
#28461,#28462,#28463,#28464,#28465,#28466,#28467,#28468,#28469,#28470,#28471,
#28472,#28473,#28474,#28475,#28476,#28477),.UNSPECIFIED.,.F.,.F.,(4,3,3,
3,3,3,3,4),(-117.190084569427,-116.45170527715,-115.456391556832,-114.461077836515,
-113.465764116197,-112.47045039588,-111.475136675562,-110.906899262247),
 .UNSPECIFIED.);
#664=B_SPLINE_CURVE_WITH_KNOTS('',3,(#28478,#28479,#28480,#28481,#28482,
#28483,#28484,#28485,#28486,#28487,#28488,#28489,#28490,#28491,#28492,#28493,
#28494,#28495,#28496,#28497,#28498,#28499),.UNSPECIFIED.,.F.,.F.,(4,3,3,
3,3,3,3,4),(107.936166508768,108.48919551461,109.484509234927,110.479822955245,
111.475136675562,112.47045039588,113.465764116197,114.219351815948),
 .UNSPECIFIED.);
#665=B_SPLINE_CURVE_WITH_KNOTS('',3,(#28504,#28505,#28506,#28507,#28508,
#28509,#28510,#28511,#28512,#28513,#28514,#28515,#28516,#28517,#28518,#28519,
#28520,#28521,#28522,#28523,#28524,#28525,#28526,#28527,#28528),
 .UNSPECIFIED.,.F.,.F.,(4,3,3,3,3,3,3,3,4),(-123.473269876606,-123.418901319372,
-122.423587599055,-121.428273878737,-120.43296015842,-119.437646438102,
-118.442332717785,-117.447018997467,-117.190084569427),.UNSPECIFIED.);
#666=B_SPLINE_CURVE_WITH_KNOTS('',3,(#28529,#28530,#28531,#28532,#28533,
#28534,#28535,#28536,#28537,#28538,#28539,#28540,#28541,#28542,#28543,#28544,
#28545,#28546,#28547,#28548,#28549,#28550,#28551,#28552,#28553),
 .UNSPECIFIED.,.F.,.F.,(4,3,3,3,3,3,3,3,4),(114.219351815948,114.461077836515,
115.456391556832,116.45170527715,117.447018997467,118.442332717785,119.437646438102,
120.43296015842,120.502537123127),.UNSPECIFIED.);
#667=B_SPLINE_CURVE_WITH_KNOTS('',3,(#28558,#28559,#28560,#28561,#28562,
#28563,#28564,#28565,#28566,#28567,#28568,#28569,#28570,#28571,#28572,#28573,
#28574,#28575,#28576,#28577,#28578,#28579),.UNSPECIFIED.,.F.,.F.,(4,3,3,
3,3,3,3,4),(-129.756455183786,-129.390783641277,-128.39546992096,-127.400156200642,
-126.404842480325,-125.409528760007,-124.41421503969,-123.473269876606),
 .UNSPECIFIED.);
#668=B_SPLINE_CURVE_WITH_KNOTS('',3,(#28580,#28581,#28582,#28583,#28584,
#28585,#28586,#28587,#28588,#28589,#28590,#28591,#28592,#28593,#28594,#28595,
#28596,#28597,#28598,#28599,#28600,#28601),.UNSPECIFIED.,.F.,.F.,(4,3,3,
3,3,3,3,4),(120.502537123127,121.428273878737,122.423587599055,123.418901319372,
124.41421503969,125.409528760007,126.404842480325,126.785722430307),
 .UNSPECIFIED.);
#669=B_SPLINE_CURVE_WITH_KNOTS('',3,(#28606,#28607,#28608,#28609,#28610,
#28611,#28612,#28613,#28614,#28615,#28616,#28617,#28618,#28619,#28620,#28621,
#28622,#28623,#28624,#28625,#28626,#28627),.UNSPECIFIED.,.F.,.F.,(4,3,3,
3,3,3,3,4),(-136.039640490966,-135.362665963182,-134.367352242865,-133.372038522547,
-132.37672480223,-131.381411081912,-130.386097361595,-129.756455183786),
 .UNSPECIFIED.);
#670=B_SPLINE_CURVE_WITH_KNOTS('',3,(#28628,#28629,#28630,#28631,#28632,
#28633,#28634,#28635,#28636,#28637,#28638,#28639,#28640,#28641,#28642,#28643,
#28644,#28645,#28646,#28647,#28648,#28649),.UNSPECIFIED.,.F.,.F.,(4,3,3,
3,3,3,3,4),(126.785722430307,127.400156200642,128.39546992096,129.390783641277,
130.386097361595,131.381411081912,132.37672480223,133.068907737487),
 .UNSPECIFIED.);
#671=B_SPLINE_CURVE_WITH_KNOTS('',3,(#28654,#28655,#28656,#28657,#28658,
#28659,#28660,#28661,#28662,#28663,#28664,#28665,#28666,#28667,#28668,#28669,
#28670,#28671,#28672,#28673,#28674,#28675),.UNSPECIFIED.,.F.,.F.,(4,3,3,
3,3,3,3,4),(-142.322825798145,-141.334548285088,-140.33923456477,-139.343920844453,
-138.348607124135,-137.353293403818,-136.3579796835,-136.039640490966),
 .UNSPECIFIED.);
#672=B_SPLINE_CURVE_WITH_KNOTS('',3,(#28676,#28677,#28678,#28679,#28680,
#28681,#28682,#28683,#28684,#28685,#28686,#28687,#28688,#28689,#28690,#28691,
#28692,#28693,#28694,#28695,#28696,#28697,#28698,#28699,#28700),
 .UNSPECIFIED.,.F.,.F.,(4,3,3,3,3,3,3,3,4),(133.068907737487,133.372038522547,
134.367352242865,135.362665963182,136.3579796835,137.353293403818,138.348607124135,
139.343920844453,139.352093044666),.UNSPECIFIED.);
#673=B_SPLINE_CURVE_WITH_KNOTS('',3,(#28707,#28708,#28709,#28710,#28711,
#28712,#28713,#28714,#28715,#28716,#28717,#28718,#28719,#28720,#28721,#28722,
#28723,#28724,#28725,#28726,#28727,#28728),.UNSPECIFIED.,.F.,.F.,(4,3,3,
3,3,3,3,4),(-148.30174432731,-147.306430606993,-146.311116886675,-145.315803166358,
-144.32048944604,-143.325175725723,-142.329862005405,-142.322825798145),
 .UNSPECIFIED.);
#674=B_SPLINE_CURVE_WITH_KNOTS('',3,(#28729,#28730,#28731,#28732,#28733,
#28734,#28735,#28736,#28737,#28738,#28739,#28740,#28741,#28742,#28743,#28744,
#28745,#28746,#28747,#28748,#28749,#28750),.UNSPECIFIED.,.F.,.F.,(4,3,3,
3,3,3,3,4),(139.352093044666,140.33923456477,141.334548285088,142.329862005405,
143.325175725723,144.32048944604,145.315803166358,145.635278351846),
 .UNSPECIFIED.);
#675=B_SPLINE_CURVE_WITH_KNOTS('',3,(#28756,#28757,#28758,#28759,#28760,
#28761,#28762,#28763),.UNSPECIFIED.,.F.,.F.,(4,1,1,1,1,4),(153.9380400259,
153.94507623316,154.940389953477,155.935703673795,156.931017394112,157.843785881745),
 .UNSPECIFIED.);
#676=B_SPLINE_CURVE_WITH_KNOTS('',3,(#28766,#28767,#28768,#28769,#28770,
#28771),.UNSPECIFIED.,.F.,.F.,(4,1,1,4),(153.9380400259,154.613878560729,
155.609192281047,156.604506001364),.UNSPECIFIED.);
#677=B_SPLINE_CURVE_WITH_KNOTS('',3,(#28776,#28777,#28778,#28779,#28780,
#28781,#28782,#28783,#28784,#28785),.UNSPECIFIED.,.F.,.F.,(4,1,1,1,1,1,
1,4),(147.65485471872,147.973193911255,148.968507631572,149.96382135189,
150.959135072207,151.954448792525,152.949762512842,153.9380400259),
 .UNSPECIFIED.);
#678=B_SPLINE_CURVE_WITH_KNOTS('',3,(#28786,#28787,#28788,#28789,#28790,
#28791,#28792,#28793,#28794,#28795),.UNSPECIFIED.,.F.,.F.,(4,1,1,1,1,1,
1,4),(147.65485471872,148.641996238824,149.637309959142,150.632623679459,
151.627937399777,152.623251120094,153.618564840412,153.9380400259),
 .UNSPECIFIED.);
#679=B_SPLINE_CURVE_WITH_KNOTS('',3,(#28800,#28801,#28802,#28803,#28804,
#28805,#28806,#28807,#28808,#28809),.UNSPECIFIED.,.F.,.F.,(4,1,1,1,1,1,
1,4),(141.371669411541,142.00131158935,142.996625309667,143.991939029985,
144.987252750302,145.98256647062,146.977880190937,147.65485471872),
 .UNSPECIFIED.);
#680=B_SPLINE_CURVE_WITH_KNOTS('',3,(#28810,#28811,#28812,#28813,#28814,
#28815,#28816,#28817,#28818,#28819,#28820),.UNSPECIFIED.,.F.,.F.,(4,1,1,
1,1,1,1,1,4),(141.371669411541,141.674800196602,142.670113916919,143.665427637237,
144.660741357554,145.656055077872,146.651368798189,147.646682518507,147.65485471872),
 .UNSPECIFIED.);
#681=B_SPLINE_CURVE_WITH_KNOTS('',3,(#28825,#28826,#28827,#28828,#28829,
#28830,#28831,#28832,#28833,#28834),.UNSPECIFIED.,.F.,.F.,(4,1,1,1,1,1,
1,4),(135.088484104361,136.029429267445,137.024742987762,138.02005670808,
139.015370428397,140.010684148715,141.005997869032,141.371669411541),
 .UNSPECIFIED.);
#682=B_SPLINE_CURVE_WITH_KNOTS('',3,(#28835,#28836,#28837,#28838,#28839,
#28840,#28841,#28842,#28843,#28844),.UNSPECIFIED.,.F.,.F.,(4,1,1,1,1,1,
1,4),(135.088484104361,135.702917874696,136.698231595014,137.693545315331,
138.688859035649,139.684172755966,140.679486476284,141.371669411541),
 .UNSPECIFIED.);
#683=B_SPLINE_CURVE_WITH_KNOTS('',3,(#28849,#28850,#28851,#28852,#28853,
#28854,#28855,#28856,#28857,#28858,#28859),.UNSPECIFIED.,.F.,.F.,(4,1,1,
1,1,1,1,1,4),(128.805298797182,129.062233225222,130.057546945539,131.052860665857,
132.048174386174,133.043488106492,134.038801826809,135.034115547127,135.088484104361),
 .UNSPECIFIED.);
#684=B_SPLINE_CURVE_WITH_KNOTS('',3,(#28860,#28861,#28862,#28863,#28864,
#28865,#28866,#28867,#28868,#28869),.UNSPECIFIED.,.F.,.F.,(4,1,1,1,1,1,
1,4),(128.805298797182,129.731035552791,130.726349273109,131.721662993426,
132.716976713744,133.712290434061,134.707604154379,135.088484104361),
 .UNSPECIFIED.);
#685=B_SPLINE_CURVE_WITH_KNOTS('',3,(#28874,#28875,#28876,#28877,#28878,
#28879,#28880,#28881,#28882,#28883),.UNSPECIFIED.,.F.,.F.,(4,1,1,1,1,1,
1,4),(122.522113490002,123.090350903317,124.085664623634,125.080978343952,
126.076292064269,127.071605784587,128.066919504904,128.805298797182),
 .UNSPECIFIED.);
#686=B_SPLINE_CURVE_WITH_KNOTS('',3,(#28884,#28885,#28886,#28887,#28888,
#28889,#28890,#28891,#28892,#28893,#28894),.UNSPECIFIED.,.F.,.F.,(4,1,1,
1,1,1,1,1,4),(122.522113490002,122.763839510569,123.759153230886,124.754466951204,
125.749780671521,126.745094391839,127.740408112156,128.735721832474,128.805298797182),
 .UNSPECIFIED.);
#687=B_SPLINE_CURVE_WITH_KNOTS('',3,(#28899,#28900,#28901,#28902,#28903,
#28904,#28905,#28906,#28907,#28908),.UNSPECIFIED.,.F.,.F.,(4,1,1,1,1,1,
1,4),(116.238928182822,117.118468581412,118.113782301729,119.109096022047,
120.104409742364,121.099723462682,122.095037182999,122.522113490002),
 .UNSPECIFIED.);
#688=B_SPLINE_CURVE_WITH_KNOTS('',3,(#28909,#28910,#28911,#28912,#28913,
#28914,#28915,#28916,#28917,#28918),.UNSPECIFIED.,.F.,.F.,(4,1,1,1,1,1,
1,4),(116.238928182822,116.791957188664,117.787270908981,118.782584629299,
119.777898349616,120.773212069934,121.768525790251,122.522113490002),
 .UNSPECIFIED.);
#689=B_SPLINE_CURVE_WITH_KNOTS('',3,(#28923,#28924,#28925,#28926,#28927,
#28928,#28929,#28930,#28931,#28932,#28933),.UNSPECIFIED.,.F.,.F.,(4,1,1,
1,1,1,1,1,4),(109.955742875643,110.151272539189,111.146586259507,112.141899979824,
113.137213700142,114.132527420459,115.127841140777,116.123154861094,116.238928182822),
 .UNSPECIFIED.);
#690=B_SPLINE_CURVE_WITH_KNOTS('',3,(#28934,#28935,#28936,#28937,#28938,
#28939,#28940,#28941,#28942,#28943),.UNSPECIFIED.,.F.,.F.,(4,1,1,1,1,1,
1,4),(109.955742875643,110.820074866758,111.815388587076,112.810702307393,
113.806016027711,114.801329748029,115.796643468346,116.238928182822),
 .UNSPECIFIED.);
#691=B_SPLINE_CURVE_WITH_KNOTS('',3,(#28948,#28949,#28950,#28951,#28952,
#28953,#28954,#28955,#28956,#28957),.UNSPECIFIED.,.F.,.F.,(4,1,1,1,1,1,
1,4),(103.672557568463,104.179390217284,105.174703937601,106.170017657919,
107.165331378236,108.160645098554,109.155958818872,109.955742875643),
 .UNSPECIFIED.);
#692=B_SPLINE_CURVE_WITH_KNOTS('',3,(#28958,#28959,#28960,#28961,#28962,
#28963,#28964,#28965,#28966,#28967,#28968),.UNSPECIFIED.,.F.,.F.,(4,1,1,
1,1,1,1,1,4),(103.672557568463,103.852878824536,104.848192544853,105.843506265171,
106.838819985488,107.834133705806,108.829447426123,109.824761146441,109.955742875643),
 .UNSPECIFIED.);
#693=B_SPLINE_CURVE_WITH_KNOTS('',3,(#28973,#28974,#28975,#28976,#28977,
#28978,#28979,#28980,#28981,#28982),.UNSPECIFIED.,.F.,.F.,(4,1,1,1,1,1,
1,4),(97.3893722612837,98.2075078953788,99.2028216156963,100.198135336014,
101.193449056331,102.188762776649,103.184076496966,103.672557568463),
 .UNSPECIFIED.);
#694=B_SPLINE_CURVE_WITH_KNOTS('',3,(#28983,#28984,#28985,#28986,#28987,
#28988,#28989,#28990,#28991,#28992),.UNSPECIFIED.,.F.,.F.,(4,1,1,1,1,1,
1,4),(97.3893722612836,97.8809965026307,98.8763102229482,99.8716239432658,
100.866937663583,101.862251383901,102.857565104218,103.672557568463),
 .UNSPECIFIED.);
#695=B_SPLINE_CURVE_WITH_KNOTS('',3,(#28997,#28998,#28999,#29000,#29001,
#29002,#29003,#29004,#29005,#29006,#29007),.UNSPECIFIED.,.F.,.F.,(4,1,1,
1,1,1,1,1,4),(91.106186954104,91.2403118531562,92.2356255734737,93.2309392937912,
94.2262530141087,95.2215667344263,96.2168804547438,97.2121941750613,97.3893722612837),
 .UNSPECIFIED.);
#696=B_SPLINE_CURVE_WITH_KNOTS('',3,(#29008,#29009,#29010,#29011,#29012,
#29013,#29014,#29015,#29016,#29017),.UNSPECIFIED.,.F.,.F.,(4,1,1,1,1,1,
1,4),(91.106186954104,91.9091141807256,92.9044279010431,93.8997416213606,
94.8950553416782,95.8903690619957,96.8856827823132,97.3893722612836),
 .UNSPECIFIED.);
#697=B_SPLINE_CURVE_WITH_KNOTS('',3,(#29022,#29023,#29024,#29025,#29026,
#29027,#29028,#29029,#29030,#29031),.UNSPECIFIED.,.F.,.F.,(4,1,1,1,1,1,
1,4),(84.8230016469244,85.2684295312511,86.2637432515686,87.2590569718861,
88.2543706922037,89.2496844125212,90.2449981328387,91.106186954104),
 .UNSPECIFIED.);
#698=B_SPLINE_CURVE_WITH_KNOTS('',3,(#29032,#29033,#29034,#29035,#29036,
#29037,#29038,#29039,#29040,#29041,#29042),.UNSPECIFIED.,.F.,.F.,(4,1,1,
1,1,1,1,1,4),(84.8230016469244,84.941918138503,85.9372318588205,86.932545579138,
87.9278592994555,88.9231730197731,89.9184867400906,90.9138004604081,91.106186954104),
 .UNSPECIFIED.);
#699=B_SPLINE_CURVE_WITH_KNOTS('',3,(#29047,#29048,#29049,#29050,#29051,
#29052,#29053,#29054,#29055,#29056),.UNSPECIFIED.,.F.,.F.,(4,1,1,1,1,1,
1,4),(78.5398163397449,79.296547209346,80.2918609296635,81.287174649981,
82.2824883702986,83.2778020906161,84.2731158109336,84.8230016469244),
 .UNSPECIFIED.);
#700=B_SPLINE_CURVE_WITH_KNOTS('',3,(#29057,#29058,#29059,#29060,#29061,
#29062,#29063,#29064,#29065,#29066),.UNSPECIFIED.,.F.,.F.,(4,1,1,1,1,1,
1,4),(78.5398163397448,78.9700358165979,79.9653495369154,80.9606632572329,
81.9559769775504,82.9512906978679,83.9466044181855,84.8230016469244),
 .UNSPECIFIED.);
#701=B_SPLINE_CURVE_WITH_KNOTS('',3,(#29071,#29072,#29073,#29074,#29075,
#29076,#29077,#29078,#29079,#29080,#29081),.UNSPECIFIED.,.F.,.F.,(4,1,1,
1,1,1,1,1,4),(72.2566310325653,72.3293511671233,73.3246648874409,74.3199786077584,
75.3152923280759,76.3106060483934,77.3059197687109,78.3012334890285,78.5398163397449),
 .UNSPECIFIED.);
#702=B_SPLINE_CURVE_WITH_KNOTS('',3,(#29082,#29083,#29084,#29085,#29086,
#29087,#29088,#29089,#29090,#29091),.UNSPECIFIED.,.F.,.F.,(4,1,1,1,1,1,
1,4),(72.2566310325653,72.9981534946928,73.9934672150103,74.9887809353278,
75.9840946556453,76.9794083759628,77.9747220962804,78.5398163397448),
 .UNSPECIFIED.);
#703=B_SPLINE_CURVE_WITH_KNOTS('',3,(#29096,#29097,#29098,#29099,#29100,
#29101,#29102,#29103,#29104,#29105),.UNSPECIFIED.,.F.,.F.,(4,1,1,1,1,1,
1,4),(65.9734457253857,66.3574688452182,67.3527825655358,68.3480962858533,
69.3434100061708,70.3387237264883,71.3340374468058,72.2566310325653),
 .UNSPECIFIED.);
#704=B_SPLINE_CURVE_WITH_KNOTS('',3,(#29106,#29107,#29108,#29109,#29110,
#29111,#29112,#29113,#29114,#29115,#29116),.UNSPECIFIED.,.F.,.F.,(4,1,1,
1,1,1,1,1,4),(65.9734457253856,66.0309574524701,67.0262711727877,68.0215848931052,
69.0168986134227,70.0122123337402,71.0075260540577,72.0028397743752,72.2566310325653),
 .UNSPECIFIED.);
#705=B_SPLINE_CURVE_WITH_KNOTS('',3,(#29121,#29122,#29123,#29124,#29125,
#29126,#29127,#29128,#29129,#29130),.UNSPECIFIED.,.F.,.F.,(4,1,1,1,1,1,
1,4),(59.6902604182061,60.3855865233131,61.3809002436307,62.3762139639482,
63.3715276842657,64.3668414045832,65.3621551249007,65.9734457253857),
 .UNSPECIFIED.);
#706=B_SPLINE_CURVE_WITH_KNOTS('',3,(#29131,#29132,#29133,#29134,#29135,
#29136,#29137,#29138,#29139,#29140),.UNSPECIFIED.,.F.,.F.,(4,1,1,1,1,1,
1,4),(59.6902604182061,60.059075130565,61.0543888508825,62.0497025712001,
63.0450162915176,64.0403300118351,65.0356437321526,65.9734457253856),
 .UNSPECIFIED.);
#707=B_SPLINE_CURVE_WITH_KNOTS('',3,(#29145,#29146,#29147,#29148,#29149,
#29150,#29151,#29152,#29153,#29154,#29155),.UNSPECIFIED.,.F.,.F.,(4,1,1,
1,1,1,1,1,4),(53.4070751110265,53.4183904810905,54.413704201408,55.4090179217255,
56.4043316420431,57.3996453623606,58.3949590826781,59.3902728029956,59.6902604182061),
 .UNSPECIFIED.);
#708=B_SPLINE_CURVE_WITH_KNOTS('',3,(#29156,#29157,#29158,#29159,#29160,
#29161,#29162,#29163,#29164,#29165),.UNSPECIFIED.,.F.,.F.,(4,1,1,1,1,1,
1,4),(53.4070751110265,54.0871928086599,55.0825065289774,56.077820249295,
57.0731339696125,58.06844768993,59.0637614102475,59.6902604182061),
 .UNSPECIFIED.);
#709=B_SPLINE_CURVE_WITH_KNOTS('',3,(#29170,#29171,#29172,#29173,#29174,
#29175,#29176,#29177,#29178,#29179),.UNSPECIFIED.,.F.,.F.,(4,1,1,1,1,1,
1,4),(47.1238898038469,47.4465081591854,48.4418218795029,49.4371355998204,
50.432449320138,51.4277630404555,52.423076760773,53.4070751110265),
 .UNSPECIFIED.);
#710=B_SPLINE_CURVE_WITH_KNOTS('',3,(#29180,#29181,#29182,#29183,#29184,
#29185,#29186,#29187,#29188,#29189),.UNSPECIFIED.,.F.,.F.,(4,1,1,1,1,1,
1,4),(47.1238898038469,48.1153104867548,49.1106242070723,50.1059379273898,
51.1012516477074,52.0965653680249,53.0918790883424,53.4070751110265),
 .UNSPECIFIED.);
#711=B_SPLINE_CURVE_WITH_KNOTS('',3,(#29194,#29195,#29196,#29197,#29198,
#29199,#29200,#29201,#29202,#29203),.UNSPECIFIED.,.F.,.F.,(4,1,1,1,1,1,
1,4),(40.8407044966673,41.4746258372803,42.4699395575978,43.4652532779153,
44.4605669982328,45.4558807185504,46.4511944388679,47.1238898038469),
 .UNSPECIFIED.);
#712=B_SPLINE_CURVE_WITH_KNOTS('',3,(#29204,#29205,#29206,#29207,#29208,
#29209,#29210,#29211,#29212,#29213,#29214),.UNSPECIFIED.,.F.,.F.,(4,1,1,
1,1,1,1,1,4),(40.8407044966673,41.1481144445322,42.1434281648497,43.1387418851672,
44.1340556054847,45.1293693258023,46.1246830461198,47.1199967664373,47.1238898038469),
 .UNSPECIFIED.);
#713=B_SPLINE_CURVE_WITH_KNOTS('',3,(#29219,#29220,#29221,#29222,#29223,
#29224,#29225,#29226,#29227,#29228),.UNSPECIFIED.,.F.,.F.,(4,1,1,1,1,1,
1,4),(34.5575191894877,35.5027435153752,36.4980572356927,37.4933709560102,
38.4886846763277,39.4839983966453,40.4793121169628,40.8407044966673),
 .UNSPECIFIED.);
#714=B_SPLINE_CURVE_WITH_KNOTS('',3,(#29229,#29230,#29231,#29232,#29233,
#29234,#29235,#29236,#29237,#29238),.UNSPECIFIED.,.F.,.F.,(4,1,1,1,1,1,
1,4),(34.5575191894877,35.1762321226271,36.1715458429446,37.1668595632621,
38.1621732835796,39.1574870038972,40.1528007242147,40.8407044966673),
 .UNSPECIFIED.);
#715=B_SPLINE_CURVE_WITH_KNOTS('',3,(#29243,#29244,#29245,#29246,#29247,
#29248,#29249,#29250,#29251,#29252,#29253),.UNSPECIFIED.,.F.,.F.,(4,1,1,
1,1,1,1,1,4),(28.2743338823081,28.5355474731526,29.5308611934701,30.5261749137876,
31.5214886341051,32.5168023544226,33.5121160747401,34.5074297950577,34.5575191894877),
 .UNSPECIFIED.);
#716=B_SPLINE_CURVE_WITH_KNOTS('',3,(#29254,#29255,#29256,#29257,#29258,
#29259,#29260,#29261,#29262,#29263),.UNSPECIFIED.,.F.,.F.,(4,1,1,1,1,1,
1,4),(28.2743338823081,29.204349800722,30.1996635210395,31.194977241357,
32.1902909616745,33.185604681992,34.1809184023096,34.5575191894877),
 .UNSPECIFIED.);
#717=B_SPLINE_CURVE_WITH_KNOTS('',3,(#29268,#29269,#29270,#29271,#29272,
#29273,#29274,#29275,#29276,#29277),.UNSPECIFIED.,.F.,.F.,(4,1,1,1,1,1,
1,4),(21.9911485751286,22.5636651512475,23.558978871565,24.5542925918825,
25.5496063122,26.5449200325175,27.540233752835,28.2743338823081),
 .UNSPECIFIED.);
#718=B_SPLINE_CURVE_WITH_KNOTS('',3,(#29278,#29279,#29280,#29281,#29282,
#29283,#29284,#29285,#29286,#29287,#29288),.UNSPECIFIED.,.F.,.F.,(4,1,1,
1,1,1,1,1,4),(21.9911485751285,22.2371537584993,23.2324674788169,24.2277811991344,
25.2230949194519,26.2184086397694,27.2137223600869,28.2090360804045,28.2743338823081),
 .UNSPECIFIED.);
#719=B_SPLINE_CURVE_WITH_KNOTS('',3,(#29293,#29294,#29295,#29296,#29297,
#29298,#29299,#29300,#29301,#29302),.UNSPECIFIED.,.F.,.F.,(4,1,1,1,1,1,
1,4),(15.707963267949,16.5917828293423,17.5870965496599,18.5824102699774,
19.5777239902949,20.5730377106124,21.5683514309299,21.9911485751286),
 .UNSPECIFIED.);
#720=B_SPLINE_CURVE_WITH_KNOTS('',3,(#29303,#29304,#29305,#29306,#29307,
#29308,#29309,#29310,#29311,#29312),.UNSPECIFIED.,.F.,.F.,(4,1,1,1,1,1,
1,4),(15.7079632679489,16.2652714365942,17.2605851569118,18.2558988772293,
19.2512125975468,20.2465263178643,21.2418400381818,21.9911485751285),
 .UNSPECIFIED.);
#721=B_SPLINE_CURVE_WITH_KNOTS('',3,(#29954,#29955,#29956,#29957,#29958,
#29959,#29960,#29961,#29962,#29963,#29964,#29965,#29966,#29967,#29968,#29969,
#29970,#29971,#29972,#29973,#29974,#29975,#29976,#29977,#29978,#29979,#29980,
#29981,#29982,#29983,#29984,#29985,#29986,#29987,#29988,#29989,#29990,#29991,
#29992,#29993,#29994,#29995,#29996,#29997,#29998,#29999,#30000,#30001,#30002,
#30003,#30004,#30005,#30006,#30007,#30008),.UNSPECIFIED.,.F.,.F.,(4,3,3,
3,3,3,3,3,3,3,3,3,3,3,3,3,3,3,4),(-0.482632075205622,-0.462336249281047,
-0.427687003019698,-0.408173644600383,-0.380690085942371,-0.361844801684832,
-0.34704441187773,-0.301818556126274,-0.266377775059192,-0.255314335513618,
-0.224577305012635,-0.190497645767355,-0.176369177709915,-0.165433267624407,
-0.124074950718305,-0.0869433870803508,-0.0742996259130463,-0.032357512502151,
0.),.UNSPECIFIED.);
#722=B_SPLINE_CURVE_WITH_KNOTS('',3,(#30009,#30010,#30011,#30012),
 .UNSPECIFIED.,.F.,.F.,(4,4),(145.635278351846,146.22857165399),
 .UNSPECIFIED.);
#723=B_SPLINE_CURVE_WITH_KNOTS('',3,(#30014,#30015,#30016,#30017,#30018,
#30019,#30020,#30021,#30022,#30023,#30024,#30025,#30026,#30027,#30028,#30029,
#30030,#30031,#30032,#30033,#30034,#30035,#30036,#30037,#30038,#30039,#30040,
#30041,#30042,#30043,#30044,#30045,#30046,#30047,#30048,#30049,#30050,#30051,
#30052,#30053,#30054,#30055,#30056,#30057,#30058,#30059,#30060,#30061,#30062,
#30063,#30064,#30065,#30066,#30067,#30068),.UNSPECIFIED.,.F.,.F.,(4,3,3,
3,3,3,3,3,3,3,3,3,3,3,3,3,3,3,4),(-0.483882268593951,-0.46576353335263,
-0.430852383331094,-0.416229815277715,-0.375093755185218,-0.358591999734009,
-0.314305848550002,-0.283376081257857,-0.270874225938811,-0.239681235538259,
-0.209721081095977,-0.193164961501836,-0.179875924261507,-0.13490694319613,
-0.112773483820775,-0.0967277303364094,-0.0829938450850564,-0.0368476966362759,
0.),.UNSPECIFIED.);
#724=B_SPLINE_CURVE_WITH_KNOTS('',3,(#30069,#30070,#30071,#30072,#30073,
#30074,#30075,#30076,#30077),.UNSPECIFIED.,.F.,.F.,(4,1,1,1,1,1,4),(10.3759343473738,
11.2887028350066,12.2840165553242,13.2793302756417,14.2746439959592,15.2699577162767,
15.7079632679489),.UNSPECIFIED.);
#725=B_SPLINE_CURVE_WITH_KNOTS('',3,(#30083,#30084,#30085,#30086,#30087,
#30088,#30089,#30090,#30091,#30092,#30093,#30094,#30095,#30096,#30097,#30098,
#30099,#30100,#30101,#30102,#30103,#30104,#30105,#30106,#30107,#30108,#30109,
#30110,#30111,#30112,#30113,#30114,#30115,#30116,#30117,#30118,#30119,#30120,
#30121,#30122,#30123,#30124,#30125,#30126,#30127,#30128,#30129,#30130,#30131,
#30132,#30133,#30134,#30135,#30136,#30137),.UNSPECIFIED.,.F.,.F.,(4,3,3,
3,3,3,3,3,3,3,3,3,3,3,3,3,3,3,4),(-0.482632075205632,-0.462336249281051,
-0.427686999954685,-0.408173642759644,-0.380690078686806,-0.361844802480269,
-0.347044410218777,-0.301818552387021,-0.26637777077025,-0.255314327560454,
-0.224577305012648,-0.190497642723496,-0.176369168534599,-0.16543325457945,
-0.124074940934588,-0.0869433711633969,-0.0742996240346052,-0.0323575236186803,
0.),.UNSPECIFIED.);
#726=B_SPLINE_CURVE_WITH_KNOTS('',3,(#30140,#30141,#30142,#30143,#30144,
#30145,#30146,#30147),.UNSPECIFIED.,.F.,.F.,(4,1,1,1,1,4),(11.6152142277548,
12.6105279480723,13.6058416683898,14.6011553887073,15.5964691090248,15.707963267949),
 .UNSPECIFIED.);
#727=B_SPLINE_CURVE_WITH_KNOTS('',3,(#30756,#30757,#30758,#30759,#30760,
#30761,#30762,#30763,#30764,#30765,#30766,#30767,#30768,#30769,#30770,#30771,
#30772,#30773,#30774,#30775,#30776,#30777,#30778,#30779,#30780,#30781,#30782,
#30783,#30784,#30785,#30786,#30787,#30788,#30789,#30790,#30791,#30792,#30793,
#30794,#30795,#30796,#30797,#30798,#30799,#30800,#30801,#30802,#30803,#30804,
#30805,#30806,#30807,#30808,#30809,#30810),.UNSPECIFIED.,.F.,.F.,(4,3,3,
3,3,3,3,3,3,3,3,3,3,3,3,3,3,3,4),(-0.483882268593942,-0.465763533352619,
-0.4308523820833,-0.416229812750554,-0.375093593923325,-0.358591971446984,
-0.314305820036663,-0.283376059421202,-0.270874217660563,-0.239681235538257,
-0.209721081095975,-0.19316496451099,-0.179875924603182,-0.134906943452387,
-0.112773485311706,-0.0967277413707433,-0.0829938472014202,-0.0368477058416217,
0.),.UNSPECIFIED.);
#949=CYLINDRICAL_SURFACE('',#17099,0.24635);
#950=CYLINDRICAL_SURFACE('',#17101,0.24635);
#951=CYLINDRICAL_SURFACE('',#17102,0.24635);
#952=CYLINDRICAL_SURFACE('',#17103,0.24635);
#953=CYLINDRICAL_SURFACE('',#17104,0.24635);
#954=CYLINDRICAL_SURFACE('',#17105,0.24635);
#955=CYLINDRICAL_SURFACE('',#17106,0.24635);
#956=CYLINDRICAL_SURFACE('',#17107,0.24635);
#957=CYLINDRICAL_SURFACE('',#17108,0.24635);
#958=CYLINDRICAL_SURFACE('',#17109,0.24635);
#959=CYLINDRICAL_SURFACE('',#17110,0.24635);
#960=CYLINDRICAL_SURFACE('',#17111,0.24635);
#961=CYLINDRICAL_SURFACE('',#17112,0.24635);
#962=CYLINDRICAL_SURFACE('',#17113,0.24635);
#963=CYLINDRICAL_SURFACE('',#17114,0.24635);
#964=CYLINDRICAL_SURFACE('',#17115,0.24635);
#965=CYLINDRICAL_SURFACE('',#17116,0.24635);
#966=CYLINDRICAL_SURFACE('',#17117,0.24635);
#967=CYLINDRICAL_SURFACE('',#17118,0.24635);
#968=CYLINDRICAL_SURFACE('',#17119,0.24635);
#969=CYLINDRICAL_SURFACE('',#17120,0.24635);
#970=CYLINDRICAL_SURFACE('',#17121,0.24635);
#971=CYLINDRICAL_SURFACE('',#17122,0.24635);
#972=CYLINDRICAL_SURFACE('',#17123,0.24635);
#973=CYLINDRICAL_SURFACE('',#17125,0.217775);
#974=CYLINDRICAL_SURFACE('',#17127,0.217775);
#975=CYLINDRICAL_SURFACE('',#17128,0.217775);
#976=CYLINDRICAL_SURFACE('',#17129,0.217775);
#977=CYLINDRICAL_SURFACE('',#17130,0.217775);
#978=CYLINDRICAL_SURFACE('',#17131,0.217775);
#979=CYLINDRICAL_SURFACE('',#17132,0.217775);
#980=CYLINDRICAL_SURFACE('',#17133,0.217775);
#981=CYLINDRICAL_SURFACE('',#17134,0.217775);
#982=CYLINDRICAL_SURFACE('',#17135,0.217775);
#983=CYLINDRICAL_SURFACE('',#17136,0.217775);
#984=CYLINDRICAL_SURFACE('',#17137,0.217775);
#985=CYLINDRICAL_SURFACE('',#17138,0.217775);
#986=CYLINDRICAL_SURFACE('',#17139,0.217775);
#987=CYLINDRICAL_SURFACE('',#17140,0.217775);
#988=CYLINDRICAL_SURFACE('',#17141,0.217775);
#989=CYLINDRICAL_SURFACE('',#17142,0.217775);
#990=CYLINDRICAL_SURFACE('',#17143,0.217775);
#991=CYLINDRICAL_SURFACE('',#17144,0.217775);
#992=CYLINDRICAL_SURFACE('',#17145,0.217775);
#993=CYLINDRICAL_SURFACE('',#17146,0.217775);
#994=CYLINDRICAL_SURFACE('',#17147,0.217775);
#995=CYLINDRICAL_SURFACE('',#17148,0.217775);
#996=CYLINDRICAL_SURFACE('',#17154,0.151);
#997=CYLINDRICAL_SURFACE('',#17162,0.217775);
#998=CYLINDRICAL_SURFACE('',#17223,0.5);
#999=CYLINDRICAL_SURFACE('',#17226,0.5);
#1000=CYLINDRICAL_SURFACE('',#17229,0.5);
#1001=CYLINDRICAL_SURFACE('',#17232,0.5);
#1002=CYLINDRICAL_SURFACE('',#17235,0.5);
#1003=CYLINDRICAL_SURFACE('',#17238,0.5);
#1004=CYLINDRICAL_SURFACE('',#17241,0.5);
#1005=CYLINDRICAL_SURFACE('',#17244,0.5);
#1006=CYLINDRICAL_SURFACE('',#17247,0.5);
#1007=CYLINDRICAL_SURFACE('',#17250,0.5);
#1008=CYLINDRICAL_SURFACE('',#17253,0.5);
#1009=CYLINDRICAL_SURFACE('',#17256,0.5);
#1010=CYLINDRICAL_SURFACE('',#17259,0.5);
#1011=CYLINDRICAL_SURFACE('',#17262,0.5);
#1012=CYLINDRICAL_SURFACE('',#17265,0.5);
#1013=CYLINDRICAL_SURFACE('',#17268,0.5);
#1014=CYLINDRICAL_SURFACE('',#17271,0.5);
#1015=CYLINDRICAL_SURFACE('',#17274,0.5);
#1016=CYLINDRICAL_SURFACE('',#17277,0.5);
#1017=CYLINDRICAL_SURFACE('',#17280,0.5);
#1018=CYLINDRICAL_SURFACE('',#17283,0.5);
#1019=CYLINDRICAL_SURFACE('',#17286,0.5);
#1020=CYLINDRICAL_SURFACE('',#17289,0.5);
#1021=CYLINDRICAL_SURFACE('',#17292,0.5);
#1022=CYLINDRICAL_SURFACE('',#17295,0.5);
#1023=CYLINDRICAL_SURFACE('',#17298,0.5);
#1024=CYLINDRICAL_SURFACE('',#17301,0.5);
#1025=CYLINDRICAL_SURFACE('',#17304,0.5);
#1026=CYLINDRICAL_SURFACE('',#17307,0.5);
#1027=CYLINDRICAL_SURFACE('',#17310,0.5);
#1028=CYLINDRICAL_SURFACE('',#17318,0.24635);
#1199=FACE_BOUND('',#3339,.T.);
#1200=FACE_BOUND('',#3343,.T.);
#1201=FACE_BOUND('',#3346,.T.);
#1443=CIRCLE('',#17100,0.24635);
#1444=CIRCLE('',#17124,0.24635);
#1445=CIRCLE('',#17126,0.217775);
#1446=CIRCLE('',#17155,0.151);
#1447=CIRCLE('',#17156,0.151);
#1448=CIRCLE('',#17159,0.24635);
#1449=CIRCLE('',#17160,0.24635);
#1450=CIRCLE('',#17161,0.217775);
#1451=CIRCLE('',#17224,0.5);
#1452=CIRCLE('',#17225,0.5);
#1453=CIRCLE('',#17227,0.5);
#1454=CIRCLE('',#17228,0.5);
#1455=CIRCLE('',#17230,0.5);
#1456=CIRCLE('',#17231,0.5);
#1457=CIRCLE('',#17233,0.5);
#1458=CIRCLE('',#17234,0.5);
#1459=CIRCLE('',#17236,0.5);
#1460=CIRCLE('',#17237,0.5);
#1461=CIRCLE('',#17239,0.5);
#1462=CIRCLE('',#17240,0.5);
#1463=CIRCLE('',#17242,0.5);
#1464=CIRCLE('',#17243,0.5);
#1465=CIRCLE('',#17245,0.5);
#1466=CIRCLE('',#17246,0.5);
#1467=CIRCLE('',#17248,0.5);
#1468=CIRCLE('',#17249,0.5);
#1469=CIRCLE('',#17251,0.5);
#1470=CIRCLE('',#17252,0.5);
#1471=CIRCLE('',#17254,0.5);
#1472=CIRCLE('',#17255,0.5);
#1473=CIRCLE('',#17257,0.5);
#1474=CIRCLE('',#17258,0.5);
#1475=CIRCLE('',#17260,0.5);
#1476=CIRCLE('',#17261,0.5);
#1477=CIRCLE('',#17263,0.5);
#1478=CIRCLE('',#17264,0.5);
#1479=CIRCLE('',#17266,0.5);
#1480=CIRCLE('',#17267,0.5);
#1481=CIRCLE('',#17269,0.5);
#1482=CIRCLE('',#17270,0.5);
#1483=CIRCLE('',#17272,0.5);
#1484=CIRCLE('',#17273,0.5);
#1485=CIRCLE('',#17275,0.5);
#1486=CIRCLE('',#17276,0.5);
#1487=CIRCLE('',#17278,0.5);
#1488=CIRCLE('',#17279,0.5);
#1489=CIRCLE('',#17281,0.5);
#1490=CIRCLE('',#17282,0.5);
#1491=CIRCLE('',#17284,0.5);
#1492=CIRCLE('',#17285,0.5);
#1493=CIRCLE('',#17287,0.5);
#1494=CIRCLE('',#17288,0.5);
#1495=CIRCLE('',#17290,0.5);
#1496=CIRCLE('',#17291,0.5);
#1497=CIRCLE('',#17293,0.5);
#1498=CIRCLE('',#17294,0.5);
#1499=CIRCLE('',#17296,0.5);
#1500=CIRCLE('',#17297,0.5);
#1501=CIRCLE('',#17299,0.5);
#1502=CIRCLE('',#17300,0.5);
#1503=CIRCLE('',#17302,0.5);
#1504=CIRCLE('',#17303,0.5);
#1505=CIRCLE('',#17305,0.5);
#1506=CIRCLE('',#17306,0.5);
#1507=CIRCLE('',#17308,0.5);
#1508=CIRCLE('',#17309,0.5);
#1509=CIRCLE('',#17311,0.5);
#1510=CIRCLE('',#17312,0.5);
#1511=CIRCLE('',#17314,0.45);
#1512=CIRCLE('',#17316,0.21);
#1513=CIRCLE('',#17319,0.24635);
#1514=CIRCLE('',#17322,0.44);
#1765=CONICAL_SURFACE('',#17313,0.475,0.785398163397448);
#1766=CONICAL_SURFACE('',#17317,0.23,0.785398163397448);
#1767=CONICAL_SURFACE('',#17321,0.47,0.785398163397448);
#2232=FACE_OUTER_BOUND('',#3189,.T.);
#2233=FACE_OUTER_BOUND('',#3190,.T.);
#2234=FACE_OUTER_BOUND('',#3191,.T.);
#2235=FACE_OUTER_BOUND('',#3192,.T.);
#2236=FACE_OUTER_BOUND('',#3193,.T.);
#2237=FACE_OUTER_BOUND('',#3194,.T.);
#2238=FACE_OUTER_BOUND('',#3195,.T.);
#2239=FACE_OUTER_BOUND('',#3196,.T.);
#2240=FACE_OUTER_BOUND('',#3197,.T.);
#2241=FACE_OUTER_BOUND('',#3198,.T.);
#2242=FACE_OUTER_BOUND('',#3199,.T.);
#2243=FACE_OUTER_BOUND('',#3200,.T.);
#2244=FACE_OUTER_BOUND('',#3201,.T.);
#2245=FACE_OUTER_BOUND('',#3202,.T.);
#2246=FACE_OUTER_BOUND('',#3203,.T.);
#2247=FACE_OUTER_BOUND('',#3204,.T.);
#2248=FACE_OUTER_BOUND('',#3205,.T.);
#2249=FACE_OUTER_BOUND('',#3206,.T.);
#2250=FACE_OUTER_BOUND('',#3207,.T.);
#2251=FACE_OUTER_BOUND('',#3208,.T.);
#2252=FACE_OUTER_BOUND('',#3209,.T.);
#2253=FACE_OUTER_BOUND('',#3210,.T.);
#2254=FACE_OUTER_BOUND('',#3211,.T.);
#2255=FACE_OUTER_BOUND('',#3212,.T.);
#2256=FACE_OUTER_BOUND('',#3213,.T.);
#2257=FACE_OUTER_BOUND('',#3214,.T.);
#2258=FACE_OUTER_BOUND('',#3215,.T.);
#2259=FACE_OUTER_BOUND('',#3216,.T.);
#2260=FACE_OUTER_BOUND('',#3217,.T.);
#2261=FACE_OUTER_BOUND('',#3218,.T.);
#2262=FACE_OUTER_BOUND('',#3219,.T.);
#2263=FACE_OUTER_BOUND('',#3220,.T.);
#2264=FACE_OUTER_BOUND('',#3221,.T.);
#2265=FACE_OUTER_BOUND('',#3222,.T.);
#2266=FACE_OUTER_BOUND('',#3223,.T.);
#2267=FACE_OUTER_BOUND('',#3224,.T.);
#2268=FACE_OUTER_BOUND('',#3225,.T.);
#2269=FACE_OUTER_BOUND('',#3226,.T.);
#2270=FACE_OUTER_BOUND('',#3227,.T.);
#2271=FACE_OUTER_BOUND('',#3228,.T.);
#2272=FACE_OUTER_BOUND('',#3229,.T.);
#2273=FACE_OUTER_BOUND('',#3230,.T.);
#2274=FACE_OUTER_BOUND('',#3231,.T.);
#2275=FACE_OUTER_BOUND('',#3232,.T.);
#2276=FACE_OUTER_BOUND('',#3233,.T.);
#2277=FACE_OUTER_BOUND('',#3234,.T.);
#2278=FACE_OUTER_BOUND('',#3235,.T.);
#2279=FACE_OUTER_BOUND('',#3236,.T.);
#2280=FACE_OUTER_BOUND('',#3237,.T.);
#2281=FACE_OUTER_BOUND('',#3238,.T.);
#2282=FACE_OUTER_BOUND('',#3239,.T.);
#2283=FACE_OUTER_BOUND('',#3240,.T.);
#2284=FACE_OUTER_BOUND('',#3241,.T.);
#2285=FACE_OUTER_BOUND('',#3242,.T.);
#2286=FACE_OUTER_BOUND('',#3243,.T.);
#2287=FACE_OUTER_BOUND('',#3244,.T.);
#2288=FACE_OUTER_BOUND('',#3245,.T.);
#2289=FACE_OUTER_BOUND('',#3246,.T.);
#2290=FACE_OUTER_BOUND('',#3247,.T.);
#2291=FACE_OUTER_BOUND('',#3248,.T.);
#2292=FACE_OUTER_BOUND('',#3249,.T.);
#2293=FACE_OUTER_BOUND('',#3250,.T.);
#2294=FACE_OUTER_BOUND('',#3251,.T.);
#2295=FACE_OUTER_BOUND('',#3252,.T.);
#2296=FACE_OUTER_BOUND('',#3253,.T.);
#2297=FACE_OUTER_BOUND('',#3254,.T.);
#2298=FACE_OUTER_BOUND('',#3255,.T.);
#2299=FACE_OUTER_BOUND('',#3256,.T.);
#2300=FACE_OUTER_BOUND('',#3257,.T.);
#2301=FACE_OUTER_BOUND('',#3258,.T.);
#2302=FACE_OUTER_BOUND('',#3259,.T.);
#2303=FACE_OUTER_BOUND('',#3260,.T.);
#2304=FACE_OUTER_BOUND('',#3261,.T.);
#2305=FACE_OUTER_BOUND('',#3262,.T.);
#2306=FACE_OUTER_BOUND('',#3263,.T.);
#2307=FACE_OUTER_BOUND('',#3264,.T.);
#2308=FACE_OUTER_BOUND('',#3265,.T.);
#2309=FACE_OUTER_BOUND('',#3266,.T.);
#2310=FACE_OUTER_BOUND('',#3267,.T.);
#2311=FACE_OUTER_BOUND('',#3268,.T.);
#2312=FACE_OUTER_BOUND('',#3269,.T.);
#2313=FACE_OUTER_BOUND('',#3270,.T.);
#2314=FACE_OUTER_BOUND('',#3271,.T.);
#2315=FACE_OUTER_BOUND('',#3272,.T.);
#2316=FACE_OUTER_BOUND('',#3273,.T.);
#2317=FACE_OUTER_BOUND('',#3274,.T.);
#2318=FACE_OUTER_BOUND('',#3275,.T.);
#2319=FACE_OUTER_BOUND('',#3276,.T.);
#2320=FACE_OUTER_BOUND('',#3277,.T.);
#2321=FACE_OUTER_BOUND('',#3278,.T.);
#2322=FACE_OUTER_BOUND('',#3279,.T.);
#2323=FACE_OUTER_BOUND('',#3280,.T.);
#2324=FACE_OUTER_BOUND('',#3281,.T.);
#2325=FACE_OUTER_BOUND('',#3282,.T.);
#2326=FACE_OUTER_BOUND('',#3283,.T.);
#2327=FACE_OUTER_BOUND('',#3284,.T.);
#2328=FACE_OUTER_BOUND('',#3285,.T.);
#2329=FACE_OUTER_BOUND('',#3286,.T.);
#2330=FACE_OUTER_BOUND('',#3287,.T.);
#2331=FACE_OUTER_BOUND('',#3288,.T.);
#2332=FACE_OUTER_BOUND('',#3289,.T.);
#2333=FACE_OUTER_BOUND('',#3290,.T.);
#2334=FACE_OUTER_BOUND('',#3291,.T.);
#2335=FACE_OUTER_BOUND('',#3292,.T.);
#2336=FACE_OUTER_BOUND('',#3293,.T.);
#2337=FACE_OUTER_BOUND('',#3294,.T.);
#2338=FACE_OUTER_BOUND('',#3295,.T.);
#2339=FACE_OUTER_BOUND('',#3296,.T.);
#2340=FACE_OUTER_BOUND('',#3297,.T.);
#2341=FACE_OUTER_BOUND('',#3298,.T.);
#2342=FACE_OUTER_BOUND('',#3299,.T.);
#2343=FACE_OUTER_BOUND('',#3300,.T.);
#2344=FACE_OUTER_BOUND('',#3301,.T.);
#2345=FACE_OUTER_BOUND('',#3302,.T.);
#2346=FACE_OUTER_BOUND('',#3303,.T.);
#2347=FACE_OUTER_BOUND('',#3304,.T.);
#2348=FACE_OUTER_BOUND('',#3305,.T.);
#2349=FACE_OUTER_BOUND('',#3306,.T.);
#2350=FACE_OUTER_BOUND('',#3307,.T.);
#2351=FACE_OUTER_BOUND('',#3308,.T.);
#2352=FACE_OUTER_BOUND('',#3309,.T.);
#2353=FACE_OUTER_BOUND('',#3310,.T.);
#2354=FACE_OUTER_BOUND('',#3311,.T.);
#2355=FACE_OUTER_BOUND('',#3312,.T.);
#2356=FACE_OUTER_BOUND('',#3313,.T.);
#2357=FACE_OUTER_BOUND('',#3314,.T.);
#2358=FACE_OUTER_BOUND('',#3315,.T.);
#2359=FACE_OUTER_BOUND('',#3316,.T.);
#2360=FACE_OUTER_BOUND('',#3317,.T.);
#2361=FACE_OUTER_BOUND('',#3318,.T.);
#2362=FACE_OUTER_BOUND('',#3319,.T.);
#2363=FACE_OUTER_BOUND('',#3320,.T.);
#2364=FACE_OUTER_BOUND('',#3321,.T.);
#2365=FACE_OUTER_BOUND('',#3322,.T.);
#2366=FACE_OUTER_BOUND('',#3323,.T.);
#2367=FACE_OUTER_BOUND('',#3324,.T.);
#2368=FACE_OUTER_BOUND('',#3325,.T.);
#2369=FACE_OUTER_BOUND('',#3326,.T.);
#2370=FACE_OUTER_BOUND('',#3327,.T.);
#2371=FACE_OUTER_BOUND('',#3328,.T.);
#2372=FACE_OUTER_BOUND('',#3329,.T.);
#2373=FACE_OUTER_BOUND('',#3330,.T.);
#2374=FACE_OUTER_BOUND('',#3331,.T.);
#2375=FACE_OUTER_BOUND('',#3332,.T.);
#2376=FACE_OUTER_BOUND('',#3333,.T.);
#2377=FACE_OUTER_BOUND('',#3334,.T.);
#2378=FACE_OUTER_BOUND('',#3335,.T.);
#2379=FACE_OUTER_BOUND('',#3336,.T.);
#2380=FACE_OUTER_BOUND('',#3337,.T.);
#2381=FACE_OUTER_BOUND('',#3338,.T.);
#2382=FACE_OUTER_BOUND('',#3340,.T.);
#2383=FACE_OUTER_BOUND('',#3341,.T.);
#2384=FACE_OUTER_BOUND('',#3342,.T.);
#2385=FACE_OUTER_BOUND('',#3344,.T.);
#2386=FACE_OUTER_BOUND('',#3345,.T.);
#3189=EDGE_LOOP('',(#12223,#12224,#12225,#12226));
#3190=EDGE_LOOP('',(#12227,#12228,#12229,#12230));
#3191=EDGE_LOOP('',(#12231,#12232,#12233,#12234));
#3192=EDGE_LOOP('',(#12235,#12236,#12237,#12238));
#3193=EDGE_LOOP('',(#12239,#12240,#12241,#12242));
#3194=EDGE_LOOP('',(#12243,#12244,#12245,#12246));
#3195=EDGE_LOOP('',(#12247,#12248,#12249,#12250));
#3196=EDGE_LOOP('',(#12251,#12252,#12253,#12254));
#3197=EDGE_LOOP('',(#12255,#12256,#12257,#12258));
#3198=EDGE_LOOP('',(#12259,#12260,#12261,#12262));
#3199=EDGE_LOOP('',(#12263,#12264,#12265,#12266));
#3200=EDGE_LOOP('',(#12267,#12268,#12269,#12270));
#3201=EDGE_LOOP('',(#12271,#12272,#12273,#12274));
#3202=EDGE_LOOP('',(#12275,#12276,#12277,#12278));
#3203=EDGE_LOOP('',(#12279,#12280,#12281,#12282));
#3204=EDGE_LOOP('',(#12283,#12284,#12285,#12286));
#3205=EDGE_LOOP('',(#12287,#12288,#12289,#12290));
#3206=EDGE_LOOP('',(#12291,#12292,#12293,#12294));
#3207=EDGE_LOOP('',(#12295,#12296,#12297,#12298));
#3208=EDGE_LOOP('',(#12299,#12300,#12301,#12302));
#3209=EDGE_LOOP('',(#12303,#12304,#12305,#12306));
#3210=EDGE_LOOP('',(#12307,#12308,#12309,#12310));
#3211=EDGE_LOOP('',(#12311,#12312,#12313,#12314));
#3212=EDGE_LOOP('',(#12315,#12316,#12317,#12318,#12319));
#3213=EDGE_LOOP('',(#12320,#12321,#12322,#12323));
#3214=EDGE_LOOP('',(#12324,#12325,#12326,#12327));
#3215=EDGE_LOOP('',(#12328,#12329,#12330,#12331));
#3216=EDGE_LOOP('',(#12332,#12333,#12334,#12335));
#3217=EDGE_LOOP('',(#12336,#12337,#12338,#12339));
#3218=EDGE_LOOP('',(#12340,#12341,#12342,#12343));
#3219=EDGE_LOOP('',(#12344,#12345,#12346,#12347));
#3220=EDGE_LOOP('',(#12348,#12349,#12350,#12351));
#3221=EDGE_LOOP('',(#12352,#12353,#12354,#12355));
#3222=EDGE_LOOP('',(#12356,#12357,#12358,#12359));
#3223=EDGE_LOOP('',(#12360,#12361,#12362,#12363));
#3224=EDGE_LOOP('',(#12364,#12365,#12366,#12367));
#3225=EDGE_LOOP('',(#12368,#12369,#12370,#12371));
#3226=EDGE_LOOP('',(#12372,#12373,#12374,#12375));
#3227=EDGE_LOOP('',(#12376,#12377,#12378,#12379));
#3228=EDGE_LOOP('',(#12380,#12381,#12382,#12383));
#3229=EDGE_LOOP('',(#12384,#12385,#12386,#12387));
#3230=EDGE_LOOP('',(#12388,#12389,#12390,#12391));
#3231=EDGE_LOOP('',(#12392,#12393,#12394,#12395));
#3232=EDGE_LOOP('',(#12396,#12397,#12398,#12399));
#3233=EDGE_LOOP('',(#12400,#12401,#12402,#12403));
#3234=EDGE_LOOP('',(#12404,#12405,#12406,#12407));
#3235=EDGE_LOOP('',(#12408,#12409,#12410,#12411));
#3236=EDGE_LOOP('',(#12412,#12413,#12414,#12415));
#3237=EDGE_LOOP('',(#12416,#12417,#12418,#12419));
#3238=EDGE_LOOP('',(#12420,#12421,#12422,#12423));
#3239=EDGE_LOOP('',(#12424,#12425,#12426,#12427));
#3240=EDGE_LOOP('',(#12428,#12429,#12430,#12431));
#3241=EDGE_LOOP('',(#12432,#12433,#12434,#12435));
#3242=EDGE_LOOP('',(#12436));
#3243=EDGE_LOOP('',(#12437,#12438,#12439,#12440,#12441,#12442,#12443,#12444,
#12445,#12446,#12447,#12448,#12449,#12450,#12451,#12452,#12453,#12454,#12455,
#12456,#12457,#12458,#12459,#12460,#12461,#12462,#12463,#12464,#12465,#12466,
#12467,#12468,#12469,#12470,#12471,#12472,#12473,#12474,#12475,#12476,#12477,
#12478,#12479,#12480,#12481,#12482,#12483,#12484,#12485,#12486,#12487));
#3244=EDGE_LOOP('',(#12488,#12489,#12490,#12491,#12492));
#3245=EDGE_LOOP('',(#12493,#12494,#12495,#12496));
#3246=EDGE_LOOP('',(#12497,#12498,#12499,#12500,#12501,#12502,#12503,#12504,
#12505,#12506,#12507,#12508,#12509,#12510,#12511,#12512,#12513,#12514,#12515,
#12516,#12517,#12518,#12519,#12520,#12521,#12522,#12523,#12524,#12525,#12526,
#12527,#12528,#12529,#12530,#12531,#12532,#12533,#12534,#12535,#12536,#12537,
#12538,#12539,#12540,#12541,#12542,#12543,#12544,#12545,#12546));
#3247=EDGE_LOOP('',(#12547,#12548,#12549,#12550));
#3248=EDGE_LOOP('',(#12551,#12552,#12553,#12554));
#3249=EDGE_LOOP('',(#12555,#12556,#12557,#12558));
#3250=EDGE_LOOP('',(#12559,#12560,#12561,#12562));
#3251=EDGE_LOOP('',(#12563,#12564,#12565,#12566));
#3252=EDGE_LOOP('',(#12567,#12568,#12569,#12570));
#3253=EDGE_LOOP('',(#12571,#12572,#12573,#12574));
#3254=EDGE_LOOP('',(#12575,#12576,#12577,#12578));
#3255=EDGE_LOOP('',(#12579,#12580,#12581,#12582));
#3256=EDGE_LOOP('',(#12583,#12584,#12585,#12586));
#3257=EDGE_LOOP('',(#12587,#12588,#12589,#12590));
#3258=EDGE_LOOP('',(#12591,#12592,#12593,#12594));
#3259=EDGE_LOOP('',(#12595,#12596,#12597,#12598));
#3260=EDGE_LOOP('',(#12599,#12600,#12601,#12602));
#3261=EDGE_LOOP('',(#12603,#12604,#12605,#12606));
#3262=EDGE_LOOP('',(#12607,#12608,#12609,#12610));
#3263=EDGE_LOOP('',(#12611,#12612,#12613,#12614));
#3264=EDGE_LOOP('',(#12615,#12616,#12617,#12618));
#3265=EDGE_LOOP('',(#12619,#12620,#12621,#12622));
#3266=EDGE_LOOP('',(#12623,#12624,#12625,#12626));
#3267=EDGE_LOOP('',(#12627,#12628,#12629,#12630));
#3268=EDGE_LOOP('',(#12631,#12632,#12633,#12634));
#3269=EDGE_LOOP('',(#12635,#12636,#12637,#12638));
#3270=EDGE_LOOP('',(#12639,#12640,#12641,#12642));
#3271=EDGE_LOOP('',(#12643,#12644,#12645,#12646));
#3272=EDGE_LOOP('',(#12647,#12648,#12649,#12650));
#3273=EDGE_LOOP('',(#12651,#12652,#12653,#12654));
#3274=EDGE_LOOP('',(#12655,#12656,#12657,#12658));
#3275=EDGE_LOOP('',(#12659,#12660,#12661,#12662));
#3276=EDGE_LOOP('',(#12663,#12664,#12665,#12666));
#3277=EDGE_LOOP('',(#12667,#12668,#12669,#12670));
#3278=EDGE_LOOP('',(#12671,#12672,#12673,#12674));
#3279=EDGE_LOOP('',(#12675,#12676,#12677,#12678));
#3280=EDGE_LOOP('',(#12679,#12680,#12681,#12682));
#3281=EDGE_LOOP('',(#12683,#12684,#12685,#12686));
#3282=EDGE_LOOP('',(#12687,#12688,#12689,#12690));
#3283=EDGE_LOOP('',(#12691,#12692,#12693,#12694));
#3284=EDGE_LOOP('',(#12695,#12696,#12697,#12698));
#3285=EDGE_LOOP('',(#12699,#12700,#12701,#12702));
#3286=EDGE_LOOP('',(#12703,#12704,#12705,#12706));
#3287=EDGE_LOOP('',(#12707,#12708,#12709,#12710));
#3288=EDGE_LOOP('',(#12711,#12712,#12713,#12714));
#3289=EDGE_LOOP('',(#12715,#12716,#12717,#12718));
#3290=EDGE_LOOP('',(#12719,#12720,#12721,#12722));
#3291=EDGE_LOOP('',(#12723,#12724,#12725,#12726));
#3292=EDGE_LOOP('',(#12727,#12728,#12729,#12730));
#3293=EDGE_LOOP('',(#12731,#12732,#12733,#12734));
#3294=EDGE_LOOP('',(#12735,#12736,#12737,#12738));
#3295=EDGE_LOOP('',(#12739,#12740,#12741,#12742));
#3296=EDGE_LOOP('',(#12743,#12744,#12745,#12746));
#3297=EDGE_LOOP('',(#12747,#12748,#12749,#12750));
#3298=EDGE_LOOP('',(#12751,#12752,#12753,#12754));
#3299=EDGE_LOOP('',(#12755,#12756,#12757,#12758));
#3300=EDGE_LOOP('',(#12759,#12760,#12761,#12762));
#3301=EDGE_LOOP('',(#12763,#12764,#12765,#12766));
#3302=EDGE_LOOP('',(#12767,#12768,#12769,#12770));
#3303=EDGE_LOOP('',(#12771,#12772,#12773,#12774));
#3304=EDGE_LOOP('',(#12775,#12776,#12777,#12778));
#3305=EDGE_LOOP('',(#12779,#12780,#12781,#12782));
#3306=EDGE_LOOP('',(#12783,#12784,#12785,#12786));
#3307=EDGE_LOOP('',(#12787,#12788,#12789,#12790));
#3308=EDGE_LOOP('',(#12791,#12792,#12793,#12794));
#3309=EDGE_LOOP('',(#12795,#12796,#12797,#12798));
#3310=EDGE_LOOP('',(#12799,#12800,#12801,#12802));
#3311=EDGE_LOOP('',(#12803,#12804,#12805,#12806));
#3312=EDGE_LOOP('',(#12807,#12808,#12809,#12810));
#3313=EDGE_LOOP('',(#12811,#12812,#12813,#12814));
#3314=EDGE_LOOP('',(#12815,#12816,#12817,#12818));
#3315=EDGE_LOOP('',(#12819,#12820,#12821,#12822));
#3316=EDGE_LOOP('',(#12823,#12824,#12825,#12826));
#3317=EDGE_LOOP('',(#12827,#12828,#12829,#12830));
#3318=EDGE_LOOP('',(#12831,#12832,#12833,#12834));
#3319=EDGE_LOOP('',(#12835,#12836,#12837,#12838));
#3320=EDGE_LOOP('',(#12839,#12840,#12841,#12842));
#3321=EDGE_LOOP('',(#12843,#12844,#12845,#12846));
#3322=EDGE_LOOP('',(#12847,#12848,#12849,#12850));
#3323=EDGE_LOOP('',(#12851,#12852,#12853,#12854));
#3324=EDGE_LOOP('',(#12855,#12856,#12857,#12858));
#3325=EDGE_LOOP('',(#12859,#12860,#12861,#12862));
#3326=EDGE_LOOP('',(#12863,#12864,#12865,#12866));
#3327=EDGE_LOOP('',(#12867,#12868,#12869,#12870));
#3328=EDGE_LOOP('',(#12871,#12872,#12873,#12874));
#3329=EDGE_LOOP('',(#12875,#12876,#12877,#12878));
#3330=EDGE_LOOP('',(#12879,#12880,#12881,#12882));
#3331=EDGE_LOOP('',(#12883,#12884,#12885,#12886));
#3332=EDGE_LOOP('',(#12887,#12888,#12889,#12890));
#3333=EDGE_LOOP('',(#12891,#12892,#12893,#12894));
#3334=EDGE_LOOP('',(#12895,#12896,#12897,#12898));
#3335=EDGE_LOOP('',(#12899,#12900,#12901,#12902));
#3336=EDGE_LOOP('',(#12903,#12904,#12905,#12906));
#3337=EDGE_LOOP('',(#12907,#12908,#12909,#12910,#12911,#12912,#12913,#12914,
#12915,#12916,#12917,#12918,#12919,#12920,#12921,#12922,#12923,#12924,#12925,
#12926,#12927,#12928,#12929,#12930,#12931,#12932,#12933,#12934,#12935,#12936,
#12937,#12938,#12939,#12940,#12941,#12942,#12943,#12944,#12945,#12946,#12947,
#12948,#12949,#12950,#12951,#12952,#12953,#12954,#12955,#12956,#12957,#12958,
#12959,#12960,#12961,#12962,#12963,#12964,#12965,#12966,#12967,#12968,#12969,
#12970,#12971,#12972,#12973,#12974,#12975,#12976,#12977,#12978,#12979,#12980,
#12981,#12982,#12983,#12984,#12985,#12986,#12987,#12988,#12989,#12990,#12991,
#12992,#12993,#12994,#12995,#12996,#12997,#12998,#12999));
#3338=EDGE_LOOP('',(#13000));
#3339=EDGE_LOOP('',(#13001));
#3340=EDGE_LOOP('',(#13002,#13003,#13004,#13005,#13006,#13007));
#3341=EDGE_LOOP('',(#13008,#13009,#13010));
#3342=EDGE_LOOP('',(#13011));
#3343=EDGE_LOOP('',(#13012,#13013,#13014,#13015,#13016));
#3344=EDGE_LOOP('',(#13017,#13018,#13019,#13020,#13021,#13022,#13023,#13024,
#13025,#13026,#13027,#13028,#13029,#13030,#13031,#13032,#13033,#13034,#13035,
#13036,#13037,#13038,#13039,#13040,#13041,#13042,#13043,#13044,#13045,#13046,
#13047,#13048,#13049,#13050,#13051,#13052,#13053,#13054,#13055,#13056,#13057,
#13058,#13059,#13060,#13061,#13062,#13063,#13064,#13065,#13066,#13067,#13068,
#13069,#13070,#13071,#13072,#13073,#13074,#13075,#13076,#13077,#13078,#13079,
#13080,#13081,#13082,#13083,#13084,#13085,#13086,#13087,#13088,#13089,#13090,
#13091,#13092,#13093,#13094,#13095,#13096,#13097,#13098,#13099,#13100,#13101,
#13102,#13103,#13104,#13105,#13106,#13107,#13108,#13109));
#3345=EDGE_LOOP('',(#13110));
#3346=EDGE_LOOP('',(#13111,#13112,#13113,#13114));
#4365=LINE('',#27588,#5589);
#4366=LINE('',#27612,#5590);
#4367=LINE('',#27660,#5591);
#4368=LINE('',#27708,#5592);
#4369=LINE('',#27762,#5593);
#4370=LINE('',#27810,#5594);
#4371=LINE('',#27858,#5595);
#4372=LINE('',#27906,#5596);
#4373=LINE('',#27957,#5597);
#4374=LINE('',#28005,#5598);
#4375=LINE('',#28053,#5599);
#4376=LINE('',#28107,#5600);
#4377=LINE('',#28155,#5601);
#4378=LINE('',#28203,#5602);
#4379=LINE('',#28257,#5603);
#4380=LINE('',#28305,#5604);
#4381=LINE('',#28353,#5605);
#4382=LINE('',#28407,#5606);
#4383=LINE('',#28455,#5607);
#4384=LINE('',#28503,#5608);
#4385=LINE('',#28557,#5609);
#4386=LINE('',#28605,#5610);
#4387=LINE('',#28653,#5611);
#4388=LINE('',#28704,#5612);
#4389=LINE('',#28754,#5613);
#4390=LINE('',#28775,#5614);
#4391=LINE('',#28799,#5615);
#4392=LINE('',#28824,#5616);
#4393=LINE('',#28848,#5617);
#4394=LINE('',#28873,#5618);
#4395=LINE('',#28898,#5619);
#4396=LINE('',#28922,#5620);
#4397=LINE('',#28947,#5621);
#4398=LINE('',#28972,#5622);
#4399=LINE('',#28996,#5623);
#4400=LINE('',#29021,#5624);
#4401=LINE('',#29046,#5625);
#4402=LINE('',#29070,#5626);
#4403=LINE('',#29095,#5627);
#4404=LINE('',#29120,#5628);
#4405=LINE('',#29144,#5629);
#4406=LINE('',#29169,#5630);
#4407=LINE('',#29193,#5631);
#4408=LINE('',#29218,#5632);
#4409=LINE('',#29242,#5633);
#4410=LINE('',#29267,#5634);
#4411=LINE('',#29292,#5635);
#4412=LINE('',#29316,#5636);
#4413=LINE('',#29318,#5637);
#4414=LINE('',#29320,#5638);
#4415=LINE('',#29321,#5639);
#4416=LINE('',#29324,#5640);
#4417=LINE('',#29326,#5641);
#4418=LINE('',#29327,#5642);
#4419=LINE('',#29330,#5643);
#4420=LINE('',#29332,#5644);
#4421=LINE('',#29333,#5645);
#4422=LINE('',#29335,#5646);
#4423=LINE('',#29336,#5647);
#4424=LINE('',#29342,#5648);
#4425=LINE('',#30818,#5649);
#4426=LINE('',#30823,#5650);
#4427=LINE('',#30830,#5651);
#4428=LINE('',#30841,#5652);
#4429=LINE('',#30846,#5653);
#4430=LINE('',#30853,#5654);
#4431=LINE('',#30864,#5655);
#4432=LINE('',#30869,#5656);
#4433=LINE('',#30876,#5657);
#4434=LINE('',#30887,#5658);
#4435=LINE('',#30892,#5659);
#4436=LINE('',#30899,#5660);
#4437=LINE('',#30910,#5661);
#4438=LINE('',#30915,#5662);
#4439=LINE('',#30922,#5663);
#4440=LINE('',#30933,#5664);
#4441=LINE('',#30938,#5665);
#4442=LINE('',#30945,#5666);
#4443=LINE('',#30956,#5667);
#4444=LINE('',#30961,#5668);
#4445=LINE('',#30968,#5669);
#4446=LINE('',#30979,#5670);
#4447=LINE('',#30984,#5671);
#4448=LINE('',#30991,#5672);
#4449=LINE('',#31002,#5673);
#4450=LINE('',#31007,#5674);
#4451=LINE('',#31014,#5675);
#4452=LINE('',#31025,#5676);
#4453=LINE('',#31030,#5677);
#4454=LINE('',#31037,#5678);
#4455=LINE('',#31048,#5679);
#4456=LINE('',#31053,#5680);
#4457=LINE('',#31060,#5681);
#4458=LINE('',#31071,#5682);
#4459=LINE('',#31076,#5683);
#4460=LINE('',#31083,#5684);
#4461=LINE('',#31094,#5685);
#4462=LINE('',#31099,#5686);
#4463=LINE('',#31106,#5687);
#4464=LINE('',#31117,#5688);
#4465=LINE('',#31122,#5689);
#4466=LINE('',#31129,#5690);
#4467=LINE('',#31140,#5691);
#4468=LINE('',#31145,#5692);
#4469=LINE('',#31152,#5693);
#4470=LINE('',#31163,#5694);
#4471=LINE('',#31168,#5695);
#4472=LINE('',#31175,#5696);
#4473=LINE('',#31186,#5697);
#4474=LINE('',#31191,#5698);
#4475=LINE('',#31198,#5699);
#4476=LINE('',#31209,#5700);
#4477=LINE('',#31214,#5701);
#4478=LINE('',#31221,#5702);
#4479=LINE('',#31232,#5703);
#4480=LINE('',#31237,#5704);
#4481=LINE('',#31244,#5705);
#4482=LINE('',#31255,#5706);
#4483=LINE('',#31260,#5707);
#4484=LINE('',#31267,#5708);
#4485=LINE('',#31278,#5709);
#4486=LINE('',#31283,#5710);
#4487=LINE('',#31290,#5711);
#4488=LINE('',#31301,#5712);
#4489=LINE('',#31306,#5713);
#4490=LINE('',#31313,#5714);
#4491=LINE('',#31324,#5715);
#4492=LINE('',#31329,#5716);
#4493=LINE('',#31336,#5717);
#4494=LINE('',#31347,#5718);
#4495=LINE('',#31352,#5719);
#4496=LINE('',#31359,#5720);
#4497=LINE('',#31370,#5721);
#4498=LINE('',#31375,#5722);
#4499=LINE('',#31382,#5723);
#4500=LINE('',#31393,#5724);
#4501=LINE('',#31398,#5725);
#4502=LINE('',#31405,#5726);
#4503=LINE('',#31416,#5727);
#4504=LINE('',#31421,#5728);
#4505=LINE('',#31428,#5729);
#4506=LINE('',#31439,#5730);
#4507=LINE('',#31444,#5731);
#4508=LINE('',#31451,#5732);
#4509=LINE('',#31462,#5733);
#4510=LINE('',#31467,#5734);
#4511=LINE('',#31474,#5735);
#4512=LINE('',#31485,#5736);
#4513=LINE('',#31490,#5737);
#4514=LINE('',#31497,#5738);
#4515=LINE('',#31593,#5739);
#4516=LINE('',#31599,#5740);
#4517=LINE('',#31606,#5741);
#5589=VECTOR('',#19910,0.25);
#5590=VECTOR('',#19915,0.25);
#5591=VECTOR('',#19918,0.25);
#5592=VECTOR('',#19921,0.25);
#5593=VECTOR('',#19924,0.25);
#5594=VECTOR('',#19927,0.25);
#5595=VECTOR('',#19930,0.25);
#5596=VECTOR('',#19933,0.25);
#5597=VECTOR('',#19936,0.25);
#5598=VECTOR('',#19939,0.25);
#5599=VECTOR('',#19942,0.25);
#5600=VECTOR('',#19945,0.25);
#5601=VECTOR('',#19948,0.25);
#5602=VECTOR('',#19951,0.25);
#5603=VECTOR('',#19954,0.25);
#5604=VECTOR('',#19957,0.25);
#5605=VECTOR('',#19960,0.25);
#5606=VECTOR('',#19963,0.25);
#5607=VECTOR('',#19966,0.25);
#5608=VECTOR('',#19969,0.25);
#5609=VECTOR('',#19972,0.25);
#5610=VECTOR('',#19975,0.25);
#5611=VECTOR('',#19978,0.25);
#5612=VECTOR('',#19981,0.25);
#5613=VECTOR('',#19986,0.217775);
#5614=VECTOR('',#19991,0.217775);
#5615=VECTOR('',#19994,0.217775);
#5616=VECTOR('',#19997,0.217775);
#5617=VECTOR('',#20000,0.217775);
#5618=VECTOR('',#20003,0.217775);
#5619=VECTOR('',#20006,0.217775);
#5620=VECTOR('',#20009,0.217775);
#5621=VECTOR('',#20012,0.217775);
#5622=VECTOR('',#20015,0.217775);
#5623=VECTOR('',#20018,0.217775);
#5624=VECTOR('',#20021,0.217775);
#5625=VECTOR('',#20024,0.217775);
#5626=VECTOR('',#20027,0.217775);
#5627=VECTOR('',#20030,0.217775);
#5628=VECTOR('',#20033,0.217775);
#5629=VECTOR('',#20036,0.217775);
#5630=VECTOR('',#20039,0.217775);
#5631=VECTOR('',#20042,0.217775);
#5632=VECTOR('',#20045,0.217775);
#5633=VECTOR('',#20048,0.217775);
#5634=VECTOR('',#20051,0.217775);
#5635=VECTOR('',#20054,0.217775);
#5636=VECTOR('',#20057,1.);
#5637=VECTOR('',#20058,1.);
#5638=VECTOR('',#20059,1.);
#5639=VECTOR('',#20060,1.);
#5640=VECTOR('',#20063,1.);
#5641=VECTOR('',#20064,1.);
#5642=VECTOR('',#20065,1.);
#5643=VECTOR('',#20068,1.);
#5644=VECTOR('',#20069,1.);
#5645=VECTOR('',#20070,1.);
#5646=VECTOR('',#20073,1.);
#5647=VECTOR('',#20074,1.);
#5648=VECTOR('',#20081,0.151);
#5649=VECTOR('',#20098,1.);
#5650=VECTOR('',#20099,1.);
#5651=VECTOR('',#20102,1.);
#5652=VECTOR('',#20105,1.);
#5653=VECTOR('',#20106,1.);
#5654=VECTOR('',#20109,1.);
#5655=VECTOR('',#20112,1.);
#5656=VECTOR('',#20113,1.);
#5657=VECTOR('',#20116,1.);
#5658=VECTOR('',#20119,1.);
#5659=VECTOR('',#20120,1.);
#5660=VECTOR('',#20123,1.);
#5661=VECTOR('',#20126,1.);
#5662=VECTOR('',#20127,1.);
#5663=VECTOR('',#20130,1.);
#5664=VECTOR('',#20133,1.);
#5665=VECTOR('',#20134,1.);
#5666=VECTOR('',#20137,1.);
#5667=VECTOR('',#20140,1.);
#5668=VECTOR('',#20141,1.);
#5669=VECTOR('',#20144,1.);
#5670=VECTOR('',#20147,1.);
#5671=VECTOR('',#20148,1.);
#5672=VECTOR('',#20151,1.);
#5673=VECTOR('',#20154,1.);
#5674=VECTOR('',#20155,1.);
#5675=VECTOR('',#20158,1.);
#5676=VECTOR('',#20161,1.);
#5677=VECTOR('',#20162,1.);
#5678=VECTOR('',#20165,1.);
#5679=VECTOR('',#20168,1.);
#5680=VECTOR('',#20169,1.);
#5681=VECTOR('',#20172,1.);
#5682=VECTOR('',#20175,1.);
#5683=VECTOR('',#20176,1.);
#5684=VECTOR('',#20179,1.);
#5685=VECTOR('',#20182,1.);
#5686=VECTOR('',#20183,1.);
#5687=VECTOR('',#20186,1.);
#5688=VECTOR('',#20189,1.);
#5689=VECTOR('',#20190,1.);
#5690=VECTOR('',#20193,1.);
#5691=VECTOR('',#20196,1.);
#5692=VECTOR('',#20197,1.);
#5693=VECTOR('',#20200,1.);
#5694=VECTOR('',#20203,1.);
#5695=VECTOR('',#20204,1.);
#5696=VECTOR('',#20207,1.);
#5697=VECTOR('',#20210,1.);
#5698=VECTOR('',#20211,1.);
#5699=VECTOR('',#20214,1.);
#5700=VECTOR('',#20217,1.);
#5701=VECTOR('',#20218,1.);
#5702=VECTOR('',#20221,1.);
#5703=VECTOR('',#20224,1.);
#5704=VECTOR('',#20225,1.);
#5705=VECTOR('',#20228,1.);
#5706=VECTOR('',#20231,1.);
#5707=VECTOR('',#20232,1.);
#5708=VECTOR('',#20235,1.);
#5709=VECTOR('',#20238,1.);
#5710=VECTOR('',#20239,1.);
#5711=VECTOR('',#20242,1.);
#5712=VECTOR('',#20245,1.);
#5713=VECTOR('',#20246,1.);
#5714=VECTOR('',#20249,1.);
#5715=VECTOR('',#20252,1.);
#5716=VECTOR('',#20253,1.);
#5717=VECTOR('',#20256,1.);
#5718=VECTOR('',#20259,1.);
#5719=VECTOR('',#20260,1.);
#5720=VECTOR('',#20263,1.);
#5721=VECTOR('',#20266,1.);
#5722=VECTOR('',#20267,1.);
#5723=VECTOR('',#20270,1.);
#5724=VECTOR('',#20273,1.);
#5725=VECTOR('',#20274,1.);
#5726=VECTOR('',#20277,1.);
#5727=VECTOR('',#20280,1.);
#5728=VECTOR('',#20281,1.);
#5729=VECTOR('',#20284,1.);
#5730=VECTOR('',#20287,1.);
#5731=VECTOR('',#20288,1.);
#5732=VECTOR('',#20291,1.);
#5733=VECTOR('',#20294,1.);
#5734=VECTOR('',#20295,1.);
#5735=VECTOR('',#20298,1.);
#5736=VECTOR('',#20301,1.);
#5737=VECTOR('',#20302,1.);
#5738=VECTOR('',#20305,1.);
#5739=VECTOR('',#20488,0.475);
#5740=VECTOR('',#20497,0.23);
#5741=VECTOR('',#20508,0.47);
#6776=VERTEX_POINT('',#27586);
#6777=VERTEX_POINT('',#27587);
#6778=VERTEX_POINT('',#27589);
#6779=VERTEX_POINT('',#27600);
#6780=VERTEX_POINT('',#27610);
#6781=VERTEX_POINT('',#27611);
#6782=VERTEX_POINT('',#27658);
#6783=VERTEX_POINT('',#27659);
#6784=VERTEX_POINT('',#27706);
#6785=VERTEX_POINT('',#27707);
#6786=VERTEX_POINT('',#27760);
#6787=VERTEX_POINT('',#27761);
#6788=VERTEX_POINT('',#27808);
#6789=VERTEX_POINT('',#27809);
#6790=VERTEX_POINT('',#27856);
#6791=VERTEX_POINT('',#27857);
#6792=VERTEX_POINT('',#27904);
#6793=VERTEX_POINT('',#27905);
#6794=VERTEX_POINT('',#27955);
#6795=VERTEX_POINT('',#27956);
#6796=VERTEX_POINT('',#28003);
#6797=VERTEX_POINT('',#28004);
#6798=VERTEX_POINT('',#28051);
#6799=VERTEX_POINT('',#28052);
#6800=VERTEX_POINT('',#28105);
#6801=VERTEX_POINT('',#28106);
#6802=VERTEX_POINT('',#28153);
#6803=VERTEX_POINT('',#28154);
#6804=VERTEX_POINT('',#28201);
#6805=VERTEX_POINT('',#28202);
#6806=VERTEX_POINT('',#28255);
#6807=VERTEX_POINT('',#28256);
#6808=VERTEX_POINT('',#28303);
#6809=VERTEX_POINT('',#28304);
#6810=VERTEX_POINT('',#28351);
#6811=VERTEX_POINT('',#28352);
#6812=VERTEX_POINT('',#28405);
#6813=VERTEX_POINT('',#28406);
#6814=VERTEX_POINT('',#28453);
#6815=VERTEX_POINT('',#28454);
#6816=VERTEX_POINT('',#28501);
#6817=VERTEX_POINT('',#28502);
#6818=VERTEX_POINT('',#28555);
#6819=VERTEX_POINT('',#28556);
#6820=VERTEX_POINT('',#28603);
#6821=VERTEX_POINT('',#28604);
#6822=VERTEX_POINT('',#28651);
#6823=VERTEX_POINT('',#28652);
#6824=VERTEX_POINT('',#28702);
#6825=VERTEX_POINT('',#28703);
#6826=VERTEX_POINT('',#28705);
#6827=VERTEX_POINT('',#28752);
#6828=VERTEX_POINT('',#28753);
#6829=VERTEX_POINT('',#28755);
#6830=VERTEX_POINT('',#28764);
#6831=VERTEX_POINT('',#28773);
#6832=VERTEX_POINT('',#28774);
#6833=VERTEX_POINT('',#28797);
#6834=VERTEX_POINT('',#28798);
#6835=VERTEX_POINT('',#28822);
#6836=VERTEX_POINT('',#28823);
#6837=VERTEX_POINT('',#28846);
#6838=VERTEX_POINT('',#28847);
#6839=VERTEX_POINT('',#28871);
#6840=VERTEX_POINT('',#28872);
#6841=VERTEX_POINT('',#28896);
#6842=VERTEX_POINT('',#28897);
#6843=VERTEX_POINT('',#28920);
#6844=VERTEX_POINT('',#28921);
#6845=VERTEX_POINT('',#28945);
#6846=VERTEX_POINT('',#28946);
#6847=VERTEX_POINT('',#28970);
#6848=VERTEX_POINT('',#28971);
#6849=VERTEX_POINT('',#28994);
#6850=VERTEX_POINT('',#28995);
#6851=VERTEX_POINT('',#29019);
#6852=VERTEX_POINT('',#29020);
#6853=VERTEX_POINT('',#29044);
#6854=VERTEX_POINT('',#29045);
#6855=VERTEX_POINT('',#29068);
#6856=VERTEX_POINT('',#29069);
#6857=VERTEX_POINT('',#29093);
#6858=VERTEX_POINT('',#29094);
#6859=VERTEX_POINT('',#29118);
#6860=VERTEX_POINT('',#29119);
#6861=VERTEX_POINT('',#29142);
#6862=VERTEX_POINT('',#29143);
#6863=VERTEX_POINT('',#29167);
#6864=VERTEX_POINT('',#29168);
#6865=VERTEX_POINT('',#29191);
#6866=VERTEX_POINT('',#29192);
#6867=VERTEX_POINT('',#29216);
#6868=VERTEX_POINT('',#29217);
#6869=VERTEX_POINT('',#29240);
#6870=VERTEX_POINT('',#29241);
#6871=VERTEX_POINT('',#29265);
#6872=VERTEX_POINT('',#29266);
#6873=VERTEX_POINT('',#29290);
#6874=VERTEX_POINT('',#29291);
#6875=VERTEX_POINT('',#29314);
#6876=VERTEX_POINT('',#29315);
#6877=VERTEX_POINT('',#29317);
#6878=VERTEX_POINT('',#29319);
#6879=VERTEX_POINT('',#29323);
#6880=VERTEX_POINT('',#29325);
#6881=VERTEX_POINT('',#29329);
#6882=VERTEX_POINT('',#29331);
#6883=VERTEX_POINT('',#29339);
#6884=VERTEX_POINT('',#29341);
#6885=VERTEX_POINT('',#29953);
#6886=VERTEX_POINT('',#30013);
#6887=VERTEX_POINT('',#30079);
#6888=VERTEX_POINT('',#30082);
#6889=VERTEX_POINT('',#30812);
#6890=VERTEX_POINT('',#30813);
#6891=VERTEX_POINT('',#30817);
#6892=VERTEX_POINT('',#30819);
#6893=VERTEX_POINT('',#30825);
#6894=VERTEX_POINT('',#30829);
#6895=VERTEX_POINT('',#30835);
#6896=VERTEX_POINT('',#30836);
#6897=VERTEX_POINT('',#30840);
#6898=VERTEX_POINT('',#30842);
#6899=VERTEX_POINT('',#30848);
#6900=VERTEX_POINT('',#30852);
#6901=VERTEX_POINT('',#30858);
#6902=VERTEX_POINT('',#30859);
#6903=VERTEX_POINT('',#30863);
#6904=VERTEX_POINT('',#30865);
#6905=VERTEX_POINT('',#30871);
#6906=VERTEX_POINT('',#30875);
#6907=VERTEX_POINT('',#30881);
#6908=VERTEX_POINT('',#30882);
#6909=VERTEX_POINT('',#30886);
#6910=VERTEX_POINT('',#30888);
#6911=VERTEX_POINT('',#30894);
#6912=VERTEX_POINT('',#30898);
#6913=VERTEX_POINT('',#30904);
#6914=VERTEX_POINT('',#30905);
#6915=VERTEX_POINT('',#30909);
#6916=VERTEX_POINT('',#30911);
#6917=VERTEX_POINT('',#30917);
#6918=VERTEX_POINT('',#30921);
#6919=VERTEX_POINT('',#30927);
#6920=VERTEX_POINT('',#30928);
#6921=VERTEX_POINT('',#30932);
#6922=VERTEX_POINT('',#30934);
#6923=VERTEX_POINT('',#30940);
#6924=VERTEX_POINT('',#30944);
#6925=VERTEX_POINT('',#30950);
#6926=VERTEX_POINT('',#30951);
#6927=VERTEX_POINT('',#30955);
#6928=VERTEX_POINT('',#30957);
#6929=VERTEX_POINT('',#30963);
#6930=VERTEX_POINT('',#30967);
#6931=VERTEX_POINT('',#30973);
#6932=VERTEX_POINT('',#30974);
#6933=VERTEX_POINT('',#30978);
#6934=VERTEX_POINT('',#30980);
#6935=VERTEX_POINT('',#30986);
#6936=VERTEX_POINT('',#30990);
#6937=VERTEX_POINT('',#30996);
#6938=VERTEX_POINT('',#30997);
#6939=VERTEX_POINT('',#31001);
#6940=VERTEX_POINT('',#31003);
#6941=VERTEX_POINT('',#31009);
#6942=VERTEX_POINT('',#31013);
#6943=VERTEX_POINT('',#31019);
#6944=VERTEX_POINT('',#31020);
#6945=VERTEX_POINT('',#31024);
#6946=VERTEX_POINT('',#31026);
#6947=VERTEX_POINT('',#31032);
#6948=VERTEX_POINT('',#31036);
#6949=VERTEX_POINT('',#31042);
#6950=VERTEX_POINT('',#31043);
#6951=VERTEX_POINT('',#31047);
#6952=VERTEX_POINT('',#31049);
#6953=VERTEX_POINT('',#31055);
#6954=VERTEX_POINT('',#31059);
#6955=VERTEX_POINT('',#31065);
#6956=VERTEX_POINT('',#31066);
#6957=VERTEX_POINT('',#31070);
#6958=VERTEX_POINT('',#31072);
#6959=VERTEX_POINT('',#31078);
#6960=VERTEX_POINT('',#31082);
#6961=VERTEX_POINT('',#31088);
#6962=VERTEX_POINT('',#31089);
#6963=VERTEX_POINT('',#31093);
#6964=VERTEX_POINT('',#31095);
#6965=VERTEX_POINT('',#31101);
#6966=VERTEX_POINT('',#31105);
#6967=VERTEX_POINT('',#31111);
#6968=VERTEX_POINT('',#31112);
#6969=VERTEX_POINT('',#31116);
#6970=VERTEX_POINT('',#31118);
#6971=VERTEX_POINT('',#31124);
#6972=VERTEX_POINT('',#31128);
#6973=VERTEX_POINT('',#31134);
#6974=VERTEX_POINT('',#31135);
#6975=VERTEX_POINT('',#31139);
#6976=VERTEX_POINT('',#31141);
#6977=VERTEX_POINT('',#31147);
#6978=VERTEX_POINT('',#31151);
#6979=VERTEX_POINT('',#31157);
#6980=VERTEX_POINT('',#31158);
#6981=VERTEX_POINT('',#31162);
#6982=VERTEX_POINT('',#31164);
#6983=VERTEX_POINT('',#31170);
#6984=VERTEX_POINT('',#31174);
#6985=VERTEX_POINT('',#31180);
#6986=VERTEX_POINT('',#31181);
#6987=VERTEX_POINT('',#31185);
#6988=VERTEX_POINT('',#31187);
#6989=VERTEX_POINT('',#31193);
#6990=VERTEX_POINT('',#31197);
#6991=VERTEX_POINT('',#31203);
#6992=VERTEX_POINT('',#31204);
#6993=VERTEX_POINT('',#31208);
#6994=VERTEX_POINT('',#31210);
#6995=VERTEX_POINT('',#31216);
#6996=VERTEX_POINT('',#31220);
#6997=VERTEX_POINT('',#31226);
#6998=VERTEX_POINT('',#31227);
#6999=VERTEX_POINT('',#31231);
#7000=VERTEX_POINT('',#31233);
#7001=VERTEX_POINT('',#31239);
#7002=VERTEX_POINT('',#31243);
#7003=VERTEX_POINT('',#31249);
#7004=VERTEX_POINT('',#31250);
#7005=VERTEX_POINT('',#31254);
#7006=VERTEX_POINT('',#31256);
#7007=VERTEX_POINT('',#31262);
#7008=VERTEX_POINT('',#31266);
#7009=VERTEX_POINT('',#31272);
#7010=VERTEX_POINT('',#31273);
#7011=VERTEX_POINT('',#31277);
#7012=VERTEX_POINT('',#31279);
#7013=VERTEX_POINT('',#31285);
#7014=VERTEX_POINT('',#31289);
#7015=VERTEX_POINT('',#31295);
#7016=VERTEX_POINT('',#31296);
#7017=VERTEX_POINT('',#31300);
#7018=VERTEX_POINT('',#31302);
#7019=VERTEX_POINT('',#31308);
#7020=VERTEX_POINT('',#31312);
#7021=VERTEX_POINT('',#31318);
#7022=VERTEX_POINT('',#31319);
#7023=VERTEX_POINT('',#31323);
#7024=VERTEX_POINT('',#31325);
#7025=VERTEX_POINT('',#31331);
#7026=VERTEX_POINT('',#31335);
#7027=VERTEX_POINT('',#31341);
#7028=VERTEX_POINT('',#31342);
#7029=VERTEX_POINT('',#31346);
#7030=VERTEX_POINT('',#31348);
#7031=VERTEX_POINT('',#31354);
#7032=VERTEX_POINT('',#31358);
#7033=VERTEX_POINT('',#31364);
#7034=VERTEX_POINT('',#31365);
#7035=VERTEX_POINT('',#31369);
#7036=VERTEX_POINT('',#31371);
#7037=VERTEX_POINT('',#31377);
#7038=VERTEX_POINT('',#31381);
#7039=VERTEX_POINT('',#31387);
#7040=VERTEX_POINT('',#31388);
#7041=VERTEX_POINT('',#31392);
#7042=VERTEX_POINT('',#31394);
#7043=VERTEX_POINT('',#31400);
#7044=VERTEX_POINT('',#31404);
#7045=VERTEX_POINT('',#31410);
#7046=VERTEX_POINT('',#31411);
#7047=VERTEX_POINT('',#31415);
#7048=VERTEX_POINT('',#31417);
#7049=VERTEX_POINT('',#31423);
#7050=VERTEX_POINT('',#31427);
#7051=VERTEX_POINT('',#31433);
#7052=VERTEX_POINT('',#31434);
#7053=VERTEX_POINT('',#31438);
#7054=VERTEX_POINT('',#31440);
#7055=VERTEX_POINT('',#31446);
#7056=VERTEX_POINT('',#31450);
#7057=VERTEX_POINT('',#31456);
#7058=VERTEX_POINT('',#31457);
#7059=VERTEX_POINT('',#31461);
#7060=VERTEX_POINT('',#31463);
#7061=VERTEX_POINT('',#31469);
#7062=VERTEX_POINT('',#31473);
#7063=VERTEX_POINT('',#31479);
#7064=VERTEX_POINT('',#31480);
#7065=VERTEX_POINT('',#31484);
#7066=VERTEX_POINT('',#31486);
#7067=VERTEX_POINT('',#31492);
#7068=VERTEX_POINT('',#31496);
#7069=VERTEX_POINT('',#31592);
#7070=VERTEX_POINT('',#31596);
#7071=VERTEX_POINT('',#31604);
#8727=EDGE_CURVE('',#6776,#6777,#4365,.T.);
#8728=EDGE_CURVE('',#6776,#6778,#627,.T.);
#8729=EDGE_CURVE('',#6778,#6779,#1443,.T.);
#8730=EDGE_CURVE('',#6779,#6777,#628,.T.);
#8731=EDGE_CURVE('',#6780,#6781,#4366,.T.);
#8732=EDGE_CURVE('',#6780,#6776,#629,.T.);
#8733=EDGE_CURVE('',#6777,#6781,#630,.T.);
#8734=EDGE_CURVE('',#6782,#6783,#4367,.T.);
#8735=EDGE_CURVE('',#6782,#6780,#631,.T.);
#8736=EDGE_CURVE('',#6781,#6783,#632,.T.);
#8737=EDGE_CURVE('',#6784,#6785,#4368,.T.);
#8738=EDGE_CURVE('',#6784,#6782,#633,.T.);
#8739=EDGE_CURVE('',#6783,#6785,#634,.T.);
#8740=EDGE_CURVE('',#6786,#6787,#4369,.T.);
#8741=EDGE_CURVE('',#6786,#6784,#635,.T.);
#8742=EDGE_CURVE('',#6785,#6787,#636,.T.);
#8743=EDGE_CURVE('',#6788,#6789,#4370,.T.);
#8744=EDGE_CURVE('',#6788,#6786,#637,.T.);
#8745=EDGE_CURVE('',#6787,#6789,#638,.T.);
#8746=EDGE_CURVE('',#6790,#6791,#4371,.T.);
#8747=EDGE_CURVE('',#6790,#6788,#639,.T.);
#8748=EDGE_CURVE('',#6789,#6791,#640,.T.);
#8749=EDGE_CURVE('',#6792,#6793,#4372,.T.);
#8750=EDGE_CURVE('',#6792,#6790,#641,.T.);
#8751=EDGE_CURVE('',#6791,#6793,#642,.T.);
#8752=EDGE_CURVE('',#6794,#6795,#4373,.T.);
#8753=EDGE_CURVE('',#6794,#6792,#643,.T.);
#8754=EDGE_CURVE('',#6793,#6795,#644,.T.);
#8755=EDGE_CURVE('',#6796,#6797,#4374,.T.);
#8756=EDGE_CURVE('',#6796,#6794,#645,.T.);
#8757=EDGE_CURVE('',#6795,#6797,#646,.T.);
#8758=EDGE_CURVE('',#6798,#6799,#4375,.T.);
#8759=EDGE_CURVE('',#6798,#6796,#647,.T.);
#8760=EDGE_CURVE('',#6797,#6799,#648,.T.);
#8761=EDGE_CURVE('',#6800,#6801,#4376,.T.);
#8762=EDGE_CURVE('',#6800,#6798,#649,.T.);
#8763=EDGE_CURVE('',#6799,#6801,#650,.T.);
#8764=EDGE_CURVE('',#6802,#6803,#4377,.T.);
#8765=EDGE_CURVE('',#6802,#6800,#651,.T.);
#8766=EDGE_CURVE('',#6801,#6803,#652,.T.);
#8767=EDGE_CURVE('',#6804,#6805,#4378,.T.);
#8768=EDGE_CURVE('',#6804,#6802,#653,.T.);
#8769=EDGE_CURVE('',#6803,#6805,#654,.T.);
#8770=EDGE_CURVE('',#6806,#6807,#4379,.T.);
#8771=EDGE_CURVE('',#6806,#6804,#655,.T.);
#8772=EDGE_CURVE('',#6805,#6807,#656,.T.);
#8773=EDGE_CURVE('',#6808,#6809,#4380,.T.);
#8774=EDGE_CURVE('',#6808,#6806,#657,.T.);
#8775=EDGE_CURVE('',#6807,#6809,#658,.T.);
#8776=EDGE_CURVE('',#6810,#6811,#4381,.T.);
#8777=EDGE_CURVE('',#6810,#6808,#659,.T.);
#8778=EDGE_CURVE('',#6809,#6811,#660,.T.);
#8779=EDGE_CURVE('',#6812,#6813,#4382,.T.);
#8780=EDGE_CURVE('',#6812,#6810,#661,.T.);
#8781=EDGE_CURVE('',#6811,#6813,#662,.T.);
#8782=EDGE_CURVE('',#6814,#6815,#4383,.T.);
#8783=EDGE_CURVE('',#6814,#6812,#663,.T.);
#8784=EDGE_CURVE('',#6813,#6815,#664,.T.);
#8785=EDGE_CURVE('',#6816,#6817,#4384,.T.);
#8786=EDGE_CURVE('',#6816,#6814,#665,.T.);
#8787=EDGE_CURVE('',#6815,#6817,#666,.T.);
#8788=EDGE_CURVE('',#6818,#6819,#4385,.T.);
#8789=EDGE_CURVE('',#6818,#6816,#667,.T.);
#8790=EDGE_CURVE('',#6817,#6819,#668,.T.);
#8791=EDGE_CURVE('',#6820,#6821,#4386,.T.);
#8792=EDGE_CURVE('',#6820,#6818,#669,.T.);
#8793=EDGE_CURVE('',#6819,#6821,#670,.T.);
#8794=EDGE_CURVE('',#6822,#6823,#4387,.T.);
#8795=EDGE_CURVE('',#6822,#6820,#671,.T.);
#8796=EDGE_CURVE('',#6821,#6823,#672,.T.);
#8797=EDGE_CURVE('',#6824,#6825,#4388,.T.);
#8798=EDGE_CURVE('',#6826,#6824,#1444,.T.);
#8799=EDGE_CURVE('',#6826,#6822,#673,.T.);
#8800=EDGE_CURVE('',#6823,#6825,#674,.T.);
#8801=EDGE_CURVE('',#6827,#6828,#4389,.T.);
#8802=EDGE_CURVE('',#6827,#6829,#675,.T.);
#8803=EDGE_CURVE('',#6830,#6829,#1445,.T.);
#8804=EDGE_CURVE('',#6828,#6830,#676,.T.);
#8805=EDGE_CURVE('',#6831,#6832,#4390,.T.);
#8806=EDGE_CURVE('',#6831,#6827,#677,.T.);
#8807=EDGE_CURVE('',#6832,#6828,#678,.T.);
#8808=EDGE_CURVE('',#6833,#6834,#4391,.T.);
#8809=EDGE_CURVE('',#6833,#6831,#679,.T.);
#8810=EDGE_CURVE('',#6834,#6832,#680,.T.);
#8811=EDGE_CURVE('',#6835,#6836,#4392,.T.);
#8812=EDGE_CURVE('',#6835,#6833,#681,.T.);
#8813=EDGE_CURVE('',#6836,#6834,#682,.T.);
#8814=EDGE_CURVE('',#6837,#6838,#4393,.T.);
#8815=EDGE_CURVE('',#6837,#6835,#683,.T.);
#8816=EDGE_CURVE('',#6838,#6836,#684,.T.);
#8817=EDGE_CURVE('',#6839,#6840,#4394,.T.);
#8818=EDGE_CURVE('',#6839,#6837,#685,.T.);
#8819=EDGE_CURVE('',#6840,#6838,#686,.T.);
#8820=EDGE_CURVE('',#6841,#6842,#4395,.T.);
#8821=EDGE_CURVE('',#6841,#6839,#687,.T.);
#8822=EDGE_CURVE('',#6842,#6840,#688,.T.);
#8823=EDGE_CURVE('',#6843,#6844,#4396,.T.);
#8824=EDGE_CURVE('',#6843,#6841,#689,.T.);
#8825=EDGE_CURVE('',#6844,#6842,#690,.T.);
#8826=EDGE_CURVE('',#6845,#6846,#4397,.T.);
#8827=EDGE_CURVE('',#6845,#6843,#691,.T.);
#8828=EDGE_CURVE('',#6846,#6844,#692,.T.);
#8829=EDGE_CURVE('',#6847,#6848,#4398,.T.);
#8830=EDGE_CURVE('',#6847,#6845,#693,.T.);
#8831=EDGE_CURVE('',#6848,#6846,#694,.T.);
#8832=EDGE_CURVE('',#6849,#6850,#4399,.T.);
#8833=EDGE_CURVE('',#6849,#6847,#695,.T.);
#8834=EDGE_CURVE('',#6850,#6848,#696,.T.);
#8835=EDGE_CURVE('',#6851,#6852,#4400,.T.);
#8836=EDGE_CURVE('',#6851,#6849,#697,.T.);
#8837=EDGE_CURVE('',#6852,#6850,#698,.T.);
#8838=EDGE_CURVE('',#6853,#6854,#4401,.T.);
#8839=EDGE_CURVE('',#6853,#6851,#699,.T.);
#8840=EDGE_CURVE('',#6854,#6852,#700,.T.);
#8841=EDGE_CURVE('',#6855,#6856,#4402,.T.);
#8842=EDGE_CURVE('',#6855,#6853,#701,.T.);
#8843=EDGE_CURVE('',#6856,#6854,#702,.T.);
#8844=EDGE_CURVE('',#6857,#6858,#4403,.T.);
#8845=EDGE_CURVE('',#6857,#6855,#703,.T.);
#8846=EDGE_CURVE('',#6858,#6856,#704,.T.);
#8847=EDGE_CURVE('',#6859,#6860,#4404,.T.);
#8848=EDGE_CURVE('',#6859,#6857,#705,.T.);
#8849=EDGE_CURVE('',#6860,#6858,#706,.T.);
#8850=EDGE_CURVE('',#6861,#6862,#4405,.T.);
#8851=EDGE_CURVE('',#6861,#6859,#707,.T.);
#8852=EDGE_CURVE('',#6862,#6860,#708,.T.);
#8853=EDGE_CURVE('',#6863,#6864,#4406,.T.);
#8854=EDGE_CURVE('',#6863,#6861,#709,.T.);
#8855=EDGE_CURVE('',#6864,#6862,#710,.T.);
#8856=EDGE_CURVE('',#6865,#6866,#4407,.T.);
#8857=EDGE_CURVE('',#6865,#6863,#711,.T.);
#8858=EDGE_CURVE('',#6866,#6864,#712,.T.);
#8859=EDGE_CURVE('',#6867,#6868,#4408,.T.);
#8860=EDGE_CURVE('',#6867,#6865,#713,.T.);
#8861=EDGE_CURVE('',#6868,#6866,#714,.T.);
#8862=EDGE_CURVE('',#6869,#6870,#4409,.T.);
#8863=EDGE_CURVE('',#6869,#6867,#715,.T.);
#8864=EDGE_CURVE('',#6870,#6868,#716,.T.);
#8865=EDGE_CURVE('',#6871,#6872,#4410,.T.);
#8866=EDGE_CURVE('',#6871,#6869,#717,.T.);
#8867=EDGE_CURVE('',#6872,#6870,#718,.T.);
#8868=EDGE_CURVE('',#6873,#6874,#4411,.T.);
#8869=EDGE_CURVE('',#6873,#6871,#719,.T.);
#8870=EDGE_CURVE('',#6874,#6872,#720,.T.);
#8871=EDGE_CURVE('',#6875,#6876,#4412,.T.);
#8872=EDGE_CURVE('',#6875,#6877,#4413,.T.);
#8873=EDGE_CURVE('',#6877,#6878,#4414,.T.);
#8874=EDGE_CURVE('',#6876,#6878,#4415,.T.);
#8875=EDGE_CURVE('',#6879,#6875,#4416,.T.);
#8876=EDGE_CURVE('',#6879,#6880,#4417,.T.);
#8877=EDGE_CURVE('',#6880,#6877,#4418,.T.);
#8878=EDGE_CURVE('',#6881,#6879,#4419,.T.);
#8879=EDGE_CURVE('',#6881,#6882,#4420,.T.);
#8880=EDGE_CURVE('',#6882,#6880,#4421,.T.);
#8881=EDGE_CURVE('',#6876,#6881,#4422,.T.);
#8882=EDGE_CURVE('',#6878,#6882,#4423,.T.);
#8883=EDGE_CURVE('',#6883,#6883,#1446,.T.);
#8884=EDGE_CURVE('',#6883,#6884,#4424,.T.);
#8885=EDGE_CURVE('',#6884,#6884,#1447,.T.);
#8886=EDGE_CURVE('',#6885,#6830,#721,.T.);
#8887=EDGE_CURVE('',#6825,#6885,#722,.T.);
#8888=EDGE_CURVE('',#6886,#6779,#723,.T.);
#8889=EDGE_CURVE('',#6886,#6874,#724,.T.);
#8890=EDGE_CURVE('',#6779,#6887,#1448,.T.);
#8891=EDGE_CURVE('',#6887,#6778,#1449,.T.);
#8892=EDGE_CURVE('',#6778,#6888,#725,.T.);
#8893=EDGE_CURVE('',#6888,#6886,#1450,.T.);
#8894=EDGE_CURVE('',#6888,#6873,#726,.T.);
#8895=EDGE_CURVE('',#6829,#6826,#727,.T.);
#8896=EDGE_CURVE('',#6889,#6890,#132,.T.);
#8897=EDGE_CURVE('',#6889,#6891,#4425,.T.);
#8898=EDGE_CURVE('',#6892,#6891,#133,.T.);
#8899=EDGE_CURVE('',#6890,#6892,#4426,.T.);
#8900=EDGE_CURVE('',#6893,#6889,#134,.T.);
#8901=EDGE_CURVE('',#6894,#6893,#4427,.T.);
#8902=EDGE_CURVE('',#6891,#6894,#135,.T.);
#8903=EDGE_CURVE('',#6895,#6896,#136,.T.);
#8904=EDGE_CURVE('',#6895,#6897,#4428,.T.);
#8905=EDGE_CURVE('',#6898,#6897,#137,.T.);
#8906=EDGE_CURVE('',#6896,#6898,#4429,.T.);
#8907=EDGE_CURVE('',#6899,#6895,#138,.T.);
#8908=EDGE_CURVE('',#6900,#6899,#4430,.T.);
#8909=EDGE_CURVE('',#6897,#6900,#139,.T.);
#8910=EDGE_CURVE('',#6901,#6902,#140,.T.);
#8911=EDGE_CURVE('',#6901,#6903,#4431,.T.);
#8912=EDGE_CURVE('',#6904,#6903,#141,.T.);
#8913=EDGE_CURVE('',#6902,#6904,#4432,.T.);
#8914=EDGE_CURVE('',#6905,#6901,#142,.T.);
#8915=EDGE_CURVE('',#6906,#6905,#4433,.T.);
#8916=EDGE_CURVE('',#6903,#6906,#143,.T.);
#8917=EDGE_CURVE('',#6907,#6908,#144,.T.);
#8918=EDGE_CURVE('',#6907,#6909,#4434,.T.);
#8919=EDGE_CURVE('',#6910,#6909,#145,.T.);
#8920=EDGE_CURVE('',#6908,#6910,#4435,.T.);
#8921=EDGE_CURVE('',#6911,#6907,#146,.T.);
#8922=EDGE_CURVE('',#6912,#6911,#4436,.T.);
#8923=EDGE_CURVE('',#6909,#6912,#147,.T.);
#8924=EDGE_CURVE('',#6913,#6914,#148,.T.);
#8925=EDGE_CURVE('',#6913,#6915,#4437,.T.);
#8926=EDGE_CURVE('',#6916,#6915,#149,.T.);
#8927=EDGE_CURVE('',#6914,#6916,#4438,.T.);
#8928=EDGE_CURVE('',#6917,#6913,#150,.T.);
#8929=EDGE_CURVE('',#6918,#6917,#4439,.T.);
#8930=EDGE_CURVE('',#6915,#6918,#151,.T.);
#8931=EDGE_CURVE('',#6919,#6920,#152,.T.);
#8932=EDGE_CURVE('',#6919,#6921,#4440,.T.);
#8933=EDGE_CURVE('',#6922,#6921,#153,.T.);
#8934=EDGE_CURVE('',#6920,#6922,#4441,.T.);
#8935=EDGE_CURVE('',#6923,#6919,#154,.T.);
#8936=EDGE_CURVE('',#6924,#6923,#4442,.T.);
#8937=EDGE_CURVE('',#6921,#6924,#155,.T.);
#8938=EDGE_CURVE('',#6925,#6926,#156,.T.);
#8939=EDGE_CURVE('',#6925,#6927,#4443,.T.);
#8940=EDGE_CURVE('',#6928,#6927,#157,.T.);
#8941=EDGE_CURVE('',#6926,#6928,#4444,.T.);
#8942=EDGE_CURVE('',#6929,#6925,#158,.T.);
#8943=EDGE_CURVE('',#6930,#6929,#4445,.T.);
#8944=EDGE_CURVE('',#6927,#6930,#159,.T.);
#8945=EDGE_CURVE('',#6931,#6932,#160,.T.);
#8946=EDGE_CURVE('',#6931,#6933,#4446,.T.);
#8947=EDGE_CURVE('',#6934,#6933,#161,.T.);
#8948=EDGE_CURVE('',#6932,#6934,#4447,.T.);
#8949=EDGE_CURVE('',#6935,#6931,#162,.T.);
#8950=EDGE_CURVE('',#6936,#6935,#4448,.T.);
#8951=EDGE_CURVE('',#6933,#6936,#163,.T.);
#8952=EDGE_CURVE('',#6937,#6938,#164,.T.);
#8953=EDGE_CURVE('',#6937,#6939,#4449,.T.);
#8954=EDGE_CURVE('',#6940,#6939,#165,.T.);
#8955=EDGE_CURVE('',#6938,#6940,#4450,.T.);
#8956=EDGE_CURVE('',#6941,#6937,#166,.T.);
#8957=EDGE_CURVE('',#6942,#6941,#4451,.T.);
#8958=EDGE_CURVE('',#6939,#6942,#167,.T.);
#8959=EDGE_CURVE('',#6943,#6944,#168,.T.);
#8960=EDGE_CURVE('',#6943,#6945,#4452,.T.);
#8961=EDGE_CURVE('',#6946,#6945,#169,.T.);
#8962=EDGE_CURVE('',#6944,#6946,#4453,.T.);
#8963=EDGE_CURVE('',#6947,#6943,#170,.T.);
#8964=EDGE_CURVE('',#6948,#6947,#4454,.T.);
#8965=EDGE_CURVE('',#6945,#6948,#171,.T.);
#8966=EDGE_CURVE('',#6949,#6950,#172,.T.);
#8967=EDGE_CURVE('',#6949,#6951,#4455,.T.);
#8968=EDGE_CURVE('',#6952,#6951,#173,.T.);
#8969=EDGE_CURVE('',#6950,#6952,#4456,.T.);
#8970=EDGE_CURVE('',#6953,#6949,#174,.T.);
#8971=EDGE_CURVE('',#6954,#6953,#4457,.T.);
#8972=EDGE_CURVE('',#6951,#6954,#175,.T.);
#8973=EDGE_CURVE('',#6955,#6956,#176,.T.);
#8974=EDGE_CURVE('',#6955,#6957,#4458,.T.);
#8975=EDGE_CURVE('',#6958,#6957,#177,.T.);
#8976=EDGE_CURVE('',#6956,#6958,#4459,.T.);
#8977=EDGE_CURVE('',#6959,#6955,#178,.T.);
#8978=EDGE_CURVE('',#6960,#6959,#4460,.T.);
#8979=EDGE_CURVE('',#6957,#6960,#179,.T.);
#8980=EDGE_CURVE('',#6961,#6962,#180,.T.);
#8981=EDGE_CURVE('',#6961,#6963,#4461,.T.);
#8982=EDGE_CURVE('',#6964,#6963,#181,.T.);
#8983=EDGE_CURVE('',#6962,#6964,#4462,.T.);
#8984=EDGE_CURVE('',#6965,#6961,#182,.T.);
#8985=EDGE_CURVE('',#6966,#6965,#4463,.T.);
#8986=EDGE_CURVE('',#6963,#6966,#183,.T.);
#8987=EDGE_CURVE('',#6967,#6968,#184,.T.);
#8988=EDGE_CURVE('',#6967,#6969,#4464,.T.);
#8989=EDGE_CURVE('',#6970,#6969,#185,.T.);
#8990=EDGE_CURVE('',#6968,#6970,#4465,.T.);
#8991=EDGE_CURVE('',#6971,#6967,#186,.T.);
#8992=EDGE_CURVE('',#6972,#6971,#4466,.T.);
#8993=EDGE_CURVE('',#6969,#6972,#187,.T.);
#8994=EDGE_CURVE('',#6973,#6974,#188,.T.);
#8995=EDGE_CURVE('',#6973,#6975,#4467,.T.);
#8996=EDGE_CURVE('',#6976,#6975,#189,.T.);
#8997=EDGE_CURVE('',#6974,#6976,#4468,.T.);
#8998=EDGE_CURVE('',#6977,#6973,#190,.T.);
#8999=EDGE_CURVE('',#6978,#6977,#4469,.T.);
#9000=EDGE_CURVE('',#6975,#6978,#191,.T.);
#9001=EDGE_CURVE('',#6979,#6980,#192,.T.);
#9002=EDGE_CURVE('',#6979,#6981,#4470,.T.);
#9003=EDGE_CURVE('',#6982,#6981,#193,.T.);
#9004=EDGE_CURVE('',#6980,#6982,#4471,.T.);
#9005=EDGE_CURVE('',#6983,#6979,#194,.T.);
#9006=EDGE_CURVE('',#6984,#6983,#4472,.T.);
#9007=EDGE_CURVE('',#6981,#6984,#195,.T.);
#9008=EDGE_CURVE('',#6985,#6986,#196,.T.);
#9009=EDGE_CURVE('',#6985,#6987,#4473,.T.);
#9010=EDGE_CURVE('',#6988,#6987,#197,.T.);
#9011=EDGE_CURVE('',#6986,#6988,#4474,.T.);
#9012=EDGE_CURVE('',#6989,#6985,#198,.T.);
#9013=EDGE_CURVE('',#6990,#6989,#4475,.T.);
#9014=EDGE_CURVE('',#6987,#6990,#199,.T.);
#9015=EDGE_CURVE('',#6991,#6992,#200,.T.);
#9016=EDGE_CURVE('',#6991,#6993,#4476,.T.);
#9017=EDGE_CURVE('',#6994,#6993,#201,.T.);
#9018=EDGE_CURVE('',#6992,#6994,#4477,.T.);
#9019=EDGE_CURVE('',#6995,#6991,#202,.T.);
#9020=EDGE_CURVE('',#6996,#6995,#4478,.T.);
#9021=EDGE_CURVE('',#6993,#6996,#203,.T.);
#9022=EDGE_CURVE('',#6997,#6998,#204,.T.);
#9023=EDGE_CURVE('',#6997,#6999,#4479,.T.);
#9024=EDGE_CURVE('',#7000,#6999,#205,.T.);
#9025=EDGE_CURVE('',#6998,#7000,#4480,.T.);
#9026=EDGE_CURVE('',#7001,#6997,#206,.T.);
#9027=EDGE_CURVE('',#7002,#7001,#4481,.T.);
#9028=EDGE_CURVE('',#6999,#7002,#207,.T.);
#9029=EDGE_CURVE('',#7003,#7004,#208,.T.);
#9030=EDGE_CURVE('',#7003,#7005,#4482,.T.);
#9031=EDGE_CURVE('',#7006,#7005,#209,.T.);
#9032=EDGE_CURVE('',#7004,#7006,#4483,.T.);
#9033=EDGE_CURVE('',#7007,#7003,#210,.T.);
#9034=EDGE_CURVE('',#7008,#7007,#4484,.T.);
#9035=EDGE_CURVE('',#7005,#7008,#211,.T.);
#9036=EDGE_CURVE('',#7009,#7010,#212,.T.);
#9037=EDGE_CURVE('',#7009,#7011,#4485,.T.);
#9038=EDGE_CURVE('',#7012,#7011,#213,.T.);
#9039=EDGE_CURVE('',#7010,#7012,#4486,.T.);
#9040=EDGE_CURVE('',#7013,#7009,#214,.T.);
#9041=EDGE_CURVE('',#7014,#7013,#4487,.T.);
#9042=EDGE_CURVE('',#7011,#7014,#215,.T.);
#9043=EDGE_CURVE('',#7015,#7016,#216,.T.);
#9044=EDGE_CURVE('',#7015,#7017,#4488,.T.);
#9045=EDGE_CURVE('',#7018,#7017,#217,.T.);
#9046=EDGE_CURVE('',#7016,#7018,#4489,.T.);
#9047=EDGE_CURVE('',#7019,#7015,#218,.T.);
#9048=EDGE_CURVE('',#7020,#7019,#4490,.T.);
#9049=EDGE_CURVE('',#7017,#7020,#219,.T.);
#9050=EDGE_CURVE('',#7021,#7022,#220,.T.);
#9051=EDGE_CURVE('',#7021,#7023,#4491,.T.);
#9052=EDGE_CURVE('',#7024,#7023,#221,.T.);
#9053=EDGE_CURVE('',#7022,#7024,#4492,.T.);
#9054=EDGE_CURVE('',#7025,#7021,#222,.T.);
#9055=EDGE_CURVE('',#7026,#7025,#4493,.T.);
#9056=EDGE_CURVE('',#7023,#7026,#223,.T.);
#9057=EDGE_CURVE('',#7027,#7028,#224,.T.);
#9058=EDGE_CURVE('',#7027,#7029,#4494,.T.);
#9059=EDGE_CURVE('',#7030,#7029,#225,.T.);
#9060=EDGE_CURVE('',#7028,#7030,#4495,.T.);
#9061=EDGE_CURVE('',#7031,#7027,#226,.T.);
#9062=EDGE_CURVE('',#7032,#7031,#4496,.T.);
#9063=EDGE_CURVE('',#7029,#7032,#227,.T.);
#9064=EDGE_CURVE('',#7033,#7034,#228,.T.);
#9065=EDGE_CURVE('',#7033,#7035,#4497,.T.);
#9066=EDGE_CURVE('',#7036,#7035,#229,.T.);
#9067=EDGE_CURVE('',#7034,#7036,#4498,.T.);
#9068=EDGE_CURVE('',#7037,#7033,#230,.T.);
#9069=EDGE_CURVE('',#7038,#7037,#4499,.T.);
#9070=EDGE_CURVE('',#7035,#7038,#231,.T.);
#9071=EDGE_CURVE('',#7039,#7040,#232,.T.);
#9072=EDGE_CURVE('',#7039,#7041,#4500,.T.);
#9073=EDGE_CURVE('',#7042,#7041,#233,.T.);
#9074=EDGE_CURVE('',#7040,#7042,#4501,.T.);
#9075=EDGE_CURVE('',#7043,#7039,#234,.T.);
#9076=EDGE_CURVE('',#7044,#7043,#4502,.T.);
#9077=EDGE_CURVE('',#7041,#7044,#235,.T.);
#9078=EDGE_CURVE('',#7045,#7046,#236,.T.);
#9079=EDGE_CURVE('',#7045,#7047,#4503,.T.);
#9080=EDGE_CURVE('',#7048,#7047,#237,.T.);
#9081=EDGE_CURVE('',#7046,#7048,#4504,.T.);
#9082=EDGE_CURVE('',#7049,#7045,#238,.T.);
#9083=EDGE_CURVE('',#7050,#7049,#4505,.T.);
#9084=EDGE_CURVE('',#7047,#7050,#239,.T.);
#9085=EDGE_CURVE('',#7051,#7052,#240,.T.);
#9086=EDGE_CURVE('',#7051,#7053,#4506,.T.);
#9087=EDGE_CURVE('',#7054,#7053,#241,.T.);
#9088=EDGE_CURVE('',#7052,#7054,#4507,.T.);
#9089=EDGE_CURVE('',#7055,#7051,#242,.T.);
#9090=EDGE_CURVE('',#7056,#7055,#4508,.T.);
#9091=EDGE_CURVE('',#7053,#7056,#243,.T.);
#9092=EDGE_CURVE('',#7057,#7058,#244,.T.);
#9093=EDGE_CURVE('',#7057,#7059,#4509,.T.);
#9094=EDGE_CURVE('',#7060,#7059,#245,.T.);
#9095=EDGE_CURVE('',#7058,#7060,#4510,.T.);
#9096=EDGE_CURVE('',#7061,#7057,#246,.T.);
#9097=EDGE_CURVE('',#7062,#7061,#4511,.T.);
#9098=EDGE_CURVE('',#7059,#7062,#247,.T.);
#9099=EDGE_CURVE('',#7063,#7064,#248,.T.);
#9100=EDGE_CURVE('',#7063,#7065,#4512,.T.);
#9101=EDGE_CURVE('',#7066,#7065,#249,.T.);
#9102=EDGE_CURVE('',#7064,#7066,#4513,.T.);
#9103=EDGE_CURVE('',#7067,#7063,#250,.T.);
#9104=EDGE_CURVE('',#7068,#7067,#4514,.T.);
#9105=EDGE_CURVE('',#7065,#7068,#251,.T.);
#9106=EDGE_CURVE('',#7018,#7026,#1451,.T.);
#9107=EDGE_CURVE('',#7016,#7025,#1452,.T.);
#9108=EDGE_CURVE('',#6976,#6984,#1453,.T.);
#9109=EDGE_CURVE('',#6974,#6983,#1454,.T.);
#9110=EDGE_CURVE('',#6980,#6971,#1455,.T.);
#9111=EDGE_CURVE('',#6982,#6972,#1456,.T.);
#9112=EDGE_CURVE('',#6970,#6990,#1457,.T.);
#9113=EDGE_CURVE('',#6968,#6989,#1458,.T.);
#9114=EDGE_CURVE('',#6986,#6965,#1459,.T.);
#9115=EDGE_CURVE('',#6988,#6966,#1460,.T.);
#9116=EDGE_CURVE('',#6964,#6996,#1461,.T.);
#9117=EDGE_CURVE('',#6962,#6995,#1462,.T.);
#9118=EDGE_CURVE('',#6992,#6959,#1463,.T.);
#9119=EDGE_CURVE('',#6994,#6960,#1464,.T.);
#9120=EDGE_CURVE('',#6958,#7002,#1465,.T.);
#9121=EDGE_CURVE('',#6956,#7001,#1466,.T.);
#9122=EDGE_CURVE('',#6998,#6953,#1467,.T.);
#9123=EDGE_CURVE('',#7000,#6954,#1468,.T.);
#9124=EDGE_CURVE('',#6952,#7008,#1469,.T.);
#9125=EDGE_CURVE('',#6950,#7007,#1470,.T.);
#9126=EDGE_CURVE('',#7004,#6947,#1471,.T.);
#9127=EDGE_CURVE('',#7006,#6948,#1472,.T.);
#9128=EDGE_CURVE('',#6946,#7014,#1473,.T.);
#9129=EDGE_CURVE('',#6944,#7013,#1474,.T.);
#9130=EDGE_CURVE('',#7010,#6941,#1475,.T.);
#9131=EDGE_CURVE('',#7012,#6942,#1476,.T.);
#9132=EDGE_CURVE('',#6940,#7020,#1477,.T.);
#9133=EDGE_CURVE('',#6938,#7019,#1478,.T.);
#9134=EDGE_CURVE('',#7064,#6935,#1479,.T.);
#9135=EDGE_CURVE('',#7066,#6936,#1480,.T.);
#9136=EDGE_CURVE('',#6934,#6978,#1481,.T.);
#9137=EDGE_CURVE('',#6932,#6977,#1482,.T.);
#9138=EDGE_CURVE('',#7022,#6929,#1483,.T.);
#9139=EDGE_CURVE('',#7024,#6930,#1484,.T.);
#9140=EDGE_CURVE('',#6928,#7032,#1485,.T.);
#9141=EDGE_CURVE('',#6926,#7031,#1486,.T.);
#9142=EDGE_CURVE('',#7028,#6923,#1487,.T.);
#9143=EDGE_CURVE('',#7030,#6924,#1488,.T.);
#9144=EDGE_CURVE('',#6922,#7038,#1489,.T.);
#9145=EDGE_CURVE('',#6920,#7037,#1490,.T.);
#9146=EDGE_CURVE('',#7034,#6917,#1491,.T.);
#9147=EDGE_CURVE('',#7036,#6918,#1492,.T.);
#9148=EDGE_CURVE('',#6916,#7044,#1493,.T.);
#9149=EDGE_CURVE('',#6914,#7043,#1494,.T.);
#9150=EDGE_CURVE('',#7040,#6911,#1495,.T.);
#9151=EDGE_CURVE('',#7042,#6912,#1496,.T.);
#9152=EDGE_CURVE('',#6910,#7050,#1497,.T.);
#9153=EDGE_CURVE('',#6908,#7049,#1498,.T.);
#9154=EDGE_CURVE('',#7046,#6905,#1499,.T.);
#9155=EDGE_CURVE('',#7048,#6906,#1500,.T.);
#9156=EDGE_CURVE('',#6904,#7056,#1501,.T.);
#9157=EDGE_CURVE('',#6902,#7055,#1502,.T.);
#9158=EDGE_CURVE('',#7052,#6899,#1503,.T.);
#9159=EDGE_CURVE('',#7054,#6900,#1504,.T.);
#9160=EDGE_CURVE('',#6898,#7062,#1505,.T.);
#9161=EDGE_CURVE('',#6896,#7061,#1506,.T.);
#9162=EDGE_CURVE('',#7058,#6893,#1507,.T.);
#9163=EDGE_CURVE('',#7060,#6894,#1508,.T.);
#9164=EDGE_CURVE('',#6892,#7068,#1509,.T.);
#9165=EDGE_CURVE('',#6890,#7067,#1510,.T.);
#9166=EDGE_CURVE('',#7023,#7069,#4515,.T.);
#9167=EDGE_CURVE('',#7069,#7069,#1511,.T.);
#9168=EDGE_CURVE('',#7070,#7070,#1512,.T.);
#9169=EDGE_CURVE('',#6887,#7070,#4516,.T.);
#9170=EDGE_CURVE('',#6824,#6885,#1513,.T.);
#9171=EDGE_CURVE('',#7071,#7071,#1514,.T.);
#9172=EDGE_CURVE('',#7071,#7021,#4517,.T.);
#12223=ORIENTED_EDGE('',*,*,#8727,.F.);
#12224=ORIENTED_EDGE('',*,*,#8728,.T.);
#12225=ORIENTED_EDGE('',*,*,#8729,.T.);
#12226=ORIENTED_EDGE('',*,*,#8730,.T.);
#12227=ORIENTED_EDGE('',*,*,#8731,.F.);
#12228=ORIENTED_EDGE('',*,*,#8732,.T.);
#12229=ORIENTED_EDGE('',*,*,#8727,.T.);
#12230=ORIENTED_EDGE('',*,*,#8733,.T.);
#12231=ORIENTED_EDGE('',*,*,#8734,.F.);
#12232=ORIENTED_EDGE('',*,*,#8735,.T.);
#12233=ORIENTED_EDGE('',*,*,#8731,.T.);
#12234=ORIENTED_EDGE('',*,*,#8736,.T.);
#12235=ORIENTED_EDGE('',*,*,#8737,.F.);
#12236=ORIENTED_EDGE('',*,*,#8738,.T.);
#12237=ORIENTED_EDGE('',*,*,#8734,.T.);
#12238=ORIENTED_EDGE('',*,*,#8739,.T.);
#12239=ORIENTED_EDGE('',*,*,#8740,.F.);
#12240=ORIENTED_EDGE('',*,*,#8741,.T.);
#12241=ORIENTED_EDGE('',*,*,#8737,.T.);
#12242=ORIENTED_EDGE('',*,*,#8742,.T.);
#12243=ORIENTED_EDGE('',*,*,#8743,.F.);
#12244=ORIENTED_EDGE('',*,*,#8744,.T.);
#12245=ORIENTED_EDGE('',*,*,#8740,.T.);
#12246=ORIENTED_EDGE('',*,*,#8745,.T.);
#12247=ORIENTED_EDGE('',*,*,#8746,.F.);
#12248=ORIENTED_EDGE('',*,*,#8747,.T.);
#12249=ORIENTED_EDGE('',*,*,#8743,.T.);
#12250=ORIENTED_EDGE('',*,*,#8748,.T.);
#12251=ORIENTED_EDGE('',*,*,#8749,.F.);
#12252=ORIENTED_EDGE('',*,*,#8750,.T.);
#12253=ORIENTED_EDGE('',*,*,#8746,.T.);
#12254=ORIENTED_EDGE('',*,*,#8751,.T.);
#12255=ORIENTED_EDGE('',*,*,#8752,.F.);
#12256=ORIENTED_EDGE('',*,*,#8753,.T.);
#12257=ORIENTED_EDGE('',*,*,#8749,.T.);
#12258=ORIENTED_EDGE('',*,*,#8754,.T.);
#12259=ORIENTED_EDGE('',*,*,#8755,.F.);
#12260=ORIENTED_EDGE('',*,*,#8756,.T.);
#12261=ORIENTED_EDGE('',*,*,#8752,.T.);
#12262=ORIENTED_EDGE('',*,*,#8757,.T.);
#12263=ORIENTED_EDGE('',*,*,#8758,.F.);
#12264=ORIENTED_EDGE('',*,*,#8759,.T.);
#12265=ORIENTED_EDGE('',*,*,#8755,.T.);
#12266=ORIENTED_EDGE('',*,*,#8760,.T.);
#12267=ORIENTED_EDGE('',*,*,#8761,.F.);
#12268=ORIENTED_EDGE('',*,*,#8762,.T.);
#12269=ORIENTED_EDGE('',*,*,#8758,.T.);
#12270=ORIENTED_EDGE('',*,*,#8763,.T.);
#12271=ORIENTED_EDGE('',*,*,#8764,.F.);
#12272=ORIENTED_EDGE('',*,*,#8765,.T.);
#12273=ORIENTED_EDGE('',*,*,#8761,.T.);
#12274=ORIENTED_EDGE('',*,*,#8766,.T.);
#12275=ORIENTED_EDGE('',*,*,#8767,.F.);
#12276=ORIENTED_EDGE('',*,*,#8768,.T.);
#12277=ORIENTED_EDGE('',*,*,#8764,.T.);
#12278=ORIENTED_EDGE('',*,*,#8769,.T.);
#12279=ORIENTED_EDGE('',*,*,#8770,.F.);
#12280=ORIENTED_EDGE('',*,*,#8771,.T.);
#12281=ORIENTED_EDGE('',*,*,#8767,.T.);
#12282=ORIENTED_EDGE('',*,*,#8772,.T.);
#12283=ORIENTED_EDGE('',*,*,#8773,.F.);
#12284=ORIENTED_EDGE('',*,*,#8774,.T.);
#12285=ORIENTED_EDGE('',*,*,#8770,.T.);
#12286=ORIENTED_EDGE('',*,*,#8775,.T.);
#12287=ORIENTED_EDGE('',*,*,#8776,.F.);
#12288=ORIENTED_EDGE('',*,*,#8777,.T.);
#12289=ORIENTED_EDGE('',*,*,#8773,.T.);
#12290=ORIENTED_EDGE('',*,*,#8778,.T.);
#12291=ORIENTED_EDGE('',*,*,#8779,.F.);
#12292=ORIENTED_EDGE('',*,*,#8780,.T.);
#12293=ORIENTED_EDGE('',*,*,#8776,.T.);
#12294=ORIENTED_EDGE('',*,*,#8781,.T.);
#12295=ORIENTED_EDGE('',*,*,#8782,.F.);
#12296=ORIENTED_EDGE('',*,*,#8783,.T.);
#12297=ORIENTED_EDGE('',*,*,#8779,.T.);
#12298=ORIENTED_EDGE('',*,*,#8784,.T.);
#12299=ORIENTED_EDGE('',*,*,#8785,.F.);
#12300=ORIENTED_EDGE('',*,*,#8786,.T.);
#12301=ORIENTED_EDGE('',*,*,#8782,.T.);
#12302=ORIENTED_EDGE('',*,*,#8787,.T.);
#12303=ORIENTED_EDGE('',*,*,#8788,.F.);
#12304=ORIENTED_EDGE('',*,*,#8789,.T.);
#12305=ORIENTED_EDGE('',*,*,#8785,.T.);
#12306=ORIENTED_EDGE('',*,*,#8790,.T.);
#12307=ORIENTED_EDGE('',*,*,#8791,.F.);
#12308=ORIENTED_EDGE('',*,*,#8792,.T.);
#12309=ORIENTED_EDGE('',*,*,#8788,.T.);
#12310=ORIENTED_EDGE('',*,*,#8793,.T.);
#12311=ORIENTED_EDGE('',*,*,#8794,.F.);
#12312=ORIENTED_EDGE('',*,*,#8795,.T.);
#12313=ORIENTED_EDGE('',*,*,#8791,.T.);
#12314=ORIENTED_EDGE('',*,*,#8796,.T.);
#12315=ORIENTED_EDGE('',*,*,#8797,.F.);
#12316=ORIENTED_EDGE('',*,*,#8798,.F.);
#12317=ORIENTED_EDGE('',*,*,#8799,.T.);
#12318=ORIENTED_EDGE('',*,*,#8794,.T.);
#12319=ORIENTED_EDGE('',*,*,#8800,.T.);
#12320=ORIENTED_EDGE('',*,*,#8801,.F.);
#12321=ORIENTED_EDGE('',*,*,#8802,.T.);
#12322=ORIENTED_EDGE('',*,*,#8803,.F.);
#12323=ORIENTED_EDGE('',*,*,#8804,.F.);
#12324=ORIENTED_EDGE('',*,*,#8805,.F.);
#12325=ORIENTED_EDGE('',*,*,#8806,.T.);
#12326=ORIENTED_EDGE('',*,*,#8801,.T.);
#12327=ORIENTED_EDGE('',*,*,#8807,.F.);
#12328=ORIENTED_EDGE('',*,*,#8808,.F.);
#12329=ORIENTED_EDGE('',*,*,#8809,.T.);
#12330=ORIENTED_EDGE('',*,*,#8805,.T.);
#12331=ORIENTED_EDGE('',*,*,#8810,.F.);
#12332=ORIENTED_EDGE('',*,*,#8811,.F.);
#12333=ORIENTED_EDGE('',*,*,#8812,.T.);
#12334=ORIENTED_EDGE('',*,*,#8808,.T.);
#12335=ORIENTED_EDGE('',*,*,#8813,.F.);
#12336=ORIENTED_EDGE('',*,*,#8814,.F.);
#12337=ORIENTED_EDGE('',*,*,#8815,.T.);
#12338=ORIENTED_EDGE('',*,*,#8811,.T.);
#12339=ORIENTED_EDGE('',*,*,#8816,.F.);
#12340=ORIENTED_EDGE('',*,*,#8817,.F.);
#12341=ORIENTED_EDGE('',*,*,#8818,.T.);
#12342=ORIENTED_EDGE('',*,*,#8814,.T.);
#12343=ORIENTED_EDGE('',*,*,#8819,.F.);
#12344=ORIENTED_EDGE('',*,*,#8820,.F.);
#12345=ORIENTED_EDGE('',*,*,#8821,.T.);
#12346=ORIENTED_EDGE('',*,*,#8817,.T.);
#12347=ORIENTED_EDGE('',*,*,#8822,.F.);
#12348=ORIENTED_EDGE('',*,*,#8823,.F.);
#12349=ORIENTED_EDGE('',*,*,#8824,.T.);
#12350=ORIENTED_EDGE('',*,*,#8820,.T.);
#12351=ORIENTED_EDGE('',*,*,#8825,.F.);
#12352=ORIENTED_EDGE('',*,*,#8826,.F.);
#12353=ORIENTED_EDGE('',*,*,#8827,.T.);
#12354=ORIENTED_EDGE('',*,*,#8823,.T.);
#12355=ORIENTED_EDGE('',*,*,#8828,.F.);
#12356=ORIENTED_EDGE('',*,*,#8829,.F.);
#12357=ORIENTED_EDGE('',*,*,#8830,.T.);
#12358=ORIENTED_EDGE('',*,*,#8826,.T.);
#12359=ORIENTED_EDGE('',*,*,#8831,.F.);
#12360=ORIENTED_EDGE('',*,*,#8832,.F.);
#12361=ORIENTED_EDGE('',*,*,#8833,.T.);
#12362=ORIENTED_EDGE('',*,*,#8829,.T.);
#12363=ORIENTED_EDGE('',*,*,#8834,.F.);
#12364=ORIENTED_EDGE('',*,*,#8835,.F.);
#12365=ORIENTED_EDGE('',*,*,#8836,.T.);
#12366=ORIENTED_EDGE('',*,*,#8832,.T.);
#12367=ORIENTED_EDGE('',*,*,#8837,.F.);
#12368=ORIENTED_EDGE('',*,*,#8838,.F.);
#12369=ORIENTED_EDGE('',*,*,#8839,.T.);
#12370=ORIENTED_EDGE('',*,*,#8835,.T.);
#12371=ORIENTED_EDGE('',*,*,#8840,.F.);
#12372=ORIENTED_EDGE('',*,*,#8841,.F.);
#12373=ORIENTED_EDGE('',*,*,#8842,.T.);
#12374=ORIENTED_EDGE('',*,*,#8838,.T.);
#12375=ORIENTED_EDGE('',*,*,#8843,.F.);
#12376=ORIENTED_EDGE('',*,*,#8844,.F.);
#12377=ORIENTED_EDGE('',*,*,#8845,.T.);
#12378=ORIENTED_EDGE('',*,*,#8841,.T.);
#12379=ORIENTED_EDGE('',*,*,#8846,.F.);
#12380=ORIENTED_EDGE('',*,*,#8847,.F.);
#12381=ORIENTED_EDGE('',*,*,#8848,.T.);
#12382=ORIENTED_EDGE('',*,*,#8844,.T.);
#12383=ORIENTED_EDGE('',*,*,#8849,.F.);
#12384=ORIENTED_EDGE('',*,*,#8850,.F.);
#12385=ORIENTED_EDGE('',*,*,#8851,.T.);
#12386=ORIENTED_EDGE('',*,*,#8847,.T.);
#12387=ORIENTED_EDGE('',*,*,#8852,.F.);
#12388=ORIENTED_EDGE('',*,*,#8853,.F.);
#12389=ORIENTED_EDGE('',*,*,#8854,.T.);
#12390=ORIENTED_EDGE('',*,*,#8850,.T.);
#12391=ORIENTED_EDGE('',*,*,#8855,.F.);
#12392=ORIENTED_EDGE('',*,*,#8856,.F.);
#12393=ORIENTED_EDGE('',*,*,#8857,.T.);
#12394=ORIENTED_EDGE('',*,*,#8853,.T.);
#12395=ORIENTED_EDGE('',*,*,#8858,.F.);
#12396=ORIENTED_EDGE('',*,*,#8859,.F.);
#12397=ORIENTED_EDGE('',*,*,#8860,.T.);
#12398=ORIENTED_EDGE('',*,*,#8856,.T.);
#12399=ORIENTED_EDGE('',*,*,#8861,.F.);
#12400=ORIENTED_EDGE('',*,*,#8862,.F.);
#12401=ORIENTED_EDGE('',*,*,#8863,.T.);
#12402=ORIENTED_EDGE('',*,*,#8859,.T.);
#12403=ORIENTED_EDGE('',*,*,#8864,.F.);
#12404=ORIENTED_EDGE('',*,*,#8865,.F.);
#12405=ORIENTED_EDGE('',*,*,#8866,.T.);
#12406=ORIENTED_EDGE('',*,*,#8862,.T.);
#12407=ORIENTED_EDGE('',*,*,#8867,.F.);
#12408=ORIENTED_EDGE('',*,*,#8868,.F.);
#12409=ORIENTED_EDGE('',*,*,#8869,.T.);
#12410=ORIENTED_EDGE('',*,*,#8865,.T.);
#12411=ORIENTED_EDGE('',*,*,#8870,.F.);
#12412=ORIENTED_EDGE('',*,*,#8871,.F.);
#12413=ORIENTED_EDGE('',*,*,#8872,.T.);
#12414=ORIENTED_EDGE('',*,*,#8873,.T.);
#12415=ORIENTED_EDGE('',*,*,#8874,.F.);
#12416=ORIENTED_EDGE('',*,*,#8875,.F.);
#12417=ORIENTED_EDGE('',*,*,#8876,.T.);
#12418=ORIENTED_EDGE('',*,*,#8877,.T.);
#12419=ORIENTED_EDGE('',*,*,#8872,.F.);
#12420=ORIENTED_EDGE('',*,*,#8878,.F.);
#12421=ORIENTED_EDGE('',*,*,#8879,.T.);
#12422=ORIENTED_EDGE('',*,*,#8880,.T.);
#12423=ORIENTED_EDGE('',*,*,#8876,.F.);
#12424=ORIENTED_EDGE('',*,*,#8881,.F.);
#12425=ORIENTED_EDGE('',*,*,#8874,.T.);
#12426=ORIENTED_EDGE('',*,*,#8882,.T.);
#12427=ORIENTED_EDGE('',*,*,#8879,.F.);
#12428=ORIENTED_EDGE('',*,*,#8882,.F.);
#12429=ORIENTED_EDGE('',*,*,#8873,.F.);
#12430=ORIENTED_EDGE('',*,*,#8877,.F.);
#12431=ORIENTED_EDGE('',*,*,#8880,.F.);
#12432=ORIENTED_EDGE('',*,*,#8883,.F.);
#12433=ORIENTED_EDGE('',*,*,#8884,.T.);
#12434=ORIENTED_EDGE('',*,*,#8885,.T.);
#12435=ORIENTED_EDGE('',*,*,#8884,.F.);
#12436=ORIENTED_EDGE('',*,*,#8885,.F.);
#12437=ORIENTED_EDGE('',*,*,#8886,.F.);
#12438=ORIENTED_EDGE('',*,*,#8887,.F.);
#12439=ORIENTED_EDGE('',*,*,#8800,.F.);
#12440=ORIENTED_EDGE('',*,*,#8796,.F.);
#12441=ORIENTED_EDGE('',*,*,#8793,.F.);
#12442=ORIENTED_EDGE('',*,*,#8790,.F.);
#12443=ORIENTED_EDGE('',*,*,#8787,.F.);
#12444=ORIENTED_EDGE('',*,*,#8784,.F.);
#12445=ORIENTED_EDGE('',*,*,#8781,.F.);
#12446=ORIENTED_EDGE('',*,*,#8778,.F.);
#12447=ORIENTED_EDGE('',*,*,#8775,.F.);
#12448=ORIENTED_EDGE('',*,*,#8772,.F.);
#12449=ORIENTED_EDGE('',*,*,#8769,.F.);
#12450=ORIENTED_EDGE('',*,*,#8766,.F.);
#12451=ORIENTED_EDGE('',*,*,#8763,.F.);
#12452=ORIENTED_EDGE('',*,*,#8760,.F.);
#12453=ORIENTED_EDGE('',*,*,#8757,.F.);
#12454=ORIENTED_EDGE('',*,*,#8754,.F.);
#12455=ORIENTED_EDGE('',*,*,#8751,.F.);
#12456=ORIENTED_EDGE('',*,*,#8748,.F.);
#12457=ORIENTED_EDGE('',*,*,#8745,.F.);
#12458=ORIENTED_EDGE('',*,*,#8742,.F.);
#12459=ORIENTED_EDGE('',*,*,#8739,.F.);
#12460=ORIENTED_EDGE('',*,*,#8736,.F.);
#12461=ORIENTED_EDGE('',*,*,#8733,.F.);
#12462=ORIENTED_EDGE('',*,*,#8730,.F.);
#12463=ORIENTED_EDGE('',*,*,#8888,.F.);
#12464=ORIENTED_EDGE('',*,*,#8889,.T.);
#12465=ORIENTED_EDGE('',*,*,#8870,.T.);
#12466=ORIENTED_EDGE('',*,*,#8867,.T.);
#12467=ORIENTED_EDGE('',*,*,#8864,.T.);
#12468=ORIENTED_EDGE('',*,*,#8861,.T.);
#12469=ORIENTED_EDGE('',*,*,#8858,.T.);
#12470=ORIENTED_EDGE('',*,*,#8855,.T.);
#12471=ORIENTED_EDGE('',*,*,#8852,.T.);
#12472=ORIENTED_EDGE('',*,*,#8849,.T.);
#12473=ORIENTED_EDGE('',*,*,#8846,.T.);
#12474=ORIENTED_EDGE('',*,*,#8843,.T.);
#12475=ORIENTED_EDGE('',*,*,#8840,.T.);
#12476=ORIENTED_EDGE('',*,*,#8837,.T.);
#12477=ORIENTED_EDGE('',*,*,#8834,.T.);
#12478=ORIENTED_EDGE('',*,*,#8831,.T.);
#12479=ORIENTED_EDGE('',*,*,#8828,.T.);
#12480=ORIENTED_EDGE('',*,*,#8825,.T.);
#12481=ORIENTED_EDGE('',*,*,#8822,.T.);
#12482=ORIENTED_EDGE('',*,*,#8819,.T.);
#12483=ORIENTED_EDGE('',*,*,#8816,.T.);
#12484=ORIENTED_EDGE('',*,*,#8813,.T.);
#12485=ORIENTED_EDGE('',*,*,#8810,.T.);
#12486=ORIENTED_EDGE('',*,*,#8807,.T.);
#12487=ORIENTED_EDGE('',*,*,#8804,.T.);
#12488=ORIENTED_EDGE('',*,*,#8890,.T.);
#12489=ORIENTED_EDGE('',*,*,#8891,.T.);
#12490=ORIENTED_EDGE('',*,*,#8892,.T.);
#12491=ORIENTED_EDGE('',*,*,#8893,.T.);
#12492=ORIENTED_EDGE('',*,*,#8888,.T.);
#12493=ORIENTED_EDGE('',*,*,#8868,.T.);
#12494=ORIENTED_EDGE('',*,*,#8889,.F.);
#12495=ORIENTED_EDGE('',*,*,#8893,.F.);
#12496=ORIENTED_EDGE('',*,*,#8894,.T.);
#12497=ORIENTED_EDGE('',*,*,#8895,.F.);
#12498=ORIENTED_EDGE('',*,*,#8802,.F.);
#12499=ORIENTED_EDGE('',*,*,#8806,.F.);
#12500=ORIENTED_EDGE('',*,*,#8809,.F.);
#12501=ORIENTED_EDGE('',*,*,#8812,.F.);
#12502=ORIENTED_EDGE('',*,*,#8815,.F.);
#12503=ORIENTED_EDGE('',*,*,#8818,.F.);
#12504=ORIENTED_EDGE('',*,*,#8821,.F.);
#12505=ORIENTED_EDGE('',*,*,#8824,.F.);
#12506=ORIENTED_EDGE('',*,*,#8827,.F.);
#12507=ORIENTED_EDGE('',*,*,#8830,.F.);
#12508=ORIENTED_EDGE('',*,*,#8833,.F.);
#12509=ORIENTED_EDGE('',*,*,#8836,.F.);
#12510=ORIENTED_EDGE('',*,*,#8839,.F.);
#12511=ORIENTED_EDGE('',*,*,#8842,.F.);
#12512=ORIENTED_EDGE('',*,*,#8845,.F.);
#12513=ORIENTED_EDGE('',*,*,#8848,.F.);
#12514=ORIENTED_EDGE('',*,*,#8851,.F.);
#12515=ORIENTED_EDGE('',*,*,#8854,.F.);
#12516=ORIENTED_EDGE('',*,*,#8857,.F.);
#12517=ORIENTED_EDGE('',*,*,#8860,.F.);
#12518=ORIENTED_EDGE('',*,*,#8863,.F.);
#12519=ORIENTED_EDGE('',*,*,#8866,.F.);
#12520=ORIENTED_EDGE('',*,*,#8869,.F.);
#12521=ORIENTED_EDGE('',*,*,#8894,.F.);
#12522=ORIENTED_EDGE('',*,*,#8892,.F.);
#12523=ORIENTED_EDGE('',*,*,#8728,.F.);
#12524=ORIENTED_EDGE('',*,*,#8732,.F.);
#12525=ORIENTED_EDGE('',*,*,#8735,.F.);
#12526=ORIENTED_EDGE('',*,*,#8738,.F.);
#12527=ORIENTED_EDGE('',*,*,#8741,.F.);
#12528=ORIENTED_EDGE('',*,*,#8744,.F.);
#12529=ORIENTED_EDGE('',*,*,#8747,.F.);
#12530=ORIENTED_EDGE('',*,*,#8750,.F.);
#12531=ORIENTED_EDGE('',*,*,#8753,.F.);
#12532=ORIENTED_EDGE('',*,*,#8756,.F.);
#12533=ORIENTED_EDGE('',*,*,#8759,.F.);
#12534=ORIENTED_EDGE('',*,*,#8762,.F.);
#12535=ORIENTED_EDGE('',*,*,#8765,.F.);
#12536=ORIENTED_EDGE('',*,*,#8768,.F.);
#12537=ORIENTED_EDGE('',*,*,#8771,.F.);
#12538=ORIENTED_EDGE('',*,*,#8774,.F.);
#12539=ORIENTED_EDGE('',*,*,#8777,.F.);
#12540=ORIENTED_EDGE('',*,*,#8780,.F.);
#12541=ORIENTED_EDGE('',*,*,#8783,.F.);
#12542=ORIENTED_EDGE('',*,*,#8786,.F.);
#12543=ORIENTED_EDGE('',*,*,#8789,.F.);
#12544=ORIENTED_EDGE('',*,*,#8792,.F.);
#12545=ORIENTED_EDGE('',*,*,#8795,.F.);
#12546=ORIENTED_EDGE('',*,*,#8799,.F.);
#12547=ORIENTED_EDGE('',*,*,#8896,.F.);
#12548=ORIENTED_EDGE('',*,*,#8897,.T.);
#12549=ORIENTED_EDGE('',*,*,#8898,.F.);
#12550=ORIENTED_EDGE('',*,*,#8899,.F.);
#12551=ORIENTED_EDGE('',*,*,#8900,.F.);
#12552=ORIENTED_EDGE('',*,*,#8901,.F.);
#12553=ORIENTED_EDGE('',*,*,#8902,.F.);
#12554=ORIENTED_EDGE('',*,*,#8897,.F.);
#12555=ORIENTED_EDGE('',*,*,#8903,.F.);
#12556=ORIENTED_EDGE('',*,*,#8904,.T.);
#12557=ORIENTED_EDGE('',*,*,#8905,.F.);
#12558=ORIENTED_EDGE('',*,*,#8906,.F.);
#12559=ORIENTED_EDGE('',*,*,#8907,.F.);
#12560=ORIENTED_EDGE('',*,*,#8908,.F.);
#12561=ORIENTED_EDGE('',*,*,#8909,.F.);
#12562=ORIENTED_EDGE('',*,*,#8904,.F.);
#12563=ORIENTED_EDGE('',*,*,#8910,.F.);
#12564=ORIENTED_EDGE('',*,*,#8911,.T.);
#12565=ORIENTED_EDGE('',*,*,#8912,.F.);
#12566=ORIENTED_EDGE('',*,*,#8913,.F.);
#12567=ORIENTED_EDGE('',*,*,#8914,.F.);
#12568=ORIENTED_EDGE('',*,*,#8915,.F.);
#12569=ORIENTED_EDGE('',*,*,#8916,.F.);
#12570=ORIENTED_EDGE('',*,*,#8911,.F.);
#12571=ORIENTED_EDGE('',*,*,#8917,.F.);
#12572=ORIENTED_EDGE('',*,*,#8918,.T.);
#12573=ORIENTED_EDGE('',*,*,#8919,.F.);
#12574=ORIENTED_EDGE('',*,*,#8920,.F.);
#12575=ORIENTED_EDGE('',*,*,#8921,.F.);
#12576=ORIENTED_EDGE('',*,*,#8922,.F.);
#12577=ORIENTED_EDGE('',*,*,#8923,.F.);
#12578=ORIENTED_EDGE('',*,*,#8918,.F.);
#12579=ORIENTED_EDGE('',*,*,#8924,.F.);
#12580=ORIENTED_EDGE('',*,*,#8925,.T.);
#12581=ORIENTED_EDGE('',*,*,#8926,.F.);
#12582=ORIENTED_EDGE('',*,*,#8927,.F.);
#12583=ORIENTED_EDGE('',*,*,#8928,.F.);
#12584=ORIENTED_EDGE('',*,*,#8929,.F.);
#12585=ORIENTED_EDGE('',*,*,#8930,.F.);
#12586=ORIENTED_EDGE('',*,*,#8925,.F.);
#12587=ORIENTED_EDGE('',*,*,#8931,.F.);
#12588=ORIENTED_EDGE('',*,*,#8932,.T.);
#12589=ORIENTED_EDGE('',*,*,#8933,.F.);
#12590=ORIENTED_EDGE('',*,*,#8934,.F.);
#12591=ORIENTED_EDGE('',*,*,#8935,.F.);
#12592=ORIENTED_EDGE('',*,*,#8936,.F.);
#12593=ORIENTED_EDGE('',*,*,#8937,.F.);
#12594=ORIENTED_EDGE('',*,*,#8932,.F.);
#12595=ORIENTED_EDGE('',*,*,#8938,.F.);
#12596=ORIENTED_EDGE('',*,*,#8939,.T.);
#12597=ORIENTED_EDGE('',*,*,#8940,.F.);
#12598=ORIENTED_EDGE('',*,*,#8941,.F.);
#12599=ORIENTED_EDGE('',*,*,#8942,.F.);
#12600=ORIENTED_EDGE('',*,*,#8943,.F.);
#12601=ORIENTED_EDGE('',*,*,#8944,.F.);
#12602=ORIENTED_EDGE('',*,*,#8939,.F.);
#12603=ORIENTED_EDGE('',*,*,#8945,.F.);
#12604=ORIENTED_EDGE('',*,*,#8946,.T.);
#12605=ORIENTED_EDGE('',*,*,#8947,.F.);
#12606=ORIENTED_EDGE('',*,*,#8948,.F.);
#12607=ORIENTED_EDGE('',*,*,#8949,.F.);
#12608=ORIENTED_EDGE('',*,*,#8950,.F.);
#12609=ORIENTED_EDGE('',*,*,#8951,.F.);
#12610=ORIENTED_EDGE('',*,*,#8946,.F.);
#12611=ORIENTED_EDGE('',*,*,#8952,.F.);
#12612=ORIENTED_EDGE('',*,*,#8953,.T.);
#12613=ORIENTED_EDGE('',*,*,#8954,.F.);
#12614=ORIENTED_EDGE('',*,*,#8955,.F.);
#12615=ORIENTED_EDGE('',*,*,#8956,.F.);
#12616=ORIENTED_EDGE('',*,*,#8957,.F.);
#12617=ORIENTED_EDGE('',*,*,#8958,.F.);
#12618=ORIENTED_EDGE('',*,*,#8953,.F.);
#12619=ORIENTED_EDGE('',*,*,#8959,.F.);
#12620=ORIENTED_EDGE('',*,*,#8960,.T.);
#12621=ORIENTED_EDGE('',*,*,#8961,.F.);
#12622=ORIENTED_EDGE('',*,*,#8962,.F.);
#12623=ORIENTED_EDGE('',*,*,#8963,.F.);
#12624=ORIENTED_EDGE('',*,*,#8964,.F.);
#12625=ORIENTED_EDGE('',*,*,#8965,.F.);
#12626=ORIENTED_EDGE('',*,*,#8960,.F.);
#12627=ORIENTED_EDGE('',*,*,#8966,.F.);
#12628=ORIENTED_EDGE('',*,*,#8967,.T.);
#12629=ORIENTED_EDGE('',*,*,#8968,.F.);
#12630=ORIENTED_EDGE('',*,*,#8969,.F.);
#12631=ORIENTED_EDGE('',*,*,#8970,.F.);
#12632=ORIENTED_EDGE('',*,*,#8971,.F.);
#12633=ORIENTED_EDGE('',*,*,#8972,.F.);
#12634=ORIENTED_EDGE('',*,*,#8967,.F.);
#12635=ORIENTED_EDGE('',*,*,#8973,.F.);
#12636=ORIENTED_EDGE('',*,*,#8974,.T.);
#12637=ORIENTED_EDGE('',*,*,#8975,.F.);
#12638=ORIENTED_EDGE('',*,*,#8976,.F.);
#12639=ORIENTED_EDGE('',*,*,#8977,.F.);
#12640=ORIENTED_EDGE('',*,*,#8978,.F.);
#12641=ORIENTED_EDGE('',*,*,#8979,.F.);
#12642=ORIENTED_EDGE('',*,*,#8974,.F.);
#12643=ORIENTED_EDGE('',*,*,#8980,.F.);
#12644=ORIENTED_EDGE('',*,*,#8981,.T.);
#12645=ORIENTED_EDGE('',*,*,#8982,.F.);
#12646=ORIENTED_EDGE('',*,*,#8983,.F.);
#12647=ORIENTED_EDGE('',*,*,#8984,.F.);
#12648=ORIENTED_EDGE('',*,*,#8985,.F.);
#12649=ORIENTED_EDGE('',*,*,#8986,.F.);
#12650=ORIENTED_EDGE('',*,*,#8981,.F.);
#12651=ORIENTED_EDGE('',*,*,#8987,.F.);
#12652=ORIENTED_EDGE('',*,*,#8988,.T.);
#12653=ORIENTED_EDGE('',*,*,#8989,.F.);
#12654=ORIENTED_EDGE('',*,*,#8990,.F.);
#12655=ORIENTED_EDGE('',*,*,#8991,.F.);
#12656=ORIENTED_EDGE('',*,*,#8992,.F.);
#12657=ORIENTED_EDGE('',*,*,#8993,.F.);
#12658=ORIENTED_EDGE('',*,*,#8988,.F.);
#12659=ORIENTED_EDGE('',*,*,#8994,.F.);
#12660=ORIENTED_EDGE('',*,*,#8995,.T.);
#12661=ORIENTED_EDGE('',*,*,#8996,.F.);
#12662=ORIENTED_EDGE('',*,*,#8997,.F.);
#12663=ORIENTED_EDGE('',*,*,#8998,.F.);
#12664=ORIENTED_EDGE('',*,*,#8999,.F.);
#12665=ORIENTED_EDGE('',*,*,#9000,.F.);
#12666=ORIENTED_EDGE('',*,*,#8995,.F.);
#12667=ORIENTED_EDGE('',*,*,#9001,.F.);
#12668=ORIENTED_EDGE('',*,*,#9002,.T.);
#12669=ORIENTED_EDGE('',*,*,#9003,.F.);
#12670=ORIENTED_EDGE('',*,*,#9004,.F.);
#12671=ORIENTED_EDGE('',*,*,#9005,.F.);
#12672=ORIENTED_EDGE('',*,*,#9006,.F.);
#12673=ORIENTED_EDGE('',*,*,#9007,.F.);
#12674=ORIENTED_EDGE('',*,*,#9002,.F.);
#12675=ORIENTED_EDGE('',*,*,#9008,.F.);
#12676=ORIENTED_EDGE('',*,*,#9009,.T.);
#12677=ORIENTED_EDGE('',*,*,#9010,.F.);
#12678=ORIENTED_EDGE('',*,*,#9011,.F.);
#12679=ORIENTED_EDGE('',*,*,#9012,.F.);
#12680=ORIENTED_EDGE('',*,*,#9013,.F.);
#12681=ORIENTED_EDGE('',*,*,#9014,.F.);
#12682=ORIENTED_EDGE('',*,*,#9009,.F.);
#12683=ORIENTED_EDGE('',*,*,#9015,.F.);
#12684=ORIENTED_EDGE('',*,*,#9016,.T.);
#12685=ORIENTED_EDGE('',*,*,#9017,.F.);
#12686=ORIENTED_EDGE('',*,*,#9018,.F.);
#12687=ORIENTED_EDGE('',*,*,#9019,.F.);
#12688=ORIENTED_EDGE('',*,*,#9020,.F.);
#12689=ORIENTED_EDGE('',*,*,#9021,.F.);
#12690=ORIENTED_EDGE('',*,*,#9016,.F.);
#12691=ORIENTED_EDGE('',*,*,#9022,.F.);
#12692=ORIENTED_EDGE('',*,*,#9023,.T.);
#12693=ORIENTED_EDGE('',*,*,#9024,.F.);
#12694=ORIENTED_EDGE('',*,*,#9025,.F.);
#12695=ORIENTED_EDGE('',*,*,#9026,.F.);
#12696=ORIENTED_EDGE('',*,*,#9027,.F.);
#12697=ORIENTED_EDGE('',*,*,#9028,.F.);
#12698=ORIENTED_EDGE('',*,*,#9023,.F.);
#12699=ORIENTED_EDGE('',*,*,#9029,.F.);
#12700=ORIENTED_EDGE('',*,*,#9030,.T.);
#12701=ORIENTED_EDGE('',*,*,#9031,.F.);
#12702=ORIENTED_EDGE('',*,*,#9032,.F.);
#12703=ORIENTED_EDGE('',*,*,#9033,.F.);
#12704=ORIENTED_EDGE('',*,*,#9034,.F.);
#12705=ORIENTED_EDGE('',*,*,#9035,.F.);
#12706=ORIENTED_EDGE('',*,*,#9030,.F.);
#12707=ORIENTED_EDGE('',*,*,#9036,.F.);
#12708=ORIENTED_EDGE('',*,*,#9037,.T.);
#12709=ORIENTED_EDGE('',*,*,#9038,.F.);
#12710=ORIENTED_EDGE('',*,*,#9039,.F.);
#12711=ORIENTED_EDGE('',*,*,#9040,.F.);
#12712=ORIENTED_EDGE('',*,*,#9041,.F.);
#12713=ORIENTED_EDGE('',*,*,#9042,.F.);
#12714=ORIENTED_EDGE('',*,*,#9037,.F.);
#12715=ORIENTED_EDGE('',*,*,#9043,.F.);
#12716=ORIENTED_EDGE('',*,*,#9044,.T.);
#12717=ORIENTED_EDGE('',*,*,#9045,.F.);
#12718=ORIENTED_EDGE('',*,*,#9046,.F.);
#12719=ORIENTED_EDGE('',*,*,#9047,.F.);
#12720=ORIENTED_EDGE('',*,*,#9048,.F.);
#12721=ORIENTED_EDGE('',*,*,#9049,.F.);
#12722=ORIENTED_EDGE('',*,*,#9044,.F.);
#12723=ORIENTED_EDGE('',*,*,#9050,.F.);
#12724=ORIENTED_EDGE('',*,*,#9051,.T.);
#12725=ORIENTED_EDGE('',*,*,#9052,.F.);
#12726=ORIENTED_EDGE('',*,*,#9053,.F.);
#12727=ORIENTED_EDGE('',*,*,#9054,.F.);
#12728=ORIENTED_EDGE('',*,*,#9055,.F.);
#12729=ORIENTED_EDGE('',*,*,#9056,.F.);
#12730=ORIENTED_EDGE('',*,*,#9051,.F.);
#12731=ORIENTED_EDGE('',*,*,#9057,.F.);
#12732=ORIENTED_EDGE('',*,*,#9058,.T.);
#12733=ORIENTED_EDGE('',*,*,#9059,.F.);
#12734=ORIENTED_EDGE('',*,*,#9060,.F.);
#12735=ORIENTED_EDGE('',*,*,#9061,.F.);
#12736=ORIENTED_EDGE('',*,*,#9062,.F.);
#12737=ORIENTED_EDGE('',*,*,#9063,.F.);
#12738=ORIENTED_EDGE('',*,*,#9058,.F.);
#12739=ORIENTED_EDGE('',*,*,#9064,.F.);
#12740=ORIENTED_EDGE('',*,*,#9065,.T.);
#12741=ORIENTED_EDGE('',*,*,#9066,.F.);
#12742=ORIENTED_EDGE('',*,*,#9067,.F.);
#12743=ORIENTED_EDGE('',*,*,#9068,.F.);
#12744=ORIENTED_EDGE('',*,*,#9069,.F.);
#12745=ORIENTED_EDGE('',*,*,#9070,.F.);
#12746=ORIENTED_EDGE('',*,*,#9065,.F.);
#12747=ORIENTED_EDGE('',*,*,#9071,.F.);
#12748=ORIENTED_EDGE('',*,*,#9072,.T.);
#12749=ORIENTED_EDGE('',*,*,#9073,.F.);
#12750=ORIENTED_EDGE('',*,*,#9074,.F.);
#12751=ORIENTED_EDGE('',*,*,#9075,.F.);
#12752=ORIENTED_EDGE('',*,*,#9076,.F.);
#12753=ORIENTED_EDGE('',*,*,#9077,.F.);
#12754=ORIENTED_EDGE('',*,*,#9072,.F.);
#12755=ORIENTED_EDGE('',*,*,#9078,.F.);
#12756=ORIENTED_EDGE('',*,*,#9079,.T.);
#12757=ORIENTED_EDGE('',*,*,#9080,.F.);
#12758=ORIENTED_EDGE('',*,*,#9081,.F.);
#12759=ORIENTED_EDGE('',*,*,#9082,.F.);
#12760=ORIENTED_EDGE('',*,*,#9083,.F.);
#12761=ORIENTED_EDGE('',*,*,#9084,.F.);
#12762=ORIENTED_EDGE('',*,*,#9079,.F.);
#12763=ORIENTED_EDGE('',*,*,#9085,.F.);
#12764=ORIENTED_EDGE('',*,*,#9086,.T.);
#12765=ORIENTED_EDGE('',*,*,#9087,.F.);
#12766=ORIENTED_EDGE('',*,*,#9088,.F.);
#12767=ORIENTED_EDGE('',*,*,#9089,.F.);
#12768=ORIENTED_EDGE('',*,*,#9090,.F.);
#12769=ORIENTED_EDGE('',*,*,#9091,.F.);
#12770=ORIENTED_EDGE('',*,*,#9086,.F.);
#12771=ORIENTED_EDGE('',*,*,#9092,.F.);
#12772=ORIENTED_EDGE('',*,*,#9093,.T.);
#12773=ORIENTED_EDGE('',*,*,#9094,.F.);
#12774=ORIENTED_EDGE('',*,*,#9095,.F.);
#12775=ORIENTED_EDGE('',*,*,#9096,.F.);
#12776=ORIENTED_EDGE('',*,*,#9097,.F.);
#12777=ORIENTED_EDGE('',*,*,#9098,.F.);
#12778=ORIENTED_EDGE('',*,*,#9093,.F.);
#12779=ORIENTED_EDGE('',*,*,#9099,.F.);
#12780=ORIENTED_EDGE('',*,*,#9100,.T.);
#12781=ORIENTED_EDGE('',*,*,#9101,.F.);
#12782=ORIENTED_EDGE('',*,*,#9102,.F.);
#12783=ORIENTED_EDGE('',*,*,#9103,.F.);
#12784=ORIENTED_EDGE('',*,*,#9104,.F.);
#12785=ORIENTED_EDGE('',*,*,#9105,.F.);
#12786=ORIENTED_EDGE('',*,*,#9100,.F.);
#12787=ORIENTED_EDGE('',*,*,#9046,.T.);
#12788=ORIENTED_EDGE('',*,*,#9106,.T.);
#12789=ORIENTED_EDGE('',*,*,#9055,.T.);
#12790=ORIENTED_EDGE('',*,*,#9107,.F.);
#12791=ORIENTED_EDGE('',*,*,#8997,.T.);
#12792=ORIENTED_EDGE('',*,*,#9108,.T.);
#12793=ORIENTED_EDGE('',*,*,#9006,.T.);
#12794=ORIENTED_EDGE('',*,*,#9109,.F.);
#12795=ORIENTED_EDGE('',*,*,#8992,.T.);
#12796=ORIENTED_EDGE('',*,*,#9110,.F.);
#12797=ORIENTED_EDGE('',*,*,#9004,.T.);
#12798=ORIENTED_EDGE('',*,*,#9111,.T.);
#12799=ORIENTED_EDGE('',*,*,#8990,.T.);
#12800=ORIENTED_EDGE('',*,*,#9112,.T.);
#12801=ORIENTED_EDGE('',*,*,#9013,.T.);
#12802=ORIENTED_EDGE('',*,*,#9113,.F.);
#12803=ORIENTED_EDGE('',*,*,#8985,.T.);
#12804=ORIENTED_EDGE('',*,*,#9114,.F.);
#12805=ORIENTED_EDGE('',*,*,#9011,.T.);
#12806=ORIENTED_EDGE('',*,*,#9115,.T.);
#12807=ORIENTED_EDGE('',*,*,#8983,.T.);
#12808=ORIENTED_EDGE('',*,*,#9116,.T.);
#12809=ORIENTED_EDGE('',*,*,#9020,.T.);
#12810=ORIENTED_EDGE('',*,*,#9117,.F.);
#12811=ORIENTED_EDGE('',*,*,#8978,.T.);
#12812=ORIENTED_EDGE('',*,*,#9118,.F.);
#12813=ORIENTED_EDGE('',*,*,#9018,.T.);
#12814=ORIENTED_EDGE('',*,*,#9119,.T.);
#12815=ORIENTED_EDGE('',*,*,#8976,.T.);
#12816=ORIENTED_EDGE('',*,*,#9120,.T.);
#12817=ORIENTED_EDGE('',*,*,#9027,.T.);
#12818=ORIENTED_EDGE('',*,*,#9121,.F.);
#12819=ORIENTED_EDGE('',*,*,#8971,.T.);
#12820=ORIENTED_EDGE('',*,*,#9122,.F.);
#12821=ORIENTED_EDGE('',*,*,#9025,.T.);
#12822=ORIENTED_EDGE('',*,*,#9123,.T.);
#12823=ORIENTED_EDGE('',*,*,#8969,.T.);
#12824=ORIENTED_EDGE('',*,*,#9124,.T.);
#12825=ORIENTED_EDGE('',*,*,#9034,.T.);
#12826=ORIENTED_EDGE('',*,*,#9125,.F.);
#12827=ORIENTED_EDGE('',*,*,#8964,.T.);
#12828=ORIENTED_EDGE('',*,*,#9126,.F.);
#12829=ORIENTED_EDGE('',*,*,#9032,.T.);
#12830=ORIENTED_EDGE('',*,*,#9127,.T.);
#12831=ORIENTED_EDGE('',*,*,#8962,.T.);
#12832=ORIENTED_EDGE('',*,*,#9128,.T.);
#12833=ORIENTED_EDGE('',*,*,#9041,.T.);
#12834=ORIENTED_EDGE('',*,*,#9129,.F.);
#12835=ORIENTED_EDGE('',*,*,#8957,.T.);
#12836=ORIENTED_EDGE('',*,*,#9130,.F.);
#12837=ORIENTED_EDGE('',*,*,#9039,.T.);
#12838=ORIENTED_EDGE('',*,*,#9131,.T.);
#12839=ORIENTED_EDGE('',*,*,#8955,.T.);
#12840=ORIENTED_EDGE('',*,*,#9132,.T.);
#12841=ORIENTED_EDGE('',*,*,#9048,.T.);
#12842=ORIENTED_EDGE('',*,*,#9133,.F.);
#12843=ORIENTED_EDGE('',*,*,#8950,.T.);
#12844=ORIENTED_EDGE('',*,*,#9134,.F.);
#12845=ORIENTED_EDGE('',*,*,#9102,.T.);
#12846=ORIENTED_EDGE('',*,*,#9135,.T.);
#12847=ORIENTED_EDGE('',*,*,#8948,.T.);
#12848=ORIENTED_EDGE('',*,*,#9136,.T.);
#12849=ORIENTED_EDGE('',*,*,#8999,.T.);
#12850=ORIENTED_EDGE('',*,*,#9137,.F.);
#12851=ORIENTED_EDGE('',*,*,#8943,.T.);
#12852=ORIENTED_EDGE('',*,*,#9138,.F.);
#12853=ORIENTED_EDGE('',*,*,#9053,.T.);
#12854=ORIENTED_EDGE('',*,*,#9139,.T.);
#12855=ORIENTED_EDGE('',*,*,#8941,.T.);
#12856=ORIENTED_EDGE('',*,*,#9140,.T.);
#12857=ORIENTED_EDGE('',*,*,#9062,.T.);
#12858=ORIENTED_EDGE('',*,*,#9141,.F.);
#12859=ORIENTED_EDGE('',*,*,#8936,.T.);
#12860=ORIENTED_EDGE('',*,*,#9142,.F.);
#12861=ORIENTED_EDGE('',*,*,#9060,.T.);
#12862=ORIENTED_EDGE('',*,*,#9143,.T.);
#12863=ORIENTED_EDGE('',*,*,#8934,.T.);
#12864=ORIENTED_EDGE('',*,*,#9144,.T.);
#12865=ORIENTED_EDGE('',*,*,#9069,.T.);
#12866=ORIENTED_EDGE('',*,*,#9145,.F.);
#12867=ORIENTED_EDGE('',*,*,#8929,.T.);
#12868=ORIENTED_EDGE('',*,*,#9146,.F.);
#12869=ORIENTED_EDGE('',*,*,#9067,.T.);
#12870=ORIENTED_EDGE('',*,*,#9147,.T.);
#12871=ORIENTED_EDGE('',*,*,#8927,.T.);
#12872=ORIENTED_EDGE('',*,*,#9148,.T.);
#12873=ORIENTED_EDGE('',*,*,#9076,.T.);
#12874=ORIENTED_EDGE('',*,*,#9149,.F.);
#12875=ORIENTED_EDGE('',*,*,#8922,.T.);
#12876=ORIENTED_EDGE('',*,*,#9150,.F.);
#12877=ORIENTED_EDGE('',*,*,#9074,.T.);
#12878=ORIENTED_EDGE('',*,*,#9151,.T.);
#12879=ORIENTED_EDGE('',*,*,#8920,.T.);
#12880=ORIENTED_EDGE('',*,*,#9152,.T.);
#12881=ORIENTED_EDGE('',*,*,#9083,.T.);
#12882=ORIENTED_EDGE('',*,*,#9153,.F.);
#12883=ORIENTED_EDGE('',*,*,#8915,.T.);
#12884=ORIENTED_EDGE('',*,*,#9154,.F.);
#12885=ORIENTED_EDGE('',*,*,#9081,.T.);
#12886=ORIENTED_EDGE('',*,*,#9155,.T.);
#12887=ORIENTED_EDGE('',*,*,#8913,.T.);
#12888=ORIENTED_EDGE('',*,*,#9156,.T.);
#12889=ORIENTED_EDGE('',*,*,#9090,.T.);
#12890=ORIENTED_EDGE('',*,*,#9157,.F.);
#12891=ORIENTED_EDGE('',*,*,#8908,.T.);
#12892=ORIENTED_EDGE('',*,*,#9158,.F.);
#12893=ORIENTED_EDGE('',*,*,#9088,.T.);
#12894=ORIENTED_EDGE('',*,*,#9159,.T.);
#12895=ORIENTED_EDGE('',*,*,#8906,.T.);
#12896=ORIENTED_EDGE('',*,*,#9160,.T.);
#12897=ORIENTED_EDGE('',*,*,#9097,.T.);
#12898=ORIENTED_EDGE('',*,*,#9161,.F.);
#12899=ORIENTED_EDGE('',*,*,#8901,.T.);
#12900=ORIENTED_EDGE('',*,*,#9162,.F.);
#12901=ORIENTED_EDGE('',*,*,#9095,.T.);
#12902=ORIENTED_EDGE('',*,*,#9163,.T.);
#12903=ORIENTED_EDGE('',*,*,#8899,.T.);
#12904=ORIENTED_EDGE('',*,*,#9164,.T.);
#12905=ORIENTED_EDGE('',*,*,#9104,.T.);
#12906=ORIENTED_EDGE('',*,*,#9165,.F.);
#12907=ORIENTED_EDGE('',*,*,#8898,.T.);
#12908=ORIENTED_EDGE('',*,*,#8902,.T.);
#12909=ORIENTED_EDGE('',*,*,#9163,.F.);
#12910=ORIENTED_EDGE('',*,*,#9094,.T.);
#12911=ORIENTED_EDGE('',*,*,#9098,.T.);
#12912=ORIENTED_EDGE('',*,*,#9160,.F.);
#12913=ORIENTED_EDGE('',*,*,#8905,.T.);
#12914=ORIENTED_EDGE('',*,*,#8909,.T.);
#12915=ORIENTED_EDGE('',*,*,#9159,.F.);
#12916=ORIENTED_EDGE('',*,*,#9087,.T.);
#12917=ORIENTED_EDGE('',*,*,#9091,.T.);
#12918=ORIENTED_EDGE('',*,*,#9156,.F.);
#12919=ORIENTED_EDGE('',*,*,#8912,.T.);
#12920=ORIENTED_EDGE('',*,*,#8916,.T.);
#12921=ORIENTED_EDGE('',*,*,#9155,.F.);
#12922=ORIENTED_EDGE('',*,*,#9080,.T.);
#12923=ORIENTED_EDGE('',*,*,#9084,.T.);
#12924=ORIENTED_EDGE('',*,*,#9152,.F.);
#12925=ORIENTED_EDGE('',*,*,#8919,.T.);
#12926=ORIENTED_EDGE('',*,*,#8923,.T.);
#12927=ORIENTED_EDGE('',*,*,#9151,.F.);
#12928=ORIENTED_EDGE('',*,*,#9073,.T.);
#12929=ORIENTED_EDGE('',*,*,#9077,.T.);
#12930=ORIENTED_EDGE('',*,*,#9148,.F.);
#12931=ORIENTED_EDGE('',*,*,#8926,.T.);
#12932=ORIENTED_EDGE('',*,*,#8930,.T.);
#12933=ORIENTED_EDGE('',*,*,#9147,.F.);
#12934=ORIENTED_EDGE('',*,*,#9066,.T.);
#12935=ORIENTED_EDGE('',*,*,#9070,.T.);
#12936=ORIENTED_EDGE('',*,*,#9144,.F.);
#12937=ORIENTED_EDGE('',*,*,#8933,.T.);
#12938=ORIENTED_EDGE('',*,*,#8937,.T.);
#12939=ORIENTED_EDGE('',*,*,#9143,.F.);
#12940=ORIENTED_EDGE('',*,*,#9059,.T.);
#12941=ORIENTED_EDGE('',*,*,#9063,.T.);
#12942=ORIENTED_EDGE('',*,*,#9140,.F.);
#12943=ORIENTED_EDGE('',*,*,#8940,.T.);
#12944=ORIENTED_EDGE('',*,*,#8944,.T.);
#12945=ORIENTED_EDGE('',*,*,#9139,.F.);
#12946=ORIENTED_EDGE('',*,*,#9052,.T.);
#12947=ORIENTED_EDGE('',*,*,#9166,.T.);
#12948=ORIENTED_EDGE('',*,*,#9167,.T.);
#12949=ORIENTED_EDGE('',*,*,#9166,.F.);
#12950=ORIENTED_EDGE('',*,*,#9056,.T.);
#12951=ORIENTED_EDGE('',*,*,#9106,.F.);
#12952=ORIENTED_EDGE('',*,*,#9045,.T.);
#12953=ORIENTED_EDGE('',*,*,#9049,.T.);
#12954=ORIENTED_EDGE('',*,*,#9132,.F.);
#12955=ORIENTED_EDGE('',*,*,#8954,.T.);
#12956=ORIENTED_EDGE('',*,*,#8958,.T.);
#12957=ORIENTED_EDGE('',*,*,#9131,.F.);
#12958=ORIENTED_EDGE('',*,*,#9038,.T.);
#12959=ORIENTED_EDGE('',*,*,#9042,.T.);
#12960=ORIENTED_EDGE('',*,*,#9128,.F.);
#12961=ORIENTED_EDGE('',*,*,#8961,.T.);
#12962=ORIENTED_EDGE('',*,*,#8965,.T.);
#12963=ORIENTED_EDGE('',*,*,#9127,.F.);
#12964=ORIENTED_EDGE('',*,*,#9031,.T.);
#12965=ORIENTED_EDGE('',*,*,#9035,.T.);
#12966=ORIENTED_EDGE('',*,*,#9124,.F.);
#12967=ORIENTED_EDGE('',*,*,#8968,.T.);
#12968=ORIENTED_EDGE('',*,*,#8972,.T.);
#12969=ORIENTED_EDGE('',*,*,#9123,.F.);
#12970=ORIENTED_EDGE('',*,*,#9024,.T.);
#12971=ORIENTED_EDGE('',*,*,#9028,.T.);
#12972=ORIENTED_EDGE('',*,*,#9120,.F.);
#12973=ORIENTED_EDGE('',*,*,#8975,.T.);
#12974=ORIENTED_EDGE('',*,*,#8979,.T.);
#12975=ORIENTED_EDGE('',*,*,#9119,.F.);
#12976=ORIENTED_EDGE('',*,*,#9017,.T.);
#12977=ORIENTED_EDGE('',*,*,#9021,.T.);
#12978=ORIENTED_EDGE('',*,*,#9116,.F.);
#12979=ORIENTED_EDGE('',*,*,#8982,.T.);
#12980=ORIENTED_EDGE('',*,*,#8986,.T.);
#12981=ORIENTED_EDGE('',*,*,#9115,.F.);
#12982=ORIENTED_EDGE('',*,*,#9010,.T.);
#12983=ORIENTED_EDGE('',*,*,#9014,.T.);
#12984=ORIENTED_EDGE('',*,*,#9112,.F.);
#12985=ORIENTED_EDGE('',*,*,#8989,.T.);
#12986=ORIENTED_EDGE('',*,*,#8993,.T.);
#12987=ORIENTED_EDGE('',*,*,#9111,.F.);
#12988=ORIENTED_EDGE('',*,*,#9003,.T.);
#12989=ORIENTED_EDGE('',*,*,#9007,.T.);
#12990=ORIENTED_EDGE('',*,*,#9108,.F.);
#12991=ORIENTED_EDGE('',*,*,#8996,.T.);
#12992=ORIENTED_EDGE('',*,*,#9000,.T.);
#12993=ORIENTED_EDGE('',*,*,#9136,.F.);
#12994=ORIENTED_EDGE('',*,*,#8947,.T.);
#12995=ORIENTED_EDGE('',*,*,#8951,.T.);
#12996=ORIENTED_EDGE('',*,*,#9135,.F.);
#12997=ORIENTED_EDGE('',*,*,#9101,.T.);
#12998=ORIENTED_EDGE('',*,*,#9105,.T.);
#12999=ORIENTED_EDGE('',*,*,#9164,.F.);
#13000=ORIENTED_EDGE('',*,*,#9168,.F.);
#13001=ORIENTED_EDGE('',*,*,#8883,.T.);
#13002=ORIENTED_EDGE('',*,*,#8890,.F.);
#13003=ORIENTED_EDGE('',*,*,#8729,.F.);
#13004=ORIENTED_EDGE('',*,*,#8891,.F.);
#13005=ORIENTED_EDGE('',*,*,#9169,.T.);
#13006=ORIENTED_EDGE('',*,*,#9168,.T.);
#13007=ORIENTED_EDGE('',*,*,#9169,.F.);
#13008=ORIENTED_EDGE('',*,*,#8797,.T.);
#13009=ORIENTED_EDGE('',*,*,#8887,.T.);
#13010=ORIENTED_EDGE('',*,*,#9170,.F.);
#13011=ORIENTED_EDGE('',*,*,#9167,.F.);
#13012=ORIENTED_EDGE('',*,*,#8798,.T.);
#13013=ORIENTED_EDGE('',*,*,#9170,.T.);
#13014=ORIENTED_EDGE('',*,*,#8886,.T.);
#13015=ORIENTED_EDGE('',*,*,#8803,.T.);
#13016=ORIENTED_EDGE('',*,*,#8895,.T.);
#13017=ORIENTED_EDGE('',*,*,#9171,.F.);
#13018=ORIENTED_EDGE('',*,*,#9172,.T.);
#13019=ORIENTED_EDGE('',*,*,#9050,.T.);
#13020=ORIENTED_EDGE('',*,*,#9138,.T.);
#13021=ORIENTED_EDGE('',*,*,#8942,.T.);
#13022=ORIENTED_EDGE('',*,*,#8938,.T.);
#13023=ORIENTED_EDGE('',*,*,#9141,.T.);
#13024=ORIENTED_EDGE('',*,*,#9061,.T.);
#13025=ORIENTED_EDGE('',*,*,#9057,.T.);
#13026=ORIENTED_EDGE('',*,*,#9142,.T.);
#13027=ORIENTED_EDGE('',*,*,#8935,.T.);
#13028=ORIENTED_EDGE('',*,*,#8931,.T.);
#13029=ORIENTED_EDGE('',*,*,#9145,.T.);
#13030=ORIENTED_EDGE('',*,*,#9068,.T.);
#13031=ORIENTED_EDGE('',*,*,#9064,.T.);
#13032=ORIENTED_EDGE('',*,*,#9146,.T.);
#13033=ORIENTED_EDGE('',*,*,#8928,.T.);
#13034=ORIENTED_EDGE('',*,*,#8924,.T.);
#13035=ORIENTED_EDGE('',*,*,#9149,.T.);
#13036=ORIENTED_EDGE('',*,*,#9075,.T.);
#13037=ORIENTED_EDGE('',*,*,#9071,.T.);
#13038=ORIENTED_EDGE('',*,*,#9150,.T.);
#13039=ORIENTED_EDGE('',*,*,#8921,.T.);
#13040=ORIENTED_EDGE('',*,*,#8917,.T.);
#13041=ORIENTED_EDGE('',*,*,#9153,.T.);
#13042=ORIENTED_EDGE('',*,*,#9082,.T.);
#13043=ORIENTED_EDGE('',*,*,#9078,.T.);
#13044=ORIENTED_EDGE('',*,*,#9154,.T.);
#13045=ORIENTED_EDGE('',*,*,#8914,.T.);
#13046=ORIENTED_EDGE('',*,*,#8910,.T.);
#13047=ORIENTED_EDGE('',*,*,#9157,.T.);
#13048=ORIENTED_EDGE('',*,*,#9089,.T.);
#13049=ORIENTED_EDGE('',*,*,#9085,.T.);
#13050=ORIENTED_EDGE('',*,*,#9158,.T.);
#13051=ORIENTED_EDGE('',*,*,#8907,.T.);
#13052=ORIENTED_EDGE('',*,*,#8903,.T.);
#13053=ORIENTED_EDGE('',*,*,#9161,.T.);
#13054=ORIENTED_EDGE('',*,*,#9096,.T.);
#13055=ORIENTED_EDGE('',*,*,#9092,.T.);
#13056=ORIENTED_EDGE('',*,*,#9162,.T.);
#13057=ORIENTED_EDGE('',*,*,#8900,.T.);
#13058=ORIENTED_EDGE('',*,*,#8896,.T.);
#13059=ORIENTED_EDGE('',*,*,#9165,.T.);
#13060=ORIENTED_EDGE('',*,*,#9103,.T.);
#13061=ORIENTED_EDGE('',*,*,#9099,.T.);
#13062=ORIENTED_EDGE('',*,*,#9134,.T.);
#13063=ORIENTED_EDGE('',*,*,#8949,.T.);
#13064=ORIENTED_EDGE('',*,*,#8945,.T.);
#13065=ORIENTED_EDGE('',*,*,#9137,.T.);
#13066=ORIENTED_EDGE('',*,*,#8998,.T.);
#13067=ORIENTED_EDGE('',*,*,#8994,.T.);
#13068=ORIENTED_EDGE('',*,*,#9109,.T.);
#13069=ORIENTED_EDGE('',*,*,#9005,.T.);
#13070=ORIENTED_EDGE('',*,*,#9001,.T.);
#13071=ORIENTED_EDGE('',*,*,#9110,.T.);
#13072=ORIENTED_EDGE('',*,*,#8991,.T.);
#13073=ORIENTED_EDGE('',*,*,#8987,.T.);
#13074=ORIENTED_EDGE('',*,*,#9113,.T.);
#13075=ORIENTED_EDGE('',*,*,#9012,.T.);
#13076=ORIENTED_EDGE('',*,*,#9008,.T.);
#13077=ORIENTED_EDGE('',*,*,#9114,.T.);
#13078=ORIENTED_EDGE('',*,*,#8984,.T.);
#13079=ORIENTED_EDGE('',*,*,#8980,.T.);
#13080=ORIENTED_EDGE('',*,*,#9117,.T.);
#13081=ORIENTED_EDGE('',*,*,#9019,.T.);
#13082=ORIENTED_EDGE('',*,*,#9015,.T.);
#13083=ORIENTED_EDGE('',*,*,#9118,.T.);
#13084=ORIENTED_EDGE('',*,*,#8977,.T.);
#13085=ORIENTED_EDGE('',*,*,#8973,.T.);
#13086=ORIENTED_EDGE('',*,*,#9121,.T.);
#13087=ORIENTED_EDGE('',*,*,#9026,.T.);
#13088=ORIENTED_EDGE('',*,*,#9022,.T.);
#13089=ORIENTED_EDGE('',*,*,#9122,.T.);
#13090=ORIENTED_EDGE('',*,*,#8970,.T.);
#13091=ORIENTED_EDGE('',*,*,#8966,.T.);
#13092=ORIENTED_EDGE('',*,*,#9125,.T.);
#13093=ORIENTED_EDGE('',*,*,#9033,.T.);
#13094=ORIENTED_EDGE('',*,*,#9029,.T.);
#13095=ORIENTED_EDGE('',*,*,#9126,.T.);
#13096=ORIENTED_EDGE('',*,*,#8963,.T.);
#13097=ORIENTED_EDGE('',*,*,#8959,.T.);
#13098=ORIENTED_EDGE('',*,*,#9129,.T.);
#13099=ORIENTED_EDGE('',*,*,#9040,.T.);
#13100=ORIENTED_EDGE('',*,*,#9036,.T.);
#13101=ORIENTED_EDGE('',*,*,#9130,.T.);
#13102=ORIENTED_EDGE('',*,*,#8956,.T.);
#13103=ORIENTED_EDGE('',*,*,#8952,.T.);
#13104=ORIENTED_EDGE('',*,*,#9133,.T.);
#13105=ORIENTED_EDGE('',*,*,#9047,.T.);
#13106=ORIENTED_EDGE('',*,*,#9043,.T.);
#13107=ORIENTED_EDGE('',*,*,#9107,.T.);
#13108=ORIENTED_EDGE('',*,*,#9054,.T.);
#13109=ORIENTED_EDGE('',*,*,#9172,.F.);
#13110=ORIENTED_EDGE('',*,*,#9171,.T.);
#13111=ORIENTED_EDGE('',*,*,#8871,.T.);
#13112=ORIENTED_EDGE('',*,*,#8881,.T.);
#13113=ORIENTED_EDGE('',*,*,#8878,.T.);
#13114=ORIENTED_EDGE('',*,*,#8875,.T.);
#15086=PLANE('',#17149);
#15087=PLANE('',#17150);
#15088=PLANE('',#17151);
#15089=PLANE('',#17152);
#15090=PLANE('',#17153);
#15091=PLANE('',#17157);
#15092=PLANE('',#17158);
#15093=PLANE('',#17163);
#15094=PLANE('',#17164);
#15095=PLANE('',#17165);
#15096=PLANE('',#17166);
#15097=PLANE('',#17167);
#15098=PLANE('',#17168);
#15099=PLANE('',#17169);
#15100=PLANE('',#17170);
#15101=PLANE('',#17171);
#15102=PLANE('',#17172);
#15103=PLANE('',#17173);
#15104=PLANE('',#17174);
#15105=PLANE('',#17175);
#15106=PLANE('',#17176);
#15107=PLANE('',#17177);
#15108=PLANE('',#17178);
#15109=PLANE('',#17179);
#15110=PLANE('',#17180);
#15111=PLANE('',#17181);
#15112=PLANE('',#17182);
#15113=PLANE('',#17183);
#15114=PLANE('',#17184);
#15115=PLANE('',#17185);
#15116=PLANE('',#17186);
#15117=PLANE('',#17187);
#15118=PLANE('',#17188);
#15119=PLANE('',#17189);
#15120=PLANE('',#17190);
#15121=PLANE('',#17191);
#15122=PLANE('',#17192);
#15123=PLANE('',#17193);
#15124=PLANE('',#17194);
#15125=PLANE('',#17195);
#15126=PLANE('',#17196);
#15127=PLANE('',#17197);
#15128=PLANE('',#17198);
#15129=PLANE('',#17199);
#15130=PLANE('',#17200);
#15131=PLANE('',#17201);
#15132=PLANE('',#17202);
#15133=PLANE('',#17203);
#15134=PLANE('',#17204);
#15135=PLANE('',#17205);
#15136=PLANE('',#17206);
#15137=PLANE('',#17207);
#15138=PLANE('',#17208);
#15139=PLANE('',#17209);
#15140=PLANE('',#17210);
#15141=PLANE('',#17211);
#15142=PLANE('',#17212);
#15143=PLANE('',#17213);
#15144=PLANE('',#17214);
#15145=PLANE('',#17215);
#15146=PLANE('',#17216);
#15147=PLANE('',#17217);
#15148=PLANE('',#17218);
#15149=PLANE('',#17219);
#15150=PLANE('',#17220);
#15151=PLANE('',#17221);
#15152=PLANE('',#17222);
#15153=PLANE('',#17315);
#15154=PLANE('',#17320);
#15155=PLANE('',#17323);
#15775=ADVANCED_FACE('',(#2232),#949,.T.);
#15776=ADVANCED_FACE('',(#2233),#950,.T.);
#15777=ADVANCED_FACE('',(#2234),#951,.T.);
#15778=ADVANCED_FACE('',(#2235),#952,.T.);
#15779=ADVANCED_FACE('',(#2236),#953,.T.);
#15780=ADVANCED_FACE('',(#2237),#954,.T.);
#15781=ADVANCED_FACE('',(#2238),#955,.T.);
#15782=ADVANCED_FACE('',(#2239),#956,.T.);
#15783=ADVANCED_FACE('',(#2240),#957,.T.);
#15784=ADVANCED_FACE('',(#2241),#958,.T.);
#15785=ADVANCED_FACE('',(#2242),#959,.T.);
#15786=ADVANCED_FACE('',(#2243),#960,.T.);
#15787=ADVANCED_FACE('',(#2244),#961,.T.);
#15788=ADVANCED_FACE('',(#2245),#962,.T.);
#15789=ADVANCED_FACE('',(#2246),#963,.T.);
#15790=ADVANCED_FACE('',(#2247),#964,.T.);
#15791=ADVANCED_FACE('',(#2248),#965,.T.);
#15792=ADVANCED_FACE('',(#2249),#966,.T.);
#15793=ADVANCED_FACE('',(#2250),#967,.T.);
#15794=ADVANCED_FACE('',(#2251),#968,.T.);
#15795=ADVANCED_FACE('',(#2252),#969,.T.);
#15796=ADVANCED_FACE('',(#2253),#970,.T.);
#15797=ADVANCED_FACE('',(#2254),#971,.T.);
#15798=ADVANCED_FACE('',(#2255),#972,.T.);
#15799=ADVANCED_FACE('',(#2256),#973,.T.);
#15800=ADVANCED_FACE('',(#2257),#974,.T.);
#15801=ADVANCED_FACE('',(#2258),#975,.T.);
#15802=ADVANCED_FACE('',(#2259),#976,.T.);
#15803=ADVANCED_FACE('',(#2260),#977,.T.);
#15804=ADVANCED_FACE('',(#2261),#978,.T.);
#15805=ADVANCED_FACE('',(#2262),#979,.T.);
#15806=ADVANCED_FACE('',(#2263),#980,.T.);
#15807=ADVANCED_FACE('',(#2264),#981,.T.);
#15808=ADVANCED_FACE('',(#2265),#982,.T.);
#15809=ADVANCED_FACE('',(#2266),#983,.T.);
#15810=ADVANCED_FACE('',(#2267),#984,.T.);
#15811=ADVANCED_FACE('',(#2268),#985,.T.);
#15812=ADVANCED_FACE('',(#2269),#986,.T.);
#15813=ADVANCED_FACE('',(#2270),#987,.T.);
#15814=ADVANCED_FACE('',(#2271),#988,.T.);
#15815=ADVANCED_FACE('',(#2272),#989,.T.);
#15816=ADVANCED_FACE('',(#2273),#990,.T.);
#15817=ADVANCED_FACE('',(#2274),#991,.T.);
#15818=ADVANCED_FACE('',(#2275),#992,.T.);
#15819=ADVANCED_FACE('',(#2276),#993,.T.);
#15820=ADVANCED_FACE('',(#2277),#994,.T.);
#15821=ADVANCED_FACE('',(#2278),#995,.T.);
#15822=ADVANCED_FACE('',(#2279),#15086,.F.);
#15823=ADVANCED_FACE('',(#2280),#15087,.F.);
#15824=ADVANCED_FACE('',(#2281),#15088,.F.);
#15825=ADVANCED_FACE('',(#2282),#15089,.F.);
#15826=ADVANCED_FACE('',(#2283),#15090,.F.);
#15827=ADVANCED_FACE('',(#2284),#996,.F.);
#15828=ADVANCED_FACE('',(#2285),#15091,.F.);
#15829=ADVANCED_FACE('',(#2286),#503,.F.);
#15830=ADVANCED_FACE('',(#2287),#15092,.T.);
#15831=ADVANCED_FACE('',(#2288),#997,.T.);
#15832=ADVANCED_FACE('',(#2289),#504,.F.);
#15833=ADVANCED_FACE('',(#2290),#15093,.F.);
#15834=ADVANCED_FACE('',(#2291),#15094,.F.);
#15835=ADVANCED_FACE('',(#2292),#15095,.F.);
#15836=ADVANCED_FACE('',(#2293),#15096,.F.);
#15837=ADVANCED_FACE('',(#2294),#15097,.F.);
#15838=ADVANCED_FACE('',(#2295),#15098,.F.);
#15839=ADVANCED_FACE('',(#2296),#15099,.F.);
#15840=ADVANCED_FACE('',(#2297),#15100,.F.);
#15841=ADVANCED_FACE('',(#2298),#15101,.F.);
#15842=ADVANCED_FACE('',(#2299),#15102,.F.);
#15843=ADVANCED_FACE('',(#2300),#15103,.F.);
#15844=ADVANCED_FACE('',(#2301),#15104,.F.);
#15845=ADVANCED_FACE('',(#2302),#15105,.F.);
#15846=ADVANCED_FACE('',(#2303),#15106,.F.);
#15847=ADVANCED_FACE('',(#2304),#15107,.F.);
#15848=ADVANCED_FACE('',(#2305),#15108,.F.);
#15849=ADVANCED_FACE('',(#2306),#15109,.F.);
#15850=ADVANCED_FACE('',(#2307),#15110,.F.);
#15851=ADVANCED_FACE('',(#2308),#15111,.F.);
#15852=ADVANCED_FACE('',(#2309),#15112,.F.);
#15853=ADVANCED_FACE('',(#2310),#15113,.F.);
#15854=ADVANCED_FACE('',(#2311),#15114,.F.);
#15855=ADVANCED_FACE('',(#2312),#15115,.F.);
#15856=ADVANCED_FACE('',(#2313),#15116,.F.);
#15857=ADVANCED_FACE('',(#2314),#15117,.F.);
#15858=ADVANCED_FACE('',(#2315),#15118,.F.);
#15859=ADVANCED_FACE('',(#2316),#15119,.F.);
#15860=ADVANCED_FACE('',(#2317),#15120,.F.);
#15861=ADVANCED_FACE('',(#2318),#15121,.F.);
#15862=ADVANCED_FACE('',(#2319),#15122,.F.);
#15863=ADVANCED_FACE('',(#2320),#15123,.F.);
#15864=ADVANCED_FACE('',(#2321),#15124,.F.);
#15865=ADVANCED_FACE('',(#2322),#15125,.F.);
#15866=ADVANCED_FACE('',(#2323),#15126,.F.);
#15867=ADVANCED_FACE('',(#2324),#15127,.F.);
#15868=ADVANCED_FACE('',(#2325),#15128,.F.);
#15869=ADVANCED_FACE('',(#2326),#15129,.F.);
#15870=ADVANCED_FACE('',(#2327),#15130,.F.);
#15871=ADVANCED_FACE('',(#2328),#15131,.F.);
#15872=ADVANCED_FACE('',(#2329),#15132,.F.);
#15873=ADVANCED_FACE('',(#2330),#15133,.F.);
#15874=ADVANCED_FACE('',(#2331),#15134,.F.);
#15875=ADVANCED_FACE('',(#2332),#15135,.F.);
#15876=ADVANCED_FACE('',(#2333),#15136,.F.);
#15877=ADVANCED_FACE('',(#2334),#15137,.F.);
#15878=ADVANCED_FACE('',(#2335),#15138,.F.);
#15879=ADVANCED_FACE('',(#2336),#15139,.F.);
#15880=ADVANCED_FACE('',(#2337),#15140,.F.);
#15881=ADVANCED_FACE('',(#2338),#15141,.F.);
#15882=ADVANCED_FACE('',(#2339),#15142,.F.);
#15883=ADVANCED_FACE('',(#2340),#15143,.F.);
#15884=ADVANCED_FACE('',(#2341),#15144,.F.);
#15885=ADVANCED_FACE('',(#2342),#15145,.F.);
#15886=ADVANCED_FACE('',(#2343),#15146,.F.);
#15887=ADVANCED_FACE('',(#2344),#15147,.F.);
#15888=ADVANCED_FACE('',(#2345),#15148,.F.);
#15889=ADVANCED_FACE('',(#2346),#15149,.F.);
#15890=ADVANCED_FACE('',(#2347),#15150,.F.);
#15891=ADVANCED_FACE('',(#2348),#15151,.F.);
#15892=ADVANCED_FACE('',(#2349),#15152,.F.);
#15893=ADVANCED_FACE('',(#2350),#998,.T.);
#15894=ADVANCED_FACE('',(#2351),#999,.T.);
#15895=ADVANCED_FACE('',(#2352),#1000,.T.);
#15896=ADVANCED_FACE('',(#2353),#1001,.T.);
#15897=ADVANCED_FACE('',(#2354),#1002,.T.);
#15898=ADVANCED_FACE('',(#2355),#1003,.T.);
#15899=ADVANCED_FACE('',(#2356),#1004,.T.);
#15900=ADVANCED_FACE('',(#2357),#1005,.T.);
#15901=ADVANCED_FACE('',(#2358),#1006,.T.);
#15902=ADVANCED_FACE('',(#2359),#1007,.T.);
#15903=ADVANCED_FACE('',(#2360),#1008,.T.);
#15904=ADVANCED_FACE('',(#2361),#1009,.T.);
#15905=ADVANCED_FACE('',(#2362),#1010,.T.);
#15906=ADVANCED_FACE('',(#2363),#1011,.T.);
#15907=ADVANCED_FACE('',(#2364),#1012,.T.);
#15908=ADVANCED_FACE('',(#2365),#1013,.T.);
#15909=ADVANCED_FACE('',(#2366),#1014,.T.);
#15910=ADVANCED_FACE('',(#2367),#1015,.T.);
#15911=ADVANCED_FACE('',(#2368),#1016,.T.);
#15912=ADVANCED_FACE('',(#2369),#1017,.T.);
#15913=ADVANCED_FACE('',(#2370),#1018,.T.);
#15914=ADVANCED_FACE('',(#2371),#1019,.T.);
#15915=ADVANCED_FACE('',(#2372),#1020,.T.);
#15916=ADVANCED_FACE('',(#2373),#1021,.T.);
#15917=ADVANCED_FACE('',(#2374),#1022,.T.);
#15918=ADVANCED_FACE('',(#2375),#1023,.T.);
#15919=ADVANCED_FACE('',(#2376),#1024,.T.);
#15920=ADVANCED_FACE('',(#2377),#1025,.T.);
#15921=ADVANCED_FACE('',(#2378),#1026,.T.);
#15922=ADVANCED_FACE('',(#2379),#1027,.T.);
#15923=ADVANCED_FACE('',(#2380),#1765,.T.);
#15924=ADVANCED_FACE('',(#2381,#1199),#15153,.T.);
#15925=ADVANCED_FACE('',(#2382),#1766,.T.);
#15926=ADVANCED_FACE('',(#2383),#1028,.T.);
#15927=ADVANCED_FACE('',(#2384,#1200),#15154,.T.);
#15928=ADVANCED_FACE('',(#2385),#1767,.T.);
#15929=ADVANCED_FACE('',(#2386,#1201),#15155,.T.);
#16243=CLOSED_SHELL('',(#15775,#15776,#15777,#15778,#15779,#15780,#15781,
#15782,#15783,#15784,#15785,#15786,#15787,#15788,#15789,#15790,#15791,#15792,
#15793,#15794,#15795,#15796,#15797,#15798,#15799,#15800,#15801,#15802,#15803,
#15804,#15805,#15806,#15807,#15808,#15809,#15810,#15811,#15812,#15813,#15814,
#15815,#15816,#15817,#15818,#15819,#15820,#15821,#15822,#15823,#15824,#15825,
#15826,#15827,#15828,#15829,#15830,#15831,#15832,#15833,#15834,#15835,#15836,
#15837,#15838,#15839,#15840,#15841,#15842,#15843,#15844,#15845,#15846,#15847,
#15848,#15849,#15850,#15851,#15852,#15853,#15854,#15855,#15856,#15857,#15858,
#15859,#15860,#15861,#15862,#15863,#15864,#15865,#15866,#15867,#15868,#15869,
#15870,#15871,#15872,#15873,#15874,#15875,#15876,#15877,#15878,#15879,#15880,
#15881,#15882,#15883,#15884,#15885,#15886,#15887,#15888,#15889,#15890,#15891,
#15892,#15893,#15894,#15895,#15896,#15897,#15898,#15899,#15900,#15901,#15902,
#15903,#15904,#15905,#15906,#15907,#15908,#15909,#15910,#15911,#15912,#15913,
#15914,#15915,#15916,#15917,#15918,#15919,#15920,#15921,#15922,#15923,#15924,
#15925,#15926,#15927,#15928,#15929));
#17098=AXIS2_PLACEMENT_3D('',#27584,#19906,#19907);
#17099=AXIS2_PLACEMENT_3D('',#27585,#19908,#19909);
#17100=AXIS2_PLACEMENT_3D('',#27601,#19911,#19912);
#17101=AXIS2_PLACEMENT_3D('',#27609,#19913,#19914);
#17102=AXIS2_PLACEMENT_3D('',#27657,#19916,#19917);
#17103=AXIS2_PLACEMENT_3D('',#27705,#19919,#19920);
#17104=AXIS2_PLACEMENT_3D('',#27759,#19922,#19923);
#17105=AXIS2_PLACEMENT_3D('',#27807,#19925,#19926);
#17106=AXIS2_PLACEMENT_3D('',#27855,#19928,#19929);
#17107=AXIS2_PLACEMENT_3D('',#27903,#19931,#19932);
#17108=AXIS2_PLACEMENT_3D('',#27954,#19934,#19935);
#17109=AXIS2_PLACEMENT_3D('',#28002,#19937,#19938);
#17110=AXIS2_PLACEMENT_3D('',#28050,#19940,#19941);
#17111=AXIS2_PLACEMENT_3D('',#28104,#19943,#19944);
#17112=AXIS2_PLACEMENT_3D('',#28152,#19946,#19947);
#17113=AXIS2_PLACEMENT_3D('',#28200,#19949,#19950);
#17114=AXIS2_PLACEMENT_3D('',#28254,#19952,#19953);
#17115=AXIS2_PLACEMENT_3D('',#28302,#19955,#19956);
#17116=AXIS2_PLACEMENT_3D('',#28350,#19958,#19959);
#17117=AXIS2_PLACEMENT_3D('',#28404,#19961,#19962);
#17118=AXIS2_PLACEMENT_3D('',#28452,#19964,#19965);
#17119=AXIS2_PLACEMENT_3D('',#28500,#19967,#19968);
#17120=AXIS2_PLACEMENT_3D('',#28554,#19970,#19971);
#17121=AXIS2_PLACEMENT_3D('',#28602,#19973,#19974);
#17122=AXIS2_PLACEMENT_3D('',#28650,#19976,#19977);
#17123=AXIS2_PLACEMENT_3D('',#28701,#19979,#19980);
#17124=AXIS2_PLACEMENT_3D('',#28706,#19982,#19983);
#17125=AXIS2_PLACEMENT_3D('',#28751,#19984,#19985);
#17126=AXIS2_PLACEMENT_3D('',#28765,#19987,#19988);
#17127=AXIS2_PLACEMENT_3D('',#28772,#19989,#19990);
#17128=AXIS2_PLACEMENT_3D('',#28796,#19992,#19993);
#17129=AXIS2_PLACEMENT_3D('',#28821,#19995,#19996);
#17130=AXIS2_PLACEMENT_3D('',#28845,#19998,#19999);
#17131=AXIS2_PLACEMENT_3D('',#28870,#20001,#20002);
#17132=AXIS2_PLACEMENT_3D('',#28895,#20004,#20005);
#17133=AXIS2_PLACEMENT_3D('',#28919,#20007,#20008);
#17134=AXIS2_PLACEMENT_3D('',#28944,#20010,#20011);
#17135=AXIS2_PLACEMENT_3D('',#28969,#20013,#20014);
#17136=AXIS2_PLACEMENT_3D('',#28993,#20016,#20017);
#17137=AXIS2_PLACEMENT_3D('',#29018,#20019,#20020);
#17138=AXIS2_PLACEMENT_3D('',#29043,#20022,#20023);
#17139=AXIS2_PLACEMENT_3D('',#29067,#20025,#20026);
#17140=AXIS2_PLACEMENT_3D('',#29092,#20028,#20029);
#17141=AXIS2_PLACEMENT_3D('',#29117,#20031,#20032);
#17142=AXIS2_PLACEMENT_3D('',#29141,#20034,#20035);
#17143=AXIS2_PLACEMENT_3D('',#29166,#20037,#20038);
#17144=AXIS2_PLACEMENT_3D('',#29190,#20040,#20041);
#17145=AXIS2_PLACEMENT_3D('',#29215,#20043,#20044);
#17146=AXIS2_PLACEMENT_3D('',#29239,#20046,#20047);
#17147=AXIS2_PLACEMENT_3D('',#29264,#20049,#20050);
#17148=AXIS2_PLACEMENT_3D('',#29289,#20052,#20053);
#17149=AXIS2_PLACEMENT_3D('',#29313,#20055,#20056);
#17150=AXIS2_PLACEMENT_3D('',#29322,#20061,#20062);
#17151=AXIS2_PLACEMENT_3D('',#29328,#20066,#20067);
#17152=AXIS2_PLACEMENT_3D('',#29334,#20071,#20072);
#17153=AXIS2_PLACEMENT_3D('',#29337,#20075,#20076);
#17154=AXIS2_PLACEMENT_3D('',#29338,#20077,#20078);
#17155=AXIS2_PLACEMENT_3D('',#29340,#20079,#20080);
#17156=AXIS2_PLACEMENT_3D('',#29343,#20082,#20083);
#17157=AXIS2_PLACEMENT_3D('',#29344,#20084,#20085);
#17158=AXIS2_PLACEMENT_3D('',#30078,#20086,#20087);
#17159=AXIS2_PLACEMENT_3D('',#30080,#20088,#20089);
#17160=AXIS2_PLACEMENT_3D('',#30081,#20090,#20091);
#17161=AXIS2_PLACEMENT_3D('',#30138,#20092,#20093);
#17162=AXIS2_PLACEMENT_3D('',#30139,#20094,#20095);
#17163=AXIS2_PLACEMENT_3D('',#30811,#20096,#20097);
#17164=AXIS2_PLACEMENT_3D('',#30824,#20100,#20101);
#17165=AXIS2_PLACEMENT_3D('',#30834,#20103,#20104);
#17166=AXIS2_PLACEMENT_3D('',#30847,#20107,#20108);
#17167=AXIS2_PLACEMENT_3D('',#30857,#20110,#20111);
#17168=AXIS2_PLACEMENT_3D('',#30870,#20114,#20115);
#17169=AXIS2_PLACEMENT_3D('',#30880,#20117,#20118);
#17170=AXIS2_PLACEMENT_3D('',#30893,#20121,#20122);
#17171=AXIS2_PLACEMENT_3D('',#30903,#20124,#20125);
#17172=AXIS2_PLACEMENT_3D('',#30916,#20128,#20129);
#17173=AXIS2_PLACEMENT_3D('',#30926,#20131,#20132);
#17174=AXIS2_PLACEMENT_3D('',#30939,#20135,#20136);
#17175=AXIS2_PLACEMENT_3D('',#30949,#20138,#20139);
#17176=AXIS2_PLACEMENT_3D('',#30962,#20142,#20143);
#17177=AXIS2_PLACEMENT_3D('',#30972,#20145,#20146);
#17178=AXIS2_PLACEMENT_3D('',#30985,#20149,#20150);
#17179=AXIS2_PLACEMENT_3D('',#30995,#20152,#20153);
#17180=AXIS2_PLACEMENT_3D('',#31008,#20156,#20157);
#17181=AXIS2_PLACEMENT_3D('',#31018,#20159,#20160);
#17182=AXIS2_PLACEMENT_3D('',#31031,#20163,#20164);
#17183=AXIS2_PLACEMENT_3D('',#31041,#20166,#20167);
#17184=AXIS2_PLACEMENT_3D('',#31054,#20170,#20171);
#17185=AXIS2_PLACEMENT_3D('',#31064,#20173,#20174);
#17186=AXIS2_PLACEMENT_3D('',#31077,#20177,#20178);
#17187=AXIS2_PLACEMENT_3D('',#31087,#20180,#20181);
#17188=AXIS2_PLACEMENT_3D('',#31100,#20184,#20185);
#17189=AXIS2_PLACEMENT_3D('',#31110,#20187,#20188);
#17190=AXIS2_PLACEMENT_3D('',#31123,#20191,#20192);
#17191=AXIS2_PLACEMENT_3D('',#31133,#20194,#20195);
#17192=AXIS2_PLACEMENT_3D('',#31146,#20198,#20199);
#17193=AXIS2_PLACEMENT_3D('',#31156,#20201,#20202);
#17194=AXIS2_PLACEMENT_3D('',#31169,#20205,#20206);
#17195=AXIS2_PLACEMENT_3D('',#31179,#20208,#20209);
#17196=AXIS2_PLACEMENT_3D('',#31192,#20212,#20213);
#17197=AXIS2_PLACEMENT_3D('',#31202,#20215,#20216);
#17198=AXIS2_PLACEMENT_3D('',#31215,#20219,#20220);
#17199=AXIS2_PLACEMENT_3D('',#31225,#20222,#20223);
#17200=AXIS2_PLACEMENT_3D('',#31238,#20226,#20227);
#17201=AXIS2_PLACEMENT_3D('',#31248,#20229,#20230);
#17202=AXIS2_PLACEMENT_3D('',#31261,#20233,#20234);
#17203=AXIS2_PLACEMENT_3D('',#31271,#20236,#20237);
#17204=AXIS2_PLACEMENT_3D('',#31284,#20240,#20241);
#17205=AXIS2_PLACEMENT_3D('',#31294,#20243,#20244);
#17206=AXIS2_PLACEMENT_3D('',#31307,#20247,#20248);
#17207=AXIS2_PLACEMENT_3D('',#31317,#20250,#20251);
#17208=AXIS2_PLACEMENT_3D('',#31330,#20254,#20255);
#17209=AXIS2_PLACEMENT_3D('',#31340,#20257,#20258);
#17210=AXIS2_PLACEMENT_3D('',#31353,#20261,#20262);
#17211=AXIS2_PLACEMENT_3D('',#31363,#20264,#20265);
#17212=AXIS2_PLACEMENT_3D('',#31376,#20268,#20269);
#17213=AXIS2_PLACEMENT_3D('',#31386,#20271,#20272);
#17214=AXIS2_PLACEMENT_3D('',#31399,#20275,#20276);
#17215=AXIS2_PLACEMENT_3D('',#31409,#20278,#20279);
#17216=AXIS2_PLACEMENT_3D('',#31422,#20282,#20283);
#17217=AXIS2_PLACEMENT_3D('',#31432,#20285,#20286);
#17218=AXIS2_PLACEMENT_3D('',#31445,#20289,#20290);
#17219=AXIS2_PLACEMENT_3D('',#31455,#20292,#20293);
#17220=AXIS2_PLACEMENT_3D('',#31468,#20296,#20297);
#17221=AXIS2_PLACEMENT_3D('',#31478,#20299,#20300);
#17222=AXIS2_PLACEMENT_3D('',#31491,#20303,#20304);
#17223=AXIS2_PLACEMENT_3D('',#31501,#20306,#20307);
#17224=AXIS2_PLACEMENT_3D('',#31502,#20308,#20309);
#17225=AXIS2_PLACEMENT_3D('',#31503,#20310,#20311);
#17226=AXIS2_PLACEMENT_3D('',#31504,#20312,#20313);
#17227=AXIS2_PLACEMENT_3D('',#31505,#20314,#20315);
#17228=AXIS2_PLACEMENT_3D('',#31506,#20316,#20317);
#17229=AXIS2_PLACEMENT_3D('',#31507,#20318,#20319);
#17230=AXIS2_PLACEMENT_3D('',#31508,#20320,#20321);
#17231=AXIS2_PLACEMENT_3D('',#31509,#20322,#20323);
#17232=AXIS2_PLACEMENT_3D('',#31510,#20324,#20325);
#17233=AXIS2_PLACEMENT_3D('',#31511,#20326,#20327);
#17234=AXIS2_PLACEMENT_3D('',#31512,#20328,#20329);
#17235=AXIS2_PLACEMENT_3D('',#31513,#20330,#20331);
#17236=AXIS2_PLACEMENT_3D('',#31514,#20332,#20333);
#17237=AXIS2_PLACEMENT_3D('',#31515,#20334,#20335);
#17238=AXIS2_PLACEMENT_3D('',#31516,#20336,#20337);
#17239=AXIS2_PLACEMENT_3D('',#31517,#20338,#20339);
#17240=AXIS2_PLACEMENT_3D('',#31518,#20340,#20341);
#17241=AXIS2_PLACEMENT_3D('',#31519,#20342,#20343);
#17242=AXIS2_PLACEMENT_3D('',#31520,#20344,#20345);
#17243=AXIS2_PLACEMENT_3D('',#31521,#20346,#20347);
#17244=AXIS2_PLACEMENT_3D('',#31522,#20348,#20349);
#17245=AXIS2_PLACEMENT_3D('',#31523,#20350,#20351);
#17246=AXIS2_PLACEMENT_3D('',#31524,#20352,#20353);
#17247=AXIS2_PLACEMENT_3D('',#31525,#20354,#20355);
#17248=AXIS2_PLACEMENT_3D('',#31526,#20356,#20357);
#17249=AXIS2_PLACEMENT_3D('',#31527,#20358,#20359);
#17250=AXIS2_PLACEMENT_3D('',#31528,#20360,#20361);
#17251=AXIS2_PLACEMENT_3D('',#31529,#20362,#20363);
#17252=AXIS2_PLACEMENT_3D('',#31530,#20364,#20365);
#17253=AXIS2_PLACEMENT_3D('',#31531,#20366,#20367);
#17254=AXIS2_PLACEMENT_3D('',#31532,#20368,#20369);
#17255=AXIS2_PLACEMENT_3D('',#31533,#20370,#20371);
#17256=AXIS2_PLACEMENT_3D('',#31534,#20372,#20373);
#17257=AXIS2_PLACEMENT_3D('',#31535,#20374,#20375);
#17258=AXIS2_PLACEMENT_3D('',#31536,#20376,#20377);
#17259=AXIS2_PLACEMENT_3D('',#31537,#20378,#20379);
#17260=AXIS2_PLACEMENT_3D('',#31538,#20380,#20381);
#17261=AXIS2_PLACEMENT_3D('',#31539,#20382,#20383);
#17262=AXIS2_PLACEMENT_3D('',#31540,#20384,#20385);
#17263=AXIS2_PLACEMENT_3D('',#31541,#20386,#20387);
#17264=AXIS2_PLACEMENT_3D('',#31542,#20388,#20389);
#17265=AXIS2_PLACEMENT_3D('',#31543,#20390,#20391);
#17266=AXIS2_PLACEMENT_3D('',#31544,#20392,#20393);
#17267=AXIS2_PLACEMENT_3D('',#31545,#20394,#20395);
#17268=AXIS2_PLACEMENT_3D('',#31546,#20396,#20397);
#17269=AXIS2_PLACEMENT_3D('',#31547,#20398,#20399);
#17270=AXIS2_PLACEMENT_3D('',#31548,#20400,#20401);
#17271=AXIS2_PLACEMENT_3D('',#31549,#20402,#20403);
#17272=AXIS2_PLACEMENT_3D('',#31550,#20404,#20405);
#17273=AXIS2_PLACEMENT_3D('',#31551,#20406,#20407);
#17274=AXIS2_PLACEMENT_3D('',#31552,#20408,#20409);
#17275=AXIS2_PLACEMENT_3D('',#31553,#20410,#20411);
#17276=AXIS2_PLACEMENT_3D('',#31554,#20412,#20413);
#17277=AXIS2_PLACEMENT_3D('',#31555,#20414,#20415);
#17278=AXIS2_PLACEMENT_3D('',#31556,#20416,#20417);
#17279=AXIS2_PLACEMENT_3D('',#31557,#20418,#20419);
#17280=AXIS2_PLACEMENT_3D('',#31558,#20420,#20421);
#17281=AXIS2_PLACEMENT_3D('',#31559,#20422,#20423);
#17282=AXIS2_PLACEMENT_3D('',#31560,#20424,#20425);
#17283=AXIS2_PLACEMENT_3D('',#31561,#20426,#20427);
#17284=AXIS2_PLACEMENT_3D('',#31562,#20428,#20429);
#17285=AXIS2_PLACEMENT_3D('',#31563,#20430,#20431);
#17286=AXIS2_PLACEMENT_3D('',#31564,#20432,#20433);
#17287=AXIS2_PLACEMENT_3D('',#31565,#20434,#20435);
#17288=AXIS2_PLACEMENT_3D('',#31566,#20436,#20437);
#17289=AXIS2_PLACEMENT_3D('',#31567,#20438,#20439);
#17290=AXIS2_PLACEMENT_3D('',#31568,#20440,#20441);
#17291=AXIS2_PLACEMENT_3D('',#31569,#20442,#20443);
#17292=AXIS2_PLACEMENT_3D('',#31570,#20444,#20445);
#17293=AXIS2_PLACEMENT_3D('',#31571,#20446,#20447);
#17294=AXIS2_PLACEMENT_3D('',#31572,#20448,#20449);
#17295=AXIS2_PLACEMENT_3D('',#31573,#20450,#20451);
#17296=AXIS2_PLACEMENT_3D('',#31574,#20452,#20453);
#17297=AXIS2_PLACEMENT_3D('',#31575,#20454,#20455);
#17298=AXIS2_PLACEMENT_3D('',#31576,#20456,#20457);
#17299=AXIS2_PLACEMENT_3D('',#31577,#20458,#20459);
#17300=AXIS2_PLACEMENT_3D('',#31578,#20460,#20461);
#17301=AXIS2_PLACEMENT_3D('',#31579,#20462,#20463);
#17302=AXIS2_PLACEMENT_3D('',#31580,#20464,#20465);
#17303=AXIS2_PLACEMENT_3D('',#31581,#20466,#20467);
#17304=AXIS2_PLACEMENT_3D('',#31582,#20468,#20469);
#17305=AXIS2_PLACEMENT_3D('',#31583,#20470,#20471);
#17306=AXIS2_PLACEMENT_3D('',#31584,#20472,#20473);
#17307=AXIS2_PLACEMENT_3D('',#31585,#20474,#20475);
#17308=AXIS2_PLACEMENT_3D('',#31586,#20476,#20477);
#17309=AXIS2_PLACEMENT_3D('',#31587,#20478,#20479);
#17310=AXIS2_PLACEMENT_3D('',#31588,#20480,#20481);
#17311=AXIS2_PLACEMENT_3D('',#31589,#20482,#20483);
#17312=AXIS2_PLACEMENT_3D('',#31590,#20484,#20485);
#17313=AXIS2_PLACEMENT_3D('',#31591,#20486,#20487);
#17314=AXIS2_PLACEMENT_3D('',#31594,#20489,#20490);
#17315=AXIS2_PLACEMENT_3D('',#31595,#20491,#20492);
#17316=AXIS2_PLACEMENT_3D('',#31597,#20493,#20494);
#17317=AXIS2_PLACEMENT_3D('',#31598,#20495,#20496);
#17318=AXIS2_PLACEMENT_3D('',#31600,#20498,#20499);
#17319=AXIS2_PLACEMENT_3D('',#31601,#20500,#20501);
#17320=AXIS2_PLACEMENT_3D('',#31602,#20502,#20503);
#17321=AXIS2_PLACEMENT_3D('',#31603,#20504,#20505);
#17322=AXIS2_PLACEMENT_3D('',#31605,#20506,#20507);
#17323=AXIS2_PLACEMENT_3D('',#31607,#20509,#20510);
#19906=DIRECTION('axis',(0.,0.,1.));
#19907=DIRECTION('refdir',(1.,0.,0.));
#19908=DIRECTION('center_axis',(0.,0.,1.));
#19909=DIRECTION('ref_axis',(1.,0.,0.));
#19910=DIRECTION('',(0.,0.,-1.));
#19911=DIRECTION('center_axis',(0.,0.,1.));
#19912=DIRECTION('ref_axis',(1.,0.,0.));
#19913=DIRECTION('center_axis',(0.,0.,1.));
#19914=DIRECTION('ref_axis',(1.,0.,0.));
#19915=DIRECTION('',(0.,0.,-1.));
#19916=DIRECTION('center_axis',(0.,0.,1.));
#19917=DIRECTION('ref_axis',(1.,0.,0.));
#19918=DIRECTION('',(0.,0.,-1.));
#19919=DIRECTION('center_axis',(0.,0.,1.));
#19920=DIRECTION('ref_axis',(1.,0.,0.));
#19921=DIRECTION('',(0.,0.,-1.));
#19922=DIRECTION('center_axis',(0.,0.,1.));
#19923=DIRECTION('ref_axis',(1.,0.,0.));
#19924=DIRECTION('',(0.,0.,-1.));
#19925=DIRECTION('center_axis',(0.,0.,1.));
#19926=DIRECTION('ref_axis',(1.,0.,0.));
#19927=DIRECTION('',(0.,0.,-1.));
#19928=DIRECTION('center_axis',(0.,0.,1.));
#19929=DIRECTION('ref_axis',(1.,0.,0.));
#19930=DIRECTION('',(0.,0.,-1.));
#19931=DIRECTION('center_axis',(0.,0.,1.));
#19932=DIRECTION('ref_axis',(1.,0.,0.));
#19933=DIRECTION('',(0.,0.,-1.));
#19934=DIRECTION('center_axis',(0.,0.,1.));
#19935=DIRECTION('ref_axis',(1.,0.,0.));
#19936=DIRECTION('',(0.,0.,-1.));
#19937=DIRECTION('center_axis',(0.,0.,1.));
#19938=DIRECTION('ref_axis',(1.,0.,0.));
#19939=DIRECTION('',(0.,0.,-1.));
#19940=DIRECTION('center_axis',(0.,0.,1.));
#19941=DIRECTION('ref_axis',(1.,0.,0.));
#19942=DIRECTION('',(0.,0.,-1.));
#19943=DIRECTION('center_axis',(0.,0.,1.));
#19944=DIRECTION('ref_axis',(1.,0.,0.));
#19945=DIRECTION('',(0.,0.,-1.));
#19946=DIRECTION('center_axis',(0.,0.,1.));
#19947=DIRECTION('ref_axis',(1.,0.,0.));
#19948=DIRECTION('',(0.,0.,-1.));
#19949=DIRECTION('center_axis',(0.,0.,1.));
#19950=DIRECTION('ref_axis',(1.,0.,0.));
#19951=DIRECTION('',(0.,0.,-1.));
#19952=DIRECTION('center_axis',(0.,0.,1.));
#19953=DIRECTION('ref_axis',(1.,0.,0.));
#19954=DIRECTION('',(0.,0.,-1.));
#19955=DIRECTION('center_axis',(0.,0.,1.));
#19956=DIRECTION('ref_axis',(1.,0.,0.));
#19957=DIRECTION('',(0.,0.,-1.));
#19958=DIRECTION('center_axis',(0.,0.,1.));
#19959=DIRECTION('ref_axis',(1.,0.,0.));
#19960=DIRECTION('',(0.,0.,-1.));
#19961=DIRECTION('center_axis',(0.,0.,1.));
#19962=DIRECTION('ref_axis',(1.,0.,0.));
#19963=DIRECTION('',(0.,0.,-1.));
#19964=DIRECTION('center_axis',(0.,0.,1.));
#19965=DIRECTION('ref_axis',(1.,0.,0.));
#19966=DIRECTION('',(0.,0.,-1.));
#19967=DIRECTION('center_axis',(0.,0.,1.));
#19968=DIRECTION('ref_axis',(1.,0.,0.));
#19969=DIRECTION('',(0.,0.,-1.));
#19970=DIRECTION('center_axis',(0.,0.,1.));
#19971=DIRECTION('ref_axis',(1.,0.,0.));
#19972=DIRECTION('',(0.,0.,-1.));
#19973=DIRECTION('center_axis',(0.,0.,1.));
#19974=DIRECTION('ref_axis',(1.,0.,0.));
#19975=DIRECTION('',(0.,0.,-1.));
#19976=DIRECTION('center_axis',(0.,0.,1.));
#19977=DIRECTION('ref_axis',(1.,0.,0.));
#19978=DIRECTION('',(0.,0.,-1.));
#19979=DIRECTION('center_axis',(0.,0.,1.));
#19980=DIRECTION('ref_axis',(1.,0.,0.));
#19981=DIRECTION('',(0.,0.,-1.));
#19982=DIRECTION('center_axis',(0.,0.,1.));
#19983=DIRECTION('ref_axis',(1.,0.,0.));
#19984=DIRECTION('center_axis',(0.,0.,1.));
#19985=DIRECTION('ref_axis',(0.37267613439428,-0.927961474875405,0.));
#19986=DIRECTION('',(0.,0.,1.));
#19987=DIRECTION('center_axis',(0.,0.,1.));
#19988=DIRECTION('ref_axis',(1.,-7.76068732292971E-15,0.));
#19989=DIRECTION('center_axis',(0.,0.,1.));
#19990=DIRECTION('ref_axis',(1.,-7.76068732292971E-15,0.));
#19991=DIRECTION('',(0.,0.,1.));
#19992=DIRECTION('center_axis',(0.,0.,1.));
#19993=DIRECTION('ref_axis',(1.,-7.76068732292971E-15,0.));
#19994=DIRECTION('',(0.,0.,1.));
#19995=DIRECTION('center_axis',(0.,0.,1.));
#19996=DIRECTION('ref_axis',(1.,-7.76068732292971E-15,0.));
#19997=DIRECTION('',(0.,0.,1.));
#19998=DIRECTION('center_axis',(0.,0.,1.));
#19999=DIRECTION('ref_axis',(1.,-7.76068732292971E-15,0.));
#20000=DIRECTION('',(0.,0.,1.));
#20001=DIRECTION('center_axis',(0.,0.,1.));
#20002=DIRECTION('ref_axis',(1.,-7.76068732292971E-15,0.));
#20003=DIRECTION('',(0.,0.,1.));
#20004=DIRECTION('center_axis',(0.,0.,1.));
#20005=DIRECTION('ref_axis',(1.,-7.76068732292971E-15,0.));
#20006=DIRECTION('',(0.,0.,1.));
#20007=DIRECTION('center_axis',(0.,0.,1.));
#20008=DIRECTION('ref_axis',(1.,-7.76068732292971E-15,0.));
#20009=DIRECTION('',(0.,0.,1.));
#20010=DIRECTION('center_axis',(0.,0.,1.));
#20011=DIRECTION('ref_axis',(1.,-7.76068732292971E-15,0.));
#20012=DIRECTION('',(0.,0.,1.));
#20013=DIRECTION('center_axis',(0.,0.,1.));
#20014=DIRECTION('ref_axis',(1.,-7.76068732292971E-15,0.));
#20015=DIRECTION('',(0.,0.,1.));
#20016=DIRECTION('center_axis',(0.,0.,1.));
#20017=DIRECTION('ref_axis',(1.,-7.76068732292971E-15,0.));
#20018=DIRECTION('',(0.,0.,1.));
#20019=DIRECTION('center_axis',(0.,0.,1.));
#20020=DIRECTION('ref_axis',(1.,-7.76068732292971E-15,0.));
#20021=DIRECTION('',(0.,0.,1.));
#20022=DIRECTION('center_axis',(0.,0.,1.));
#20023=DIRECTION('ref_axis',(1.,-7.76068732292971E-15,0.));
#20024=DIRECTION('',(0.,0.,1.));
#20025=DIRECTION('center_axis',(0.,0.,1.));
#20026=DIRECTION('ref_axis',(1.,-7.76068732292971E-15,0.));
#20027=DIRECTION('',(0.,0.,1.));
#20028=DIRECTION('center_axis',(0.,0.,1.));
#20029=DIRECTION('ref_axis',(1.,-7.76068732292971E-15,0.));
#20030=DIRECTION('',(0.,0.,1.));
#20031=DIRECTION('center_axis',(0.,0.,1.));
#20032=DIRECTION('ref_axis',(1.,-7.76068732292971E-15,0.));
#20033=DIRECTION('',(0.,0.,1.));
#20034=DIRECTION('center_axis',(0.,0.,1.));
#20035=DIRECTION('ref_axis',(1.,-7.76068732292971E-15,0.));
#20036=DIRECTION('',(0.,0.,1.));
#20037=DIRECTION('center_axis',(0.,0.,1.));
#20038=DIRECTION('ref_axis',(1.,-7.76068732292971E-15,0.));
#20039=DIRECTION('',(0.,0.,1.));
#20040=DIRECTION('center_axis',(0.,0.,1.));
#20041=DIRECTION('ref_axis',(1.,-7.76068732292971E-15,0.));
#20042=DIRECTION('',(0.,0.,1.));
#20043=DIRECTION('center_axis',(0.,0.,1.));
#20044=DIRECTION('ref_axis',(1.,-7.76068732292971E-15,0.));
#20045=DIRECTION('',(0.,0.,1.));
#20046=DIRECTION('center_axis',(0.,0.,1.));
#20047=DIRECTION('ref_axis',(1.,-7.76068732292971E-15,0.));
#20048=DIRECTION('',(0.,0.,1.));
#20049=DIRECTION('center_axis',(0.,0.,1.));
#20050=DIRECTION('ref_axis',(1.,-7.76068732292971E-15,0.));
#20051=DIRECTION('',(0.,0.,1.));
#20052=DIRECTION('center_axis',(0.,0.,1.));
#20053=DIRECTION('ref_axis',(1.,-7.76068732292971E-15,0.));
#20054=DIRECTION('',(0.,0.,1.));
#20055=DIRECTION('center_axis',(0.,-1.,0.));
#20056=DIRECTION('ref_axis',(-1.,0.,0.));
#20057=DIRECTION('',(-1.,0.,0.));
#20058=DIRECTION('',(0.,0.,-1.));
#20059=DIRECTION('',(-1.,0.,0.));
#20060=DIRECTION('',(0.,0.,-1.));
#20061=DIRECTION('center_axis',(1.,0.,0.));
#20062=DIRECTION('ref_axis',(0.,-1.,0.));
#20063=DIRECTION('',(0.,-1.,0.));
#20064=DIRECTION('',(0.,0.,-1.));
#20065=DIRECTION('',(0.,-1.,0.));
#20066=DIRECTION('center_axis',(0.,1.,0.));
#20067=DIRECTION('ref_axis',(1.,0.,0.));
#20068=DIRECTION('',(1.,0.,0.));
#20069=DIRECTION('',(0.,0.,-1.));
#20070=DIRECTION('',(1.,0.,0.));
#20071=DIRECTION('center_axis',(-1.,0.,0.));
#20072=DIRECTION('ref_axis',(0.,1.,0.));
#20073=DIRECTION('',(0.,1.,0.));
#20074=DIRECTION('',(0.,1.,0.));
#20075=DIRECTION('center_axis',(0.,0.,-1.));
#20076=DIRECTION('ref_axis',(-1.,0.,0.));
#20077=DIRECTION('center_axis',(0.,0.,1.));
#20078=DIRECTION('ref_axis',(1.,0.,0.));
#20079=DIRECTION('center_axis',(0.,0.,1.));
#20080=DIRECTION('ref_axis',(1.,0.,0.));
#20081=DIRECTION('',(0.,0.,1.));
#20082=DIRECTION('center_axis',(0.,0.,1.));
#20083=DIRECTION('ref_axis',(1.,0.,0.));
#20084=DIRECTION('center_axis',(0.,0.,1.));
#20085=DIRECTION('ref_axis',(1.,0.,0.));
#20086=DIRECTION('center_axis',(0.,0.,1.));
#20087=DIRECTION('ref_axis',(1.,0.,0.));
#20088=DIRECTION('center_axis',(0.,0.,1.));
#20089=DIRECTION('ref_axis',(1.,0.,0.));
#20090=DIRECTION('center_axis',(0.,0.,1.));
#20091=DIRECTION('ref_axis',(1.,0.,0.));
#20092=DIRECTION('center_axis',(0.,0.,-1.));
#20093=DIRECTION('ref_axis',(1.,-7.76068732292971E-15,0.));
#20094=DIRECTION('center_axis',(0.,0.,1.));
#20095=DIRECTION('ref_axis',(1.,-7.76068732292971E-15,0.));
#20096=DIRECTION('center_axis',(-0.0382353162534336,0.999268762941682,0.));
#20097=DIRECTION('ref_axis',(0.999268762941682,0.0382353162534336,0.));
#20098=DIRECTION('',(0.,0.,-1.));
#20099=DIRECTION('',(0.,0.,-1.));
#20100=DIRECTION('center_axis',(-0.768185830790291,-0.640226935838403,0.));
#20101=DIRECTION('ref_axis',(-0.640226935838403,0.768185830790291,0.));
#20102=DIRECTION('',(0.,0.,1.));
#20103=DIRECTION('center_axis',(0.371509522684555,0.928429143529378,0.));
#20104=DIRECTION('ref_axis',(0.928429143529378,-0.371509522684555,0.));
#20105=DIRECTION('',(0.,0.,-1.));
#20106=DIRECTION('',(0.,0.,-1.));
#20107=DIRECTION('center_axis',(-0.962176431033494,-0.272427083021583,0.));
#20108=DIRECTION('ref_axis',(-0.272427083021583,0.962176431033494,0.));
#20109=DIRECTION('',(0.,0.,1.));
#20110=DIRECTION('center_axis',(0.717016990092325,0.697055690686865,0.));
#20111=DIRECTION('ref_axis',(0.697055690686865,-0.717016990092325,0.));
#20112=DIRECTION('',(0.,0.,-1.));
#20113=DIRECTION('',(0.,0.,-1.));
#20114=DIRECTION('center_axis',(-0.989797985252547,0.142477887372033,0.));
#20115=DIRECTION('ref_axis',(0.142477887372033,0.989797985252547,0.));
#20116=DIRECTION('',(0.,0.,1.));
#20117=DIRECTION('center_axis',(0.938545706018272,0.345154976372445,0.));
#20118=DIRECTION('ref_axis',(0.345154976372445,-0.938545706018272,0.));
#20119=DIRECTION('',(0.,0.,-1.));
#20120=DIRECTION('',(0.,0.,-1.));
#20121=DIRECTION('center_axis',(-0.84627447578903,0.532747136668047,0.));
#20122=DIRECTION('ref_axis',(0.532747136668047,0.84627447578903,0.));
#20123=DIRECTION('',(0.,0.,1.));
#20124=DIRECTION('center_axis',(0.997791342953596,-0.0664261689912929,0.));
#20125=DIRECTION('ref_axis',(-0.0664261689912929,-0.997791342953596,0.));
#20126=DIRECTION('',(0.,0.,-1.));
#20127=DIRECTION('',(0.,0.,-1.));
#20128=DIRECTION('center_axis',(-0.556422421299341,0.830899566178355,0.));
#20129=DIRECTION('ref_axis',(0.830899566178355,0.556422421299341,0.));
#20130=DIRECTION('',(0.,0.,1.));
#20131=DIRECTION('center_axis',(0.884509792042463,-0.466521626273638,0.));
#20132=DIRECTION('ref_axis',(-0.466521626273638,-0.884509792042463,0.));
#20133=DIRECTION('',(0.,0.,-1.));
#20134=DIRECTION('',(0.,0.,-1.));
#20135=DIRECTION('center_axis',(-0.170359875227987,0.985381912210847,0.));
#20136=DIRECTION('ref_axis',(0.985381912210847,0.170359875227987,0.));
#20137=DIRECTION('',(0.,0.,1.));
#20138=DIRECTION('center_axis',(0.618288462567988,-0.785951256157348,0.));
#20139=DIRECTION('ref_axis',(-0.785951256157348,-0.618288462567988,0.));
#20140=DIRECTION('',(0.,0.,-1.));
#20141=DIRECTION('',(0.,0.,-1.));
#20142=DIRECTION('center_axis',(0.245159440941167,0.969482773708442,0.));
#20143=DIRECTION('ref_axis',(0.969482773708442,-0.245159440941167,0.));
#20144=DIRECTION('',(0.,0.,1.));
#20145=DIRECTION('center_axis',(-0.441368921654257,0.897325735169653,0.));
#20146=DIRECTION('ref_axis',(0.897325735169653,0.441368921654257,0.));
#20147=DIRECTION('',(0.,0.,-1.));
#20148=DIRECTION('',(0.,0.,-1.));
#20149=DIRECTION('center_axis',(-0.441368921654257,-0.897325735169653,0.));
#20150=DIRECTION('ref_axis',(-0.897325735169653,0.441368921654257,0.));
#20151=DIRECTION('',(0.,0.,1.));
#20152=DIRECTION('center_axis',(0.0382353162534307,-0.999268762941682,0.));
#20153=DIRECTION('ref_axis',(-0.999268762941682,-0.0382353162534307,0.));
#20154=DIRECTION('',(0.,0.,-1.));
#20155=DIRECTION('',(0.,0.,-1.));
#20156=DIRECTION('center_axis',(0.768185830790288,0.640226935838407,0.));
#20157=DIRECTION('ref_axis',(0.640226935838407,-0.768185830790288,0.));
#20158=DIRECTION('',(0.,0.,1.));
#20159=DIRECTION('center_axis',(-0.37150952268456,-0.928429143529376,0.));
#20160=DIRECTION('ref_axis',(-0.928429143529376,0.37150952268456,0.));
#20161=DIRECTION('',(0.,0.,-1.));
#20162=DIRECTION('',(0.,0.,-1.));
#20163=DIRECTION('center_axis',(0.962176431033495,0.27242708302158,0.));
#20164=DIRECTION('ref_axis',(0.27242708302158,-0.962176431033495,0.));
#20165=DIRECTION('',(0.,0.,1.));
#20166=DIRECTION('center_axis',(-0.717016990092328,-0.697055690686862,0.));
#20167=DIRECTION('ref_axis',(-0.697055690686862,0.717016990092328,0.));
#20168=DIRECTION('',(0.,0.,-1.));
#20169=DIRECTION('',(0.,0.,-1.));
#20170=DIRECTION('center_axis',(0.989797985252548,-0.142477887372029,0.));
#20171=DIRECTION('ref_axis',(-0.142477887372029,-0.989797985252548,0.));
#20172=DIRECTION('',(0.,0.,1.));
#20173=DIRECTION('center_axis',(-0.938545706018274,-0.34515497637244,0.));
#20174=DIRECTION('ref_axis',(-0.34515497637244,0.938545706018274,0.));
#20175=DIRECTION('',(0.,0.,-1.));
#20176=DIRECTION('',(0.,0.,-1.));
#20177=DIRECTION('center_axis',(0.846274475789033,-0.532747136668042,0.));
#20178=DIRECTION('ref_axis',(-0.532747136668042,-0.846274475789033,0.));
#20179=DIRECTION('',(0.,0.,1.));
#20180=DIRECTION('center_axis',(-0.997791342953596,0.0664261689912958,0.));
#20181=DIRECTION('ref_axis',(0.0664261689912958,0.997791342953596,0.));
#20182=DIRECTION('',(0.,0.,-1.));
#20183=DIRECTION('',(0.,0.,-1.));
#20184=DIRECTION('center_axis',(0.556422421299338,-0.830899566178357,0.));
#20185=DIRECTION('ref_axis',(-0.830899566178357,-0.556422421299338,0.));
#20186=DIRECTION('',(0.,0.,1.));
#20187=DIRECTION('center_axis',(-0.884509792042462,0.466521626273638,0.));
#20188=DIRECTION('ref_axis',(0.466521626273638,0.884509792042462,0.));
#20189=DIRECTION('',(0.,0.,-1.));
#20190=DIRECTION('',(0.,0.,-1.));
#20191=DIRECTION('center_axis',(0.170359875227985,-0.985381912210847,0.));
#20192=DIRECTION('ref_axis',(-0.985381912210847,-0.170359875227985,0.));
#20193=DIRECTION('',(0.,0.,1.));
#20194=DIRECTION('center_axis',(-0.61828846256799,0.785951256157347,0.));
#20195=DIRECTION('ref_axis',(0.785951256157347,0.61828846256799,0.));
#20196=DIRECTION('',(0.,0.,-1.));
#20197=DIRECTION('',(0.,0.,-1.));
#20198=DIRECTION('center_axis',(-0.245159440941167,-0.969482773708442,0.));
#20199=DIRECTION('ref_axis',(-0.969482773708442,0.245159440941167,0.));
#20200=DIRECTION('',(0.,0.,1.));
#20201=DIRECTION('center_axis',(-0.768185830790289,0.640226935838406,0.));
#20202=DIRECTION('ref_axis',(0.640226935838406,0.768185830790289,0.));
#20203=DIRECTION('',(0.,0.,-1.));
#20204=DIRECTION('',(0.,0.,-1.));
#20205=DIRECTION('center_axis',(-0.0382353162534311,-0.999268762941682,
0.));
#20206=DIRECTION('ref_axis',(-0.999268762941682,0.0382353162534311,0.));
#20207=DIRECTION('',(0.,0.,1.));
#20208=DIRECTION('center_axis',(-0.962176431033495,0.27242708302158,0.));
#20209=DIRECTION('ref_axis',(0.27242708302158,0.962176431033495,0.));
#20210=DIRECTION('',(0.,0.,-1.));
#20211=DIRECTION('',(0.,0.,-1.));
#20212=DIRECTION('center_axis',(0.371509522684558,-0.928429143529377,0.));
#20213=DIRECTION('ref_axis',(-0.928429143529377,-0.371509522684558,0.));
#20214=DIRECTION('',(0.,0.,1.));
#20215=DIRECTION('center_axis',(-0.989797985252548,-0.142477887372029,0.));
#20216=DIRECTION('ref_axis',(-0.142477887372029,0.989797985252548,0.));
#20217=DIRECTION('',(0.,0.,-1.));
#20218=DIRECTION('',(0.,0.,-1.));
#20219=DIRECTION('center_axis',(0.717016990092329,-0.697055690686861,0.));
#20220=DIRECTION('ref_axis',(-0.697055690686861,-0.717016990092329,0.));
#20221=DIRECTION('',(0.,0.,1.));
#20222=DIRECTION('center_axis',(-0.846274475789033,-0.532747136668042,0.));
#20223=DIRECTION('ref_axis',(-0.532747136668042,0.846274475789033,0.));
#20224=DIRECTION('',(0.,0.,-1.));
#20225=DIRECTION('',(0.,0.,-1.));
#20226=DIRECTION('center_axis',(0.938545706018273,-0.345154976372442,0.));
#20227=DIRECTION('ref_axis',(-0.345154976372442,-0.938545706018273,0.));
#20228=DIRECTION('',(0.,0.,1.));
#20229=DIRECTION('center_axis',(-0.556422421299338,-0.830899566178357,0.));
#20230=DIRECTION('ref_axis',(-0.830899566178357,0.556422421299338,0.));
#20231=DIRECTION('',(0.,0.,-1.));
#20232=DIRECTION('',(0.,0.,-1.));
#20233=DIRECTION('center_axis',(0.997791342953596,0.066426168991298,0.));
#20234=DIRECTION('ref_axis',(0.066426168991298,-0.997791342953596,0.));
#20235=DIRECTION('',(0.,0.,1.));
#20236=DIRECTION('center_axis',(-0.170359875227984,-0.985381912210847,0.));
#20237=DIRECTION('ref_axis',(-0.985381912210847,0.170359875227984,0.));
#20238=DIRECTION('',(0.,0.,-1.));
#20239=DIRECTION('',(0.,0.,-1.));
#20240=DIRECTION('center_axis',(0.884509792042461,0.466521626273641,0.));
#20241=DIRECTION('ref_axis',(0.466521626273641,-0.884509792042461,0.));
#20242=DIRECTION('',(0.,0.,1.));
#20243=DIRECTION('center_axis',(0.245159440941165,-0.969482773708443,0.));
#20244=DIRECTION('ref_axis',(-0.969482773708443,-0.245159440941165,0.));
#20245=DIRECTION('',(0.,0.,-1.));
#20246=DIRECTION('',(0.,0.,-1.));
#20247=DIRECTION('center_axis',(0.618288462567991,0.785951256157346,0.));
#20248=DIRECTION('ref_axis',(0.785951256157346,-0.618288462567991,0.));
#20249=DIRECTION('',(0.,0.,1.));
#20250=DIRECTION('center_axis',(0.441368921654258,-0.897325735169653,0.));
#20251=DIRECTION('ref_axis',(-0.897325735169653,-0.441368921654258,0.));
#20252=DIRECTION('',(0.,0.,-1.));
#20253=DIRECTION('',(0.,0.,-1.));
#20254=DIRECTION('center_axis',(0.441368921654255,0.897325735169654,0.));
#20255=DIRECTION('ref_axis',(0.897325735169654,-0.441368921654255,0.));
#20256=DIRECTION('',(0.,0.,1.));
#20257=DIRECTION('center_axis',(0.768185830790287,-0.640226935838408,0.));
#20258=DIRECTION('ref_axis',(-0.640226935838408,-0.768185830790287,0.));
#20259=DIRECTION('',(0.,0.,-1.));
#20260=DIRECTION('',(0.,0.,-1.));
#20261=DIRECTION('center_axis',(0.0382353162534311,0.999268762941682,0.));
#20262=DIRECTION('ref_axis',(0.999268762941682,-0.0382353162534311,0.));
#20263=DIRECTION('',(0.,0.,1.));
#20264=DIRECTION('center_axis',(0.962176431033494,-0.272427083021581,0.));
#20265=DIRECTION('ref_axis',(-0.272427083021581,-0.962176431033494,0.));
#20266=DIRECTION('',(0.,0.,-1.));
#20267=DIRECTION('',(0.,0.,-1.));
#20268=DIRECTION('center_axis',(-0.371509522684558,0.928429143529377,0.));
#20269=DIRECTION('ref_axis',(0.928429143529377,0.371509522684558,0.));
#20270=DIRECTION('',(0.,0.,1.));
#20271=DIRECTION('center_axis',(0.989797985252548,0.142477887372027,0.));
#20272=DIRECTION('ref_axis',(0.142477887372027,-0.989797985252548,0.));
#20273=DIRECTION('',(0.,0.,-1.));
#20274=DIRECTION('',(0.,0.,-1.));
#20275=DIRECTION('center_axis',(-0.717016990092329,0.697055690686861,0.));
#20276=DIRECTION('ref_axis',(0.697055690686861,0.717016990092329,0.));
#20277=DIRECTION('',(0.,0.,1.));
#20278=DIRECTION('center_axis',(0.84627447578903,0.532747136668047,0.));
#20279=DIRECTION('ref_axis',(0.532747136668047,-0.84627447578903,0.));
#20280=DIRECTION('',(0.,0.,-1.));
#20281=DIRECTION('',(0.,0.,-1.));
#20282=DIRECTION('center_axis',(-0.938545706018274,0.34515497637244,0.));
#20283=DIRECTION('ref_axis',(0.34515497637244,0.938545706018274,0.));
#20284=DIRECTION('',(0.,0.,1.));
#20285=DIRECTION('center_axis',(0.556422421299336,0.830899566178359,0.));
#20286=DIRECTION('ref_axis',(0.830899566178359,-0.556422421299336,0.));
#20287=DIRECTION('',(0.,0.,-1.));
#20288=DIRECTION('',(0.,0.,-1.));
#20289=DIRECTION('center_axis',(-0.997791342953596,-0.0664261689912929,
0.));
#20290=DIRECTION('ref_axis',(-0.0664261689912929,0.997791342953596,0.));
#20291=DIRECTION('',(0.,0.,1.));
#20292=DIRECTION('center_axis',(0.170359875227981,0.985381912210848,0.));
#20293=DIRECTION('ref_axis',(0.985381912210848,-0.170359875227981,0.));
#20294=DIRECTION('',(0.,0.,-1.));
#20295=DIRECTION('',(0.,0.,-1.));
#20296=DIRECTION('center_axis',(-0.884509792042464,-0.466521626273636,0.));
#20297=DIRECTION('ref_axis',(-0.466521626273636,0.884509792042464,0.));
#20298=DIRECTION('',(0.,0.,1.));
#20299=DIRECTION('center_axis',(-0.24515944094117,0.969482773708441,0.));
#20300=DIRECTION('ref_axis',(0.969482773708441,0.24515944094117,0.));
#20301=DIRECTION('',(0.,0.,-1.));
#20302=DIRECTION('',(0.,0.,-1.));
#20303=DIRECTION('center_axis',(-0.618288462567989,-0.785951256157348,0.));
#20304=DIRECTION('ref_axis',(-0.785951256157348,0.618288462567989,0.));
#20305=DIRECTION('',(0.,0.,1.));
#20306=DIRECTION('center_axis',(0.,0.,1.));
#20307=DIRECTION('ref_axis',(1.,0.,0.));
#20308=DIRECTION('center_axis',(0.,0.,1.));
#20309=DIRECTION('ref_axis',(1.,0.,0.));
#20310=DIRECTION('center_axis',(0.,0.,1.));
#20311=DIRECTION('ref_axis',(1.,0.,0.));
#20312=DIRECTION('center_axis',(0.,0.,1.));
#20313=DIRECTION('ref_axis',(1.,0.,0.));
#20314=DIRECTION('center_axis',(0.,0.,1.));
#20315=DIRECTION('ref_axis',(1.,0.,0.));
#20316=DIRECTION('center_axis',(0.,0.,1.));
#20317=DIRECTION('ref_axis',(1.,0.,0.));
#20318=DIRECTION('center_axis',(0.,0.,1.));
#20319=DIRECTION('ref_axis',(1.,0.,0.));
#20320=DIRECTION('center_axis',(0.,0.,1.));
#20321=DIRECTION('ref_axis',(1.,0.,0.));
#20322=DIRECTION('center_axis',(0.,0.,1.));
#20323=DIRECTION('ref_axis',(1.,0.,0.));
#20324=DIRECTION('center_axis',(0.,0.,1.));
#20325=DIRECTION('ref_axis',(1.,0.,0.));
#20326=DIRECTION('center_axis',(0.,0.,1.));
#20327=DIRECTION('ref_axis',(1.,0.,0.));
#20328=DIRECTION('center_axis',(0.,0.,1.));
#20329=DIRECTION('ref_axis',(1.,0.,0.));
#20330=DIRECTION('center_axis',(0.,0.,1.));
#20331=DIRECTION('ref_axis',(1.,0.,0.));
#20332=DIRECTION('center_axis',(0.,0.,1.));
#20333=DIRECTION('ref_axis',(1.,0.,0.));
#20334=DIRECTION('center_axis',(0.,0.,1.));
#20335=DIRECTION('ref_axis',(1.,0.,0.));
#20336=DIRECTION('center_axis',(0.,0.,1.));
#20337=DIRECTION('ref_axis',(1.,0.,0.));
#20338=DIRECTION('center_axis',(0.,0.,1.));
#20339=DIRECTION('ref_axis',(1.,0.,0.));
#20340=DIRECTION('center_axis',(0.,0.,1.));
#20341=DIRECTION('ref_axis',(1.,0.,0.));
#20342=DIRECTION('center_axis',(0.,0.,1.));
#20343=DIRECTION('ref_axis',(1.,0.,0.));
#20344=DIRECTION('center_axis',(0.,0.,1.));
#20345=DIRECTION('ref_axis',(1.,0.,0.));
#20346=DIRECTION('center_axis',(0.,0.,1.));
#20347=DIRECTION('ref_axis',(1.,0.,0.));
#20348=DIRECTION('center_axis',(0.,0.,1.));
#20349=DIRECTION('ref_axis',(1.,0.,0.));
#20350=DIRECTION('center_axis',(0.,0.,1.));
#20351=DIRECTION('ref_axis',(1.,0.,0.));
#20352=DIRECTION('center_axis',(0.,0.,1.));
#20353=DIRECTION('ref_axis',(1.,0.,0.));
#20354=DIRECTION('center_axis',(0.,0.,1.));
#20355=DIRECTION('ref_axis',(1.,0.,0.));
#20356=DIRECTION('center_axis',(0.,0.,1.));
#20357=DIRECTION('ref_axis',(1.,0.,0.));
#20358=DIRECTION('center_axis',(0.,0.,1.));
#20359=DIRECTION('ref_axis',(1.,0.,0.));
#20360=DIRECTION('center_axis',(0.,0.,1.));
#20361=DIRECTION('ref_axis',(1.,0.,0.));
#20362=DIRECTION('center_axis',(0.,0.,1.));
#20363=DIRECTION('ref_axis',(1.,0.,0.));
#20364=DIRECTION('center_axis',(0.,0.,1.));
#20365=DIRECTION('ref_axis',(1.,0.,0.));
#20366=DIRECTION('center_axis',(0.,0.,1.));
#20367=DIRECTION('ref_axis',(1.,0.,0.));
#20368=DIRECTION('center_axis',(0.,0.,1.));
#20369=DIRECTION('ref_axis',(1.,0.,0.));
#20370=DIRECTION('center_axis',(0.,0.,1.));
#20371=DIRECTION('ref_axis',(1.,0.,0.));
#20372=DIRECTION('center_axis',(0.,0.,1.));
#20373=DIRECTION('ref_axis',(1.,0.,0.));
#20374=DIRECTION('center_axis',(0.,0.,1.));
#20375=DIRECTION('ref_axis',(1.,0.,0.));
#20376=DIRECTION('center_axis',(0.,0.,1.));
#20377=DIRECTION('ref_axis',(1.,0.,0.));
#20378=DIRECTION('center_axis',(0.,0.,1.));
#20379=DIRECTION('ref_axis',(1.,0.,0.));
#20380=DIRECTION('center_axis',(0.,0.,1.));
#20381=DIRECTION('ref_axis',(1.,0.,0.));
#20382=DIRECTION('center_axis',(0.,0.,1.));
#20383=DIRECTION('ref_axis',(1.,0.,0.));
#20384=DIRECTION('center_axis',(0.,0.,1.));
#20385=DIRECTION('ref_axis',(1.,0.,0.));
#20386=DIRECTION('center_axis',(0.,0.,1.));
#20387=DIRECTION('ref_axis',(1.,0.,0.));
#20388=DIRECTION('center_axis',(0.,0.,1.));
#20389=DIRECTION('ref_axis',(1.,0.,0.));
#20390=DIRECTION('center_axis',(0.,0.,1.));
#20391=DIRECTION('ref_axis',(1.,0.,0.));
#20392=DIRECTION('center_axis',(0.,0.,1.));
#20393=DIRECTION('ref_axis',(1.,0.,0.));
#20394=DIRECTION('center_axis',(0.,0.,1.));
#20395=DIRECTION('ref_axis',(1.,0.,0.));
#20396=DIRECTION('center_axis',(0.,0.,1.));
#20397=DIRECTION('ref_axis',(1.,0.,0.));
#20398=DIRECTION('center_axis',(0.,0.,1.));
#20399=DIRECTION('ref_axis',(1.,0.,0.));
#20400=DIRECTION('center_axis',(0.,0.,1.));
#20401=DIRECTION('ref_axis',(1.,0.,0.));
#20402=DIRECTION('center_axis',(0.,0.,1.));
#20403=DIRECTION('ref_axis',(1.,0.,0.));
#20404=DIRECTION('center_axis',(0.,0.,1.));
#20405=DIRECTION('ref_axis',(1.,0.,0.));
#20406=DIRECTION('center_axis',(0.,0.,1.));
#20407=DIRECTION('ref_axis',(1.,0.,0.));
#20408=DIRECTION('center_axis',(0.,0.,1.));
#20409=DIRECTION('ref_axis',(1.,0.,0.));
#20410=DIRECTION('center_axis',(0.,0.,1.));
#20411=DIRECTION('ref_axis',(1.,0.,0.));
#20412=DIRECTION('center_axis',(0.,0.,1.));
#20413=DIRECTION('ref_axis',(1.,0.,0.));
#20414=DIRECTION('center_axis',(0.,0.,1.));
#20415=DIRECTION('ref_axis',(1.,0.,0.));
#20416=DIRECTION('center_axis',(0.,0.,1.));
#20417=DIRECTION('ref_axis',(1.,0.,0.));
#20418=DIRECTION('center_axis',(0.,0.,1.));
#20419=DIRECTION('ref_axis',(1.,0.,0.));
#20420=DIRECTION('center_axis',(0.,0.,1.));
#20421=DIRECTION('ref_axis',(1.,0.,0.));
#20422=DIRECTION('center_axis',(0.,0.,1.));
#20423=DIRECTION('ref_axis',(1.,0.,0.));
#20424=DIRECTION('center_axis',(0.,0.,1.));
#20425=DIRECTION('ref_axis',(1.,0.,0.));
#20426=DIRECTION('center_axis',(0.,0.,1.));
#20427=DIRECTION('ref_axis',(1.,0.,0.));
#20428=DIRECTION('center_axis',(0.,0.,1.));
#20429=DIRECTION('ref_axis',(1.,0.,0.));
#20430=DIRECTION('center_axis',(0.,0.,1.));
#20431=DIRECTION('ref_axis',(1.,0.,0.));
#20432=DIRECTION('center_axis',(0.,0.,1.));
#20433=DIRECTION('ref_axis',(1.,0.,0.));
#20434=DIRECTION('center_axis',(0.,0.,1.));
#20435=DIRECTION('ref_axis',(1.,0.,0.));
#20436=DIRECTION('center_axis',(0.,0.,1.));
#20437=DIRECTION('ref_axis',(1.,0.,0.));
#20438=DIRECTION('center_axis',(0.,0.,1.));
#20439=DIRECTION('ref_axis',(1.,0.,0.));
#20440=DIRECTION('center_axis',(0.,0.,1.));
#20441=DIRECTION('ref_axis',(1.,0.,0.));
#20442=DIRECTION('center_axis',(0.,0.,1.));
#20443=DIRECTION('ref_axis',(1.,0.,0.));
#20444=DIRECTION('center_axis',(0.,0.,1.));
#20445=DIRECTION('ref_axis',(1.,0.,0.));
#20446=DIRECTION('center_axis',(0.,0.,1.));
#20447=DIRECTION('ref_axis',(1.,0.,0.));
#20448=DIRECTION('center_axis',(0.,0.,1.));
#20449=DIRECTION('ref_axis',(1.,0.,0.));
#20450=DIRECTION('center_axis',(0.,0.,1.));
#20451=DIRECTION('ref_axis',(1.,0.,0.));
#20452=DIRECTION('center_axis',(0.,0.,1.));
#20453=DIRECTION('ref_axis',(1.,0.,0.));
#20454=DIRECTION('center_axis',(0.,0.,1.));
#20455=DIRECTION('ref_axis',(1.,0.,0.));
#20456=DIRECTION('center_axis',(0.,0.,1.));
#20457=DIRECTION('ref_axis',(1.,0.,0.));
#20458=DIRECTION('center_axis',(0.,0.,1.));
#20459=DIRECTION('ref_axis',(1.,0.,0.));
#20460=DIRECTION('center_axis',(0.,0.,1.));
#20461=DIRECTION('ref_axis',(1.,0.,0.));
#20462=DIRECTION('center_axis',(0.,0.,1.));
#20463=DIRECTION('ref_axis',(1.,0.,0.));
#20464=DIRECTION('center_axis',(0.,0.,1.));
#20465=DIRECTION('ref_axis',(1.,0.,0.));
#20466=DIRECTION('center_axis',(0.,0.,1.));
#20467=DIRECTION('ref_axis',(1.,0.,0.));
#20468=DIRECTION('center_axis',(0.,0.,1.));
#20469=DIRECTION('ref_axis',(1.,0.,0.));
#20470=DIRECTION('center_axis',(0.,0.,1.));
#20471=DIRECTION('ref_axis',(1.,0.,0.));
#20472=DIRECTION('center_axis',(0.,0.,1.));
#20473=DIRECTION('ref_axis',(1.,0.,0.));
#20474=DIRECTION('center_axis',(0.,0.,1.));
#20475=DIRECTION('ref_axis',(1.,0.,0.));
#20476=DIRECTION('center_axis',(0.,0.,1.));
#20477=DIRECTION('ref_axis',(1.,0.,0.));
#20478=DIRECTION('center_axis',(0.,0.,1.));
#20479=DIRECTION('ref_axis',(1.,0.,0.));
#20480=DIRECTION('center_axis',(0.,0.,1.));
#20481=DIRECTION('ref_axis',(1.,0.,0.));
#20482=DIRECTION('center_axis',(0.,0.,1.));
#20483=DIRECTION('ref_axis',(1.,0.,0.));
#20484=DIRECTION('center_axis',(0.,0.,1.));
#20485=DIRECTION('ref_axis',(1.,0.,0.));
#20486=DIRECTION('center_axis',(0.,0.,1.));
#20487=DIRECTION('ref_axis',(1.,0.,0.));
#20488=DIRECTION('',(0.707106781186547,8.65956056235493E-17,-0.707106781186548));
#20489=DIRECTION('center_axis',(0.,0.,1.));
#20490=DIRECTION('ref_axis',(1.,0.,0.));
#20491=DIRECTION('center_axis',(0.,0.,-1.));
#20492=DIRECTION('ref_axis',(-1.,0.,0.));
#20493=DIRECTION('center_axis',(0.,0.,1.));
#20494=DIRECTION('ref_axis',(1.,0.,0.));
#20495=DIRECTION('center_axis',(0.,0.,1.));
#20496=DIRECTION('ref_axis',(1.,0.,0.));
#20497=DIRECTION('',(0.707106781186547,8.65956056235493E-17,-0.707106781186548));
#20498=DIRECTION('center_axis',(0.,0.,1.));
#20499=DIRECTION('ref_axis',(-0.956376276288062,-0.292137669863679,0.));
#20500=DIRECTION('center_axis',(0.,0.,1.));
#20501=DIRECTION('ref_axis',(1.,0.,0.));
#20502=DIRECTION('center_axis',(0.,0.,-1.));
#20503=DIRECTION('ref_axis',(-1.,0.,0.));
#20504=DIRECTION('center_axis',(0.,0.,-1.));
#20505=DIRECTION('ref_axis',(1.,0.,0.));
#20506=DIRECTION('center_axis',(0.,0.,1.));
#20507=DIRECTION('ref_axis',(1.,0.,0.));
#20508=DIRECTION('',(-0.707106781186548,-8.65956056235493E-17,-0.707106781186547));
#20509=DIRECTION('center_axis',(0.,0.,1.));
#20510=DIRECTION('ref_axis',(1.,0.,0.));
#27584=CARTESIAN_POINT('',(0.,0.,0.));
#27585=CARTESIAN_POINT('Origin',(0.,0.,-0.58));
#27586=CARTESIAN_POINT('',(-0.246625721155034,0.000168494669343964,-1.14757872191302));
#27587=CARTESIAN_POINT('',(-0.246561196381942,0.00027133617513674,-1.15472127808698));
#27588=CARTESIAN_POINT('',(-0.24635,-3.0169173896995E-17,-0.58));
#27589=CARTESIAN_POINT('',(0.107012561312306,0.222107835256874,-1.16365));
#27590=CARTESIAN_POINT('Ctrl Pts',(-0.246625721155034,0.000168494669343964,
-1.14757872191302));
#27591=CARTESIAN_POINT('Ctrl Pts',(-0.246691802496828,0.00929404761416736,
-1.147874469355));
#27592=CARTESIAN_POINT('Ctrl Pts',(-0.246229090033986,0.0184124162622834,
-1.14817021679697));
#27593=CARTESIAN_POINT('Ctrl Pts',(-0.245215256688347,0.0274685625149367,
-1.14846596423895));
#27594=CARTESIAN_POINT('Ctrl Pts',(-0.236164717639783,0.108313215772521,
-1.15110611588088));
#27595=CARTESIAN_POINT('Ctrl Pts',(-0.183194149645427,0.184199230199488,
-1.15374626752281));
#27596=CARTESIAN_POINT('Ctrl Pts',(-0.11042968587659,0.220635087366368,
-1.15638641916474));
#27597=CARTESIAN_POINT('Ctrl Pts',(-0.0436998617096857,0.254049177379322,
-1.15880761277649));
#27598=CARTESIAN_POINT('Ctrl Pts',(0.0396768319088052,0.254285280338311,
-1.16122880638824));
#27599=CARTESIAN_POINT('Ctrl Pts',(0.107142060752371,0.222259968661296,
-1.16365));
#27600=CARTESIAN_POINT('',(-0.106883061872245,0.22195570185245,-1.16365));
#27601=CARTESIAN_POINT('Origin',(0.,0.,-1.16365));
#27602=CARTESIAN_POINT('Ctrl Pts',(-0.106883061872243,0.221955701852451,
-1.16365));
#27603=CARTESIAN_POINT('Ctrl Pts',(-0.180521580324393,0.186494975868788,
-1.16100984835807));
#27604=CARTESIAN_POINT('Ctrl Pts',(-0.234503589708069,0.111829210743298,
-1.15836969671614));
#27605=CARTESIAN_POINT('Ctrl Pts',(-0.244745176790073,0.0312497853638165,
-1.15572954507421));
#27606=CARTESIAN_POINT('Ctrl Pts',(-0.246048921871434,0.0209920949632681,
-1.15539345607847));
#27607=CARTESIAN_POINT('Ctrl Pts',(-0.246643850461073,0.0106385732996934,
-1.15505736708273));
#27608=CARTESIAN_POINT('Ctrl Pts',(-0.246561196381942,0.00027133617513674,
-1.15472127808698));
#27609=CARTESIAN_POINT('Origin',(0.,0.,-0.58));
#27610=CARTESIAN_POINT('',(-0.245986779925945,9.73375077604199E-5,-1.09757872191302));
#27611=CARTESIAN_POINT('',(-0.245972779806236,8.0061809554402E-5,-1.10472127808698));
#27612=CARTESIAN_POINT('',(-0.24635,-3.0169173896995E-17,-0.58));
#27613=CARTESIAN_POINT('Ctrl Pts',(-0.245986779925945,9.73375077604199E-5,
-1.09757872191302));
#27614=CARTESIAN_POINT('Ctrl Pts',(-0.246110835529417,0.0349354674350985,
-1.09870022617009));
#27615=CARTESIAN_POINT('Ctrl Pts',(-0.239203249496549,0.0697265760046414,
-1.09982173042716));
#27616=CARTESIAN_POINT('Ctrl Pts',(-0.225022115887616,0.1012449175221,-1.10094323468424));
#27617=CARTESIAN_POINT('Ctrl Pts',(-0.191638075705932,0.175442764372367,
-1.10358338632616));
#27618=CARTESIAN_POINT('Ctrl Pts',(-0.117945021508019,0.231503380167954,
-1.10622353796809));
#27619=CARTESIAN_POINT('Ctrl Pts',(-0.0375289851653269,0.243878547528516,
-1.10886368961002));
#27620=CARTESIAN_POINT('Ctrl Pts',(0.0428870511773651,0.256253714889078,
-1.11150384125195));
#27621=CARTESIAN_POINT('Ctrl Pts',(0.130026069664836,0.224943433814618,
-1.11414399289388));
#27622=CARTESIAN_POINT('Ctrl Pts',(0.184172931613497,0.164213916417055,
-1.11678414453581));
#27623=CARTESIAN_POINT('Ctrl Pts',(0.238319793562158,0.103484399019491,
-1.11942429617774));
#27624=CARTESIAN_POINT('Ctrl Pts',(0.259474498972009,0.013335645298826,
-1.12206444781966));
#27625=CARTESIAN_POINT('Ctrl Pts',(0.237996781658196,-0.065138960392713,
-1.12470459946159));
#27626=CARTESIAN_POINT('Ctrl Pts',(0.216519064344383,-0.143613566084252,
-1.12734475110352));
#27627=CARTESIAN_POINT('Ctrl Pts',(0.152408924306906,-0.210414023746664,
-1.12998490274545));
#27628=CARTESIAN_POINT('Ctrl Pts',(0.074882920919521,-0.235108951496199,
-1.13262505438738));
#27629=CARTESIAN_POINT('Ctrl Pts',(-0.00264308246786443,-0.259803879245735,
-1.13526520602931));
#27630=CARTESIAN_POINT('Ctrl Pts',(-0.0935849492051585,-0.242393277082393,
-1.13790535767124));
#27631=CARTESIAN_POINT('Ctrl Pts',(-0.15649062752242,-0.190786329956621,
-1.14054550931316));
#27632=CARTESIAN_POINT('Ctrl Pts',(-0.212349667626659,-0.144960347211201,
-1.14288991351311));
#27633=CARTESIAN_POINT('Ctrl Pts',(-0.24610189117968,-0.0721702025233373,
-1.14523431771307));
#27634=CARTESIAN_POINT('Ctrl Pts',(-0.246625721155034,0.000168494669343964,
-1.14757872191302));
#27635=CARTESIAN_POINT('Ctrl Pts',(-0.246561196381942,0.00027133617513674,
-1.15472127808698));
#27636=CARTESIAN_POINT('Ctrl Pts',(-0.245994560226962,-0.0708013978486803,
-1.1524172154408));
#27637=CARTESIAN_POINT('Ctrl Pts',(-0.213582849563037,-0.142518732003264,
-1.15011315279461));
#27638=CARTESIAN_POINT('Ctrl Pts',(-0.159389473178768,-0.188423293933392,
-1.14780909014843));
#27639=CARTESIAN_POINT('Ctrl Pts',(-0.0972910177051287,-0.241023862217646,
-1.1451689385065));
#27640=CARTESIAN_POINT('Ctrl Pts',(-0.00659294197751922,-0.259731913152679,
-1.14252878686457));
#27641=CARTESIAN_POINT('Ctrl Pts',(0.0713071689350544,-0.236198721659865,
-1.13988863522264));
#27642=CARTESIAN_POINT('Ctrl Pts',(0.149207279847628,-0.212665530167051,
-1.13724848358071));
#27643=CARTESIAN_POINT('Ctrl Pts',(0.214309425945166,-0.146891096246389,
-1.13460833193878));
#27644=CARTESIAN_POINT('Ctrl Pts',(0.236974179897325,-0.0687624955230583,
-1.13196818029685));
#27645=CARTESIAN_POINT('Ctrl Pts',(0.259638933849485,0.00936610520027226,
-1.12932802865493));
#27646=CARTESIAN_POINT('Ctrl Pts',(0.239866295656266,0.0998488727262715,
-1.126687877013));
#27647=CARTESIAN_POINT('Ctrl Pts',(0.186651310767665,0.161400207752535,
-1.12404772537107));
#27648=CARTESIAN_POINT('Ctrl Pts',(0.133436325879063,0.222951542778798,
-1.12140757372914));
#27649=CARTESIAN_POINT('Ctrl Pts',(0.0467789942950804,0.255571445305326,
-1.11876742208721));
#27650=CARTESIAN_POINT('Ctrl Pts',(-0.0338170183009678,0.244417831018811,
-1.11612727044528));
#27651=CARTESIAN_POINT('Ctrl Pts',(-0.114413030897016,0.233264216732296,
-1.11348711880335));
#27652=CARTESIAN_POINT('Ctrl Pts',(-0.188947724505129,0.178337085632739,
-1.11084696716143));
#27653=CARTESIAN_POINT('Ctrl Pts',(-0.22345572321461,0.104657009211454,
-1.1082068155195));
#27654=CARTESIAN_POINT('Ctrl Pts',(-0.238641583414576,0.0722327776738232,
-1.10704496970866));
#27655=CARTESIAN_POINT('Ctrl Pts',(-0.246075885996451,0.0361768564216556,
-1.10588312389782));
#27656=CARTESIAN_POINT('Ctrl Pts',(-0.245972779806236,8.0061809554402E-5,
-1.10472127808698));
#27657=CARTESIAN_POINT('Origin',(0.,0.,-0.58));
#27658=CARTESIAN_POINT('',(-0.246278037043403,-0.000220690792281708,-1.04757872191302));
#27659=CARTESIAN_POINT('',(-0.246314807272961,-0.000222469138248099,-1.05472127808698));
#27660=CARTESIAN_POINT('',(-0.24635,-3.0169173896995E-17,-0.58));
#27661=CARTESIAN_POINT('Ctrl Pts',(-0.246278037043403,-0.000220690792281708,
-1.04757872191302));
#27662=CARTESIAN_POINT('Ctrl Pts',(-0.245746501286765,0.0600881005582325,
-1.04952598298519));
#27663=CARTESIAN_POINT('Ctrl Pts',(-0.22339687683019,0.120749402095025,
-1.05147324405735));
#27664=CARTESIAN_POINT('Ctrl Pts',(-0.183195388910587,0.165302445288965,
-1.05342050512952));
#27665=CARTESIAN_POINT('Ctrl Pts',(-0.128689074448717,0.22570872148,-1.05606065677145));
#27666=CARTESIAN_POINT('Ctrl Pts',(-0.0413662088476531,0.256503664111021,
-1.05870080841338));
#27667=CARTESIAN_POINT('Ctrl Pts',(0.0389749219358994,0.243652203884091,
-1.0613409600553));
#27668=CARTESIAN_POINT('Ctrl Pts',(0.119316052719451,0.23080074365716,-1.06398111169723));
#27669=CARTESIAN_POINT('Ctrl Pts',(0.192675448685492,0.174302880572279,
-1.06662126333916));
#27670=CARTESIAN_POINT('Ctrl Pts',(0.225618797988557,0.0999080160201263,
-1.06926141498109));
#27671=CARTESIAN_POINT('Ctrl Pts',(0.258562147291622,0.0255131514679726,
-1.07190156662302));
#27672=CARTESIAN_POINT('Ctrl Pts',(0.25108944993171,-0.0667787145514542,
-1.07454171826495));
#27673=CARTESIAN_POINT('Ctrl Pts',(0.206606490170236,-0.134904463759243,
-1.07718186990688));
#27674=CARTESIAN_POINT('Ctrl Pts',(0.162123530408764,-0.203030212967032,
-1.07982202154881));
#27675=CARTESIAN_POINT('Ctrl Pts',(0.0806303082457299,-0.246989845363183,
-1.08246217319073));
#27676=CARTESIAN_POINT('Ctrl Pts',(-0.000731851916270801,-0.24674859612438,
-1.08510232483266));
#27677=CARTESIAN_POINT('Ctrl Pts',(-0.0820940120782718,-0.246507346885578,
-1.08774247647459));
#27678=CARTESIAN_POINT('Ctrl Pts',(-0.16332511023924,-0.202065216011821,
-1.09038262811652));
#27679=CARTESIAN_POINT('Ctrl Pts',(-0.207403146236997,-0.133676611622469,
-1.09302277975845));
#27680=CARTESIAN_POINT('Ctrl Pts',(-0.232757369469678,-0.0943386533171701,
-1.0945414271433));
#27681=CARTESIAN_POINT('Ctrl Pts',(-0.245818794190178,-0.0470775479853526,
-1.09606007452816));
#27682=CARTESIAN_POINT('Ctrl Pts',(-0.245986779925945,9.73375077604199E-5,
-1.09757872191302));
#27683=CARTESIAN_POINT('Ctrl Pts',(-0.245972779806236,8.0061809554402E-5,
-1.10472127808698));
#27684=CARTESIAN_POINT('Ctrl Pts',(-0.245841589866234,-0.0458486676835616,
-1.10324297225589));
#27685=CARTESIAN_POINT('Ctrl Pts',(-0.233507763949213,-0.0918435688210061,
-1.1017646664248));
#27686=CARTESIAN_POINT('Ctrl Pts',(-0.209412428525571,-0.130507897824181,
-1.10028636059371));
#27687=CARTESIAN_POINT('Ctrl Pts',(-0.166379831316204,-0.199559706695517,
-1.09764620895178));
#27688=CARTESIAN_POINT('Ctrl Pts',(-0.0858333330866237,-0.245230302695177,
-1.09500605730986));
#27689=CARTESIAN_POINT('Ctrl Pts',(-0.00448409557601711,-0.2467084525501,
-1.09236590566793));
#27690=CARTESIAN_POINT('Ctrl Pts',(0.0768651419345896,-0.248186602405022,
-1.089725754026));
#27691=CARTESIAN_POINT('Ctrl Pts',(0.159017118726222,-0.205472306115207,
-1.08708560238407));
#27692=CARTESIAN_POINT('Ctrl Pts',(0.204530894665673,-0.138031142950934,
-1.08444545074214));
#27693=CARTESIAN_POINT('Ctrl Pts',(0.250044670605124,-0.0705899797866627,
-1.08180529910021));
#27694=CARTESIAN_POINT('Ctrl Pts',(0.258920245692393,0.0215780502520655,
-1.07916514745828));
#27695=CARTESIAN_POINT('Ctrl Pts',(0.2271121342129,0.0964654205629691,-1.07652499581635));
#27696=CARTESIAN_POINT('Ctrl Pts',(0.195304022733407,0.171352790873873,
-1.07388484417443));
#27697=CARTESIAN_POINT('Ctrl Pts',(0.122812224687151,0.228959501456952,
-1.0712446925325));
#27698=CARTESIAN_POINT('Ctrl Pts',(0.0426758065862595,0.243031228537435,
-1.06860454089057));
#27699=CARTESIAN_POINT('Ctrl Pts',(-0.0374606115146319,0.257102955617917,
-1.06596438924864));
#27700=CARTESIAN_POINT('Ctrl Pts',(-0.125241649670159,0.227639699195803,
-1.06332423760671));
#27701=CARTESIAN_POINT('Ctrl Pts',(-0.180660295253063,0.168069364017089,
-1.06068408596478));
#27702=CARTESIAN_POINT('Ctrl Pts',(-0.22238147661892,0.123222639022737,
-1.05869648333885));
#27703=CARTESIAN_POINT('Ctrl Pts',(-0.245760855967737,0.0613123401091911,
-1.05670888071292));
#27704=CARTESIAN_POINT('Ctrl Pts',(-0.246314807272961,-0.000222469138248099,
-1.05472127808698));
#27705=CARTESIAN_POINT('Origin',(0.,0.,-0.58));
#27706=CARTESIAN_POINT('',(-0.246722231227711,7.40581688979149E-5,-0.997578721913017));
#27707=CARTESIAN_POINT('',(-0.246704275548887,9.50529893469801E-5,-1.00472127808698));
#27708=CARTESIAN_POINT('',(-0.24635,-3.0169173896995E-17,-0.58));
#27709=CARTESIAN_POINT('Ctrl Pts',(-0.246722231227711,7.40581688979149E-5,
-0.997578721913017));
#27710=CARTESIAN_POINT('Ctrl Pts',(-0.246738504101205,0.0041698706903469,
-0.997711588158351));
#27711=CARTESIAN_POINT('Ctrl Pts',(-0.246645299597814,0.00826492716717819,
-0.997844454403685));
#27712=CARTESIAN_POINT('Ctrl Pts',(-0.246440289964872,0.0123543787050153,
-0.997977320649018));
#27713=CARTESIAN_POINT('Ctrl Pts',(-0.242366595267892,0.0936148385388302,
-1.00061747229095));
#27714=CARTESIAN_POINT('Ctrl Pts',(-0.194147023620069,0.172662207183106,
-1.00325762393288));
#27715=CARTESIAN_POINT('Ctrl Pts',(-0.1237581402402,0.213469833851227,-1.0058977755748));
#27716=CARTESIAN_POINT('Ctrl Pts',(-0.0533692568603309,0.254277460519347,
-1.00853792721673));
#27717=CARTESIAN_POINT('Ctrl Pts',(0.0391889382515836,0.256845345211314,
-1.01117807885866));
#27718=CARTESIAN_POINT('Ctrl Pts',(0.111732096971909,0.220003148994786,
-1.01381823050059));
#27719=CARTESIAN_POINT('Ctrl Pts',(0.184275255692235,0.183160952778257,
-1.01645838214252));
#27720=CARTESIAN_POINT('Ctrl Pts',(0.236803378020971,0.106908675653232,
-1.01909853378445));
#27721=CARTESIAN_POINT('Ctrl Pts',(0.245376232297069,0.0259990745584446,
-1.02173868542638));
#27722=CARTESIAN_POINT('Ctrl Pts',(0.253949086573167,-0.0549105265363425,
-1.02437883706831));
#27723=CARTESIAN_POINT('Ctrl Pts',(0.218566672796627,-0.140477451600892,
-1.02701898871023));
#27724=CARTESIAN_POINT('Ctrl Pts',(0.155354890075996,-0.191703692271305,
-1.02965914035216));
#27725=CARTESIAN_POINT('Ctrl Pts',(0.0921431073553662,-0.242929932941718,
-1.03229929199409));
#27726=CARTESIAN_POINT('Ctrl Pts',(0.00110195569064579,-0.259815489217995,
-1.03493944363602));
#27727=CARTESIAN_POINT('Ctrl Pts',(-0.0762756258156698,-0.234664601507783,
-1.03757959527795));
#27728=CARTESIAN_POINT('Ctrl Pts',(-0.153653207321985,-0.209513713797572,
-1.04021974691988));
#27729=CARTESIAN_POINT('Ctrl Pts',(-0.217367218669897,-0.142326382100871,
-1.0428598985618));
#27730=CARTESIAN_POINT('Ctrl Pts',(-0.238379342682514,-0.0637239113769959,
-1.04550005020373));
#27731=CARTESIAN_POINT('Ctrl Pts',(-0.243893837512198,-0.0430952058664597,
-1.04619294077349));
#27732=CARTESIAN_POINT('Ctrl Pts',(-0.246467172500651,-0.0216802646510429,
-1.04688583134326));
#27733=CARTESIAN_POINT('Ctrl Pts',(-0.246278037043403,-0.000220690792281708,
-1.04757872191302));
#27734=CARTESIAN_POINT('Ctrl Pts',(-0.246314807272961,-0.000222469138248099,
-1.05472127808698));
#27735=CARTESIAN_POINT('Ctrl Pts',(-0.246496674802424,-0.0204249375290262,
-1.05406872907099));
#27736=CARTESIAN_POINT('Ctrl Pts',(-0.244218253557143,-0.0405869329434031,
-1.05341618005499));
#27737=CARTESIAN_POINT('Ctrl Pts',(-0.23932087891077,-0.0600913293117114,
-1.052763631039));
#27738=CARTESIAN_POINT('Ctrl Pts',(-0.21950656397529,-0.139004273526488,
-1.05012347939707));
#27739=CARTESIAN_POINT('Ctrl Pts',(-0.156821681094049,-0.20715274802073,
-1.04748332775514));
#27740=CARTESIAN_POINT('Ctrl Pts',(-0.0798355365549801,-0.233477462201628,
-1.04484317611321));
#27741=CARTESIAN_POINT('Ctrl Pts',(-0.00284939201591072,-0.259802176382527,
-1.04220302447128));
#27742=CARTESIAN_POINT('Ctrl Pts',(0.0884380141809866,-0.244303130250082,
-1.03956287282935));
#27743=CARTESIAN_POINT('Ctrl Pts',(0.152421523049327,-0.194044132905792,
-1.03692272118743));
#27744=CARTESIAN_POINT('Ctrl Pts',(0.216405031917667,-0.143785135561503,
-1.0342825695455));
#27745=CARTESIAN_POINT('Ctrl Pts',(0.253084643457451,-0.0587661870053685,
-1.03164241790357));
#27746=CARTESIAN_POINT('Ctrl Pts',(0.245743240432631,0.0222644322950805,
-1.02900226626164));
#27747=CARTESIAN_POINT('Ctrl Pts',(0.238401837407811,0.103295051595529,
-1.02636211461971));
#27748=CARTESIAN_POINT('Ctrl Pts',(0.187039419818387,0.180337341640293,
-1.02372196297778));
#27749=CARTESIAN_POINT('Ctrl Pts',(0.115064941057801,0.218278498474838,
-1.02108181133585));
#27750=CARTESIAN_POINT('Ctrl Pts',(0.0430904622972144,0.256219655309383,
-1.01844165969393));
#27751=CARTESIAN_POINT('Ctrl Pts',(-0.0494960776345338,0.255059678933708,
-1.015801508052));
#27752=CARTESIAN_POINT('Ctrl Pts',(-0.12049741408824,0.215327234607512,
-1.01316135641007));
#27753=CARTESIAN_POINT('Ctrl Pts',(-0.191498750541946,0.175594790281315,
-1.01052120476814));
#27754=CARTESIAN_POINT('Ctrl Pts',(-0.240914883517609,0.0972898780045968,
-1.00788105312621));
#27755=CARTESIAN_POINT('Ctrl Pts',(-0.246223901669846,0.0161007690757402,
-1.00524090148428));
#27756=CARTESIAN_POINT('Ctrl Pts',(-0.246572201114063,0.0107743375764552,
-1.00506769368518));
#27757=CARTESIAN_POINT('Ctrl Pts',(-0.246730661403056,0.00543549235529937,
-1.00489448588608));
#27758=CARTESIAN_POINT('Ctrl Pts',(-0.246704275548887,9.50529893469801E-5,
-1.00472127808698));
#27759=CARTESIAN_POINT('Origin',(0.,0.,-0.58));
#27760=CARTESIAN_POINT('',(-0.246068967124758,0.000163257868156283,-0.947578721913017));
#27761=CARTESIAN_POINT('',(-0.246044690514741,0.000148590017213961,-0.954721278086983));
#27762=CARTESIAN_POINT('',(-0.24635,-3.0169173896995E-17,-0.58));
#27763=CARTESIAN_POINT('Ctrl Pts',(-0.246068967124758,0.000163257868156283,
-0.947578721913017));
#27764=CARTESIAN_POINT('Ctrl Pts',(-0.246251016085628,0.0299166900142917,
-0.948537344973446));
#27765=CARTESIAN_POINT('Ctrl Pts',(-0.241256522550863,0.059611081389455,
-0.949495968033874));
#27766=CARTESIAN_POINT('Ctrl Pts',(-0.230811068104658,0.0872450458601642,
-0.950454591094303));
#27767=CARTESIAN_POINT('Ctrl Pts',(-0.202043156247306,0.163351974309931,
-0.953094742736232));
#27768=CARTESIAN_POINT('Ctrl Pts',(-0.131929095164112,0.22383033384413,
-0.955734894378161));
#27769=CARTESIAN_POINT('Ctrl Pts',(-0.0524240884788059,0.24111649079944,
-0.958375046020089));
#27770=CARTESIAN_POINT('Ctrl Pts',(0.0270809182064996,0.25840264775475,
-0.961015197662018));
#27771=CARTESIAN_POINT('Ctrl Pts',(0.115976870493916,0.232496602131172,
-0.963655349303947));
#27772=CARTESIAN_POINT('Ctrl Pts',(0.173748524901487,0.175205300374098,
-0.966295500945875));
#27773=CARTESIAN_POINT('Ctrl Pts',(0.231520179309058,0.117913998617024,
-0.968935652587804));
#27774=CARTESIAN_POINT('Ctrl Pts',(0.258167535836783,0.0292374407264532,
-0.971575804229732));
#27775=CARTESIAN_POINT('Ctrl Pts',(0.241545787992139,-0.0504091210988275,
-0.974215955871661));
#27776=CARTESIAN_POINT('Ctrl Pts',(0.224924040147495,-0.130055682924108,
-0.976856107513589));
#27777=CARTESIAN_POINT('Ctrl Pts',(0.165033187930483,-0.200672248684099,
-0.979496259155518));
#27778=CARTESIAN_POINT('Ctrl Pts',(0.0891691025107115,-0.23007459301933,
-0.982136410797447));
#27779=CARTESIAN_POINT('Ctrl Pts',(0.0133050170909386,-0.259476937354563,
-0.984776562439376));
#27780=CARTESIAN_POINT('Ctrl Pts',(-0.0785323015315946,-0.247665060265035,
-0.987416714081304));
#27781=CARTESIAN_POINT('Ctrl Pts',(-0.144487051969792,-0.200022346208593,
-0.990056865723233));
#27782=CARTESIAN_POINT('Ctrl Pts',(-0.20712261425475,-0.15477726281611,
-0.992564151119827));
#27783=CARTESIAN_POINT('Ctrl Pts',(-0.24641514993727,-0.0772169866440894,
-0.995071436516422));
#27784=CARTESIAN_POINT('Ctrl Pts',(-0.246722231227711,7.40581688979149E-5,
-0.997578721913017));
#27785=CARTESIAN_POINT('Ctrl Pts',(-0.246704275548887,9.50529893469801E-5,
-1.00472127808698));
#27786=CARTESIAN_POINT('Ctrl Pts',(-0.246328470182043,-0.0759671340501024,
-1.00225433424415));
#27787=CARTESIAN_POINT('Ctrl Pts',(-0.208455879730509,-0.152352699786071,
-0.999787390401325));
#27788=CARTESIAN_POINT('Ctrl Pts',(-0.147512243360909,-0.197801876593369,
-0.997320446558496));
#27789=CARTESIAN_POINT('Ctrl Pts',(-0.0822896635709238,-0.246442107752627,
-0.994680294916568));
#27790=CARTESIAN_POINT('Ctrl Pts',(0.00935739933785658,-0.259649264490148,
-0.99204014327464));
#27791=CARTESIAN_POINT('Ctrl Pts',(0.0856598552539378,-0.231404048586573,
-0.989399991632711));
#27792=CARTESIAN_POINT('Ctrl Pts',(0.161962311170019,-0.203158832682998,
-0.986759839990783));
#27793=CARTESIAN_POINT('Ctrl Pts',(0.222920160093402,-0.133461244138326,
-0.984119688348854));
#27794=CARTESIAN_POINT('Ctrl Pts',(0.240751235997126,-0.0540766753887532,
-0.981479536706925));
#27795=CARTESIAN_POINT('Ctrl Pts',(0.25858231190085,0.02530789336082,-0.978839385064996));
#27796=CARTESIAN_POINT('Ctrl Pts',(0.233286614784916,0.114379442315294,
-0.976199233423067));
#27797=CARTESIAN_POINT('Ctrl Pts',(0.176392918556739,0.172542698242494,
-0.973559081781138));
#27798=CARTESIAN_POINT('Ctrl Pts',(0.119499222328562,0.230705954169694,
-0.97091893013921));
#27799=CARTESIAN_POINT('Ctrl Pts',(0.0310075269881437,0.257960917069619,
-0.968278778497282));
#27800=CARTESIAN_POINT('Ctrl Pts',(-0.0487511682798576,0.241885857484542,
-0.965638626855353));
#27801=CARTESIAN_POINT('Ctrl Pts',(-0.128509863547858,0.225810797899465,
-0.962998475213425));
#27802=CARTESIAN_POINT('Ctrl Pts',(-0.199535558743442,0.166405715829386,
-0.960358323571496));
#27803=CARTESIAN_POINT('Ctrl Pts',(-0.229457563609463,0.0907450877634371,
-0.957718171929567));
#27804=CARTESIAN_POINT('Ctrl Pts',(-0.24077927088272,0.0621170768093258,
-0.956719207315372));
#27805=CARTESIAN_POINT('Ctrl Pts',(-0.246216292346804,0.0311618105631647,
-0.955720242701178));
#27806=CARTESIAN_POINT('Ctrl Pts',(-0.246044690514741,0.000148590017213961,
-0.954721278086983));
#27807=CARTESIAN_POINT('Origin',(0.,0.,-0.58));
#27808=CARTESIAN_POINT('',(-0.246140990925822,-0.000194203052083286,-0.897578721913017));
#27809=CARTESIAN_POINT('',(-0.24617270257491,-0.000203503496127644,-0.904721278086982));
#27810=CARTESIAN_POINT('',(-0.24635,-3.0169173896995E-17,-0.58));
#27811=CARTESIAN_POINT('Ctrl Pts',(-0.246140990925822,-0.000194203052083286,
-0.897578721913017));
#27812=CARTESIAN_POINT('Ctrl Pts',(-0.245730015818884,0.0551480007569202,
-0.899363101788541));
#27813=CARTESIAN_POINT('Ctrl Pts',(-0.227258101070754,0.110738834210626,
-0.901147481664065));
#27814=CARTESIAN_POINT('Ctrl Pts',(-0.192994105070856,0.15374889461325,
-0.902931861539588));
#27815=CARTESIAN_POINT('Ctrl Pts',(-0.142297419606602,0.217386174515947,
-0.905572013181517));
#27816=CARTESIAN_POINT('Ctrl Pts',(-0.0570288952207411,0.253481773718221,
-0.908212164823445));
#27817=CARTESIAN_POINT('Ctrl Pts',(0.0239494621323068,0.245584752072496,
-0.910852316465374));
#27818=CARTESIAN_POINT('Ctrl Pts',(0.104927819485355,0.237687730426771,
-0.913492468107302));
#27819=CARTESIAN_POINT('Ctrl Pts',(0.181616009805589,0.185798087933047,
-0.916132619749232));
#27820=CARTESIAN_POINT('Ctrl Pts',(0.219062602535076,0.113565062221743,
-0.91877277139116));
#27821=CARTESIAN_POINT('Ctrl Pts',(0.256509195264563,0.0413320365104399,
-0.921412923033089));
#27822=CARTESIAN_POINT('Ctrl Pts',(0.254714190403302,-0.0512443724184431,
-0.924053074675017));
#27823=CARTESIAN_POINT('Ctrl Pts',(0.214495679856809,-0.121971515156742,
-0.926693226316946));
#27824=CARTESIAN_POINT('Ctrl Pts',(0.174277169310317,-0.192698657895042,
-0.929333377958874));
#27825=CARTESIAN_POINT('Ctrl Pts',(0.0956351530785919,-0.241576534442757,
-0.931973529600803));
#27826=CARTESIAN_POINT('Ctrl Pts',(0.0144115379507457,-0.246328550438247,
-0.934613681242732));
#27827=CARTESIAN_POINT('Ctrl Pts',(-0.0668120771770993,-0.251080566433737,
-0.937253832884661));
#27828=CARTESIAN_POINT('Ctrl Pts',(-0.150617291201066,-0.211706721877003,
-0.939893984526589));
#27829=CARTESIAN_POINT('Ctrl Pts',(-0.198809016897293,-0.146152050915969,
-0.942534136168517));
#27830=CARTESIAN_POINT('Ctrl Pts',(-0.229502619061303,-0.104399883683908,
-0.944215664750017));
#27831=CARTESIAN_POINT('Ctrl Pts',(-0.245749633547702,-0.0520274817631998,
-0.945897193331517));
#27832=CARTESIAN_POINT('Ctrl Pts',(-0.246068967124758,0.000163257868156283,
-0.947578721913017));
#27833=CARTESIAN_POINT('Ctrl Pts',(-0.246044690514741,0.000148590017213961,
-0.954721278086983));
#27834=CARTESIAN_POINT('Ctrl Pts',(-0.245762767915366,-0.0508026594314752,
-0.953080091059249));
#27835=CARTESIAN_POINT('Ctrl Pts',(-0.230342715915977,-0.101910332238121,
-0.951438904031516));
#27836=CARTESIAN_POINT('Ctrl Pts',(-0.201008675250746,-0.143111693871055,
-0.949797717003782));
#27837=CARTESIAN_POINT('Ctrl Pts',(-0.153819467489548,-0.209391673377774,
-0.947157565361853));
#27838=CARTESIAN_POINT('Ctrl Pts',(-0.0706227374306924,-0.250035458329393,
-0.944517413719924));
#27839=CARTESIAN_POINT('Ctrl Pts',(0.0106637505259729,-0.246519226181408,
-0.941877262077995));
#27840=CARTESIAN_POINT('Ctrl Pts',(0.0919502384826396,-0.243002994033424,
-0.939237110436067));
#27841=CARTESIAN_POINT('Ctrl Pts',(0.171326484337116,-0.195326744785834,
-0.936596958794139));
#27842=CARTESIAN_POINT('Ctrl Pts',(0.212615948603837,-0.125219418822052,
-0.93395680715221));
#27843=CARTESIAN_POINT('Ctrl Pts',(0.253905412870557,-0.0551120928582709,
-0.931316655510282));
#27844=CARTESIAN_POINT('Ctrl Pts',(0.257108095549521,0.0374263098217014,
-0.928676503868353));
#27845=CARTESIAN_POINT('Ctrl Pts',(0.220764341110336,0.110220461552371,
-0.926036352226424));
#27846=CARTESIAN_POINT('Ctrl Pts',(0.18442058667115,0.183014613283042,-0.923396200584495));
#27847=CARTESIAN_POINT('Ctrl Pts',(0.108530395113813,0.236064514064409,
-0.920756048942567));
#27848=CARTESIAN_POINT('Ctrl Pts',(0.0276815008613437,0.245192126629843,
-0.918115897300638));
#27849=CARTESIAN_POINT('Ctrl Pts',(-0.0531673933911258,0.254319739195276,
-0.915475745658709));
#27850=CARTESIAN_POINT('Ctrl Pts',(-0.138974990338729,0.219525063544776,
-0.912835594016781));
#27851=CARTESIAN_POINT('Ctrl Pts',(-0.19063359616867,0.156666130553969,
-0.910195442374852));
#27852=CARTESIAN_POINT('Ctrl Pts',(-0.22633706242725,0.113221640385657,
-0.908370720945562));
#27853=CARTESIAN_POINT('Ctrl Pts',(-0.245728300868163,0.0563714669369404,
-0.906545999516272));
#27854=CARTESIAN_POINT('Ctrl Pts',(-0.24617270257491,-0.000203503496127644,
-0.904721278086982));
#27855=CARTESIAN_POINT('Origin',(0.,0.,-0.58));
#27856=CARTESIAN_POINT('',(-0.24674826027019,-1.7099131415399E-5,-0.847578721913017));
#27857=CARTESIAN_POINT('',(-0.246749580224057,5.88930587390795E-6,-0.854721278086983));
#27858=CARTESIAN_POINT('',(-0.24635,-3.0169173896995E-17,-0.58));
#27859=CARTESIAN_POINT('Ctrl Pts',(-0.24674826027019,-1.7099131415399E-5,
-0.847578721913017));
#27860=CARTESIAN_POINT('Ctrl Pts',(-0.246667412551575,0.0804217509967416,
-0.850188858603636));
#27861=CARTESIAN_POINT('Ctrl Pts',(-0.203606490563192,0.160934891961365,
-0.852798995294255));
#27862=CARTESIAN_POINT('Ctrl Pts',(-0.136624724734367,0.205472946584612,
-0.855409131984873));
#27863=CARTESIAN_POINT('Ctrl Pts',(-0.0688727101874428,0.25052316118238,
-0.858049283626802));
#27864=CARTESIAN_POINT('Ctrl Pts',(0.0233534610933846,0.258766149935299,
-0.86068943526873));
#27865=CARTESIAN_POINT('Ctrl Pts',(0.0980207641052817,0.226445086038806,
-0.863329586910659));
#27866=CARTESIAN_POINT('Ctrl Pts',(0.172688067117179,0.194124022142313,
-0.865969738552587));
#27867=CARTESIAN_POINT('Ctrl Pts',(0.229796501860146,0.121238905596409,
-0.868609890194516));
#27868=CARTESIAN_POINT('Ctrl Pts',(0.243318312523803,0.0410078770173896,
-0.871250041836445));
#27869=CARTESIAN_POINT('Ctrl Pts',(0.25684012318746,-0.0392231515616299,
-0.873890193478373));
#27870=CARTESIAN_POINT('Ctrl Pts',(0.226775309771808,-0.126800092173765,
-0.876530345120302));
#27871=CARTESIAN_POINT('Ctrl Pts',(0.166826219847552,-0.181808854455111,
-0.87917049676223));
#27872=CARTESIAN_POINT('Ctrl Pts',(0.106877129923296,-0.236817616736456,
-0.881810648404159));
#27873=CARTESIAN_POINT('Ctrl Pts',(0.0170437634904362,-0.259258200687012,
-0.884450800046088));
#27874=CARTESIAN_POINT('Ctrl Pts',(-0.061731399838991,-0.238903079638643,
-0.887090951688017));
#27875=CARTESIAN_POINT('Ctrl Pts',(-0.140506563168418,-0.218547958590274,
-0.889731103329945));
#27876=CARTESIAN_POINT('Ctrl Pts',(-0.208223523394413,-0.15539713254298,
-0.892371254971873));
#27877=CARTESIAN_POINT('Ctrl Pts',(-0.234019580236086,-0.0782322392177732,
-0.895011406613802));
#27878=CARTESIAN_POINT('Ctrl Pts',(-0.242381045834917,-0.0532202149019548,
-0.895867178380207));
#27879=CARTESIAN_POINT('Ctrl Pts',(-0.24633809071272,-0.0267358022709602,
-0.896722950146612));
#27880=CARTESIAN_POINT('Ctrl Pts',(-0.246140990925822,-0.000194203052083286,
-0.897578721913017));
#27881=CARTESIAN_POINT('Ctrl Pts',(-0.24617270257491,-0.000203503496127644,
-0.904721278086982));
#27882=CARTESIAN_POINT('Ctrl Pts',(-0.24637129649309,-0.0254856859869767,
-0.903905847874344));
#27883=CARTESIAN_POINT('Ctrl Pts',(-0.242786186315468,-0.0507129101334804,
-0.903090417661705));
#27884=CARTESIAN_POINT('Ctrl Pts',(-0.235182253523972,-0.0746642623906653,
-0.902274987449066));
#27885=CARTESIAN_POINT('Ctrl Pts',(-0.210562690337051,-0.152212532013379,
-0.899634835807138));
#27886=CARTESIAN_POINT('Ctrl Pts',(-0.143813949250927,-0.216385880927691,
-0.896994684165209));
#27887=CARTESIAN_POINT('Ctrl Pts',(-0.0653574547268311,-0.237936646111214,
-0.894354532523281));
#27888=CARTESIAN_POINT('Ctrl Pts',(0.0130990397972646,-0.259487411294737,
-0.891714380881352));
#27889=CARTESIAN_POINT('Ctrl Pts',(0.103263287759333,-0.238415592747473,
-0.889074229239423));
#27890=CARTESIAN_POINT('Ctrl Pts',(0.164042006891183,-0.184324888243821,
-0.886434077597494));
#27891=CARTESIAN_POINT('Ctrl Pts',(0.224820726023033,-0.130234183740168,
-0.883793925955566));
#27892=CARTESIAN_POINT('Ctrl Pts',(0.256213916324662,-0.0431245932801274,
-0.881153774313637));
#27893=CARTESIAN_POINT('Ctrl Pts',(0.243913808813169,0.0373027924054035,
-0.878513622671709));
#27894=CARTESIAN_POINT('Ctrl Pts',(0.231613701301676,0.117730178090933,
-0.87587347102978));
#27895=CARTESIAN_POINT('Ctrl Pts',(0.175620295977063,0.191475359001952,
-0.873233319387852));
#27896=CARTESIAN_POINT('Ctrl Pts',(0.101453162537552,0.224928211352256,
-0.870593167745923));
#27897=CARTESIAN_POINT('Ctrl Pts',(0.0272860290980399,0.258381063702561,
-0.867953016103994));
#27898=CARTESIAN_POINT('Ctrl Pts',(-0.0650548324563724,0.251541587492149,
-0.865312864462065));
#27899=CARTESIAN_POINT('Ctrl Pts',(-0.133484125852437,0.207526944266042,
-0.862672712820137));
#27900=CARTESIAN_POINT('Ctrl Pts',(-0.202181071340161,0.16334014360942,
-0.860022234575752));
#27901=CARTESIAN_POINT('Ctrl Pts',(-0.246778412616135,0.0816867933466605,
-0.857371756331367));
#27902=CARTESIAN_POINT('Ctrl Pts',(-0.246749580224057,5.88930587390795E-6,
-0.854721278086983));
#27903=CARTESIAN_POINT('Origin',(0.,0.,-0.58));
#27904=CARTESIAN_POINT('',(-0.246188793287857,0.000207412629416426,-0.797578721913017));
#27905=CARTESIAN_POINT('',(-0.246156246887236,0.000198954902853581,-0.804721278086982));
#27906=CARTESIAN_POINT('',(-0.24635,-3.0169173896995E-17,-0.58));
#27907=CARTESIAN_POINT('Ctrl Pts',(-0.246188793287857,0.000207412629416426,
-0.797578721913017));
#27908=CARTESIAN_POINT('Ctrl Pts',(-0.246387252386039,0.0248750860659389,
-0.798374463776802));
#27909=CARTESIAN_POINT('Ctrl Pts',(-0.242976611149663,0.049489136932403,
-0.799170205640587));
#27910=CARTESIAN_POINT('Ctrl Pts',(-0.235729958539167,0.0729166224809383,
-0.799965947504372));
#27911=CARTESIAN_POINT('Ctrl Pts',(-0.211686656736383,0.150645490663177,
-0.802606099146301));
#27912=CARTESIAN_POINT('Ctrl Pts',(-0.145416064350721,0.21531250016226,
-0.805246250788229));
#27913=CARTESIAN_POINT('Ctrl Pts',(-0.0671216846612779,0.237444997073294,
-0.807886402430158));
#27914=CARTESIAN_POINT('Ctrl Pts',(0.0111726950281651,0.259577493984328,
-0.810526554072086));
#27915=CARTESIAN_POINT('Ctrl Pts',(0.101490862021389,0.239175478307313,
-0.813166705714014));
#27916=CARTESIAN_POINT('Ctrl Pts',(0.16266938387061,0.185537378277427,-0.815806857355943));
#27917=CARTESIAN_POINT('Ctrl Pts',(0.223847905719831,0.131899278247541,
-0.818447008997872));
#27918=CARTESIAN_POINT('Ctrl Pts',(0.255886782425048,0.0450250938647844,
-0.821087160639801));
#27919=CARTESIAN_POINT('Ctrl Pts',(0.244183966791736,-0.0354913728778911,
-0.82372731228173));
#27920=CARTESIAN_POINT('Ctrl Pts',(0.232481151158423,-0.116007839620565,
-0.826367463923659));
#27921=CARTESIAN_POINT('Ctrl Pts',(0.177036643186582,-0.190166588723159,
-0.829007615565587));
#27922=CARTESIAN_POINT('Ctrl Pts',(0.103119846967095,-0.224169008447617,
-0.831647767207515));
#27923=CARTESIAN_POINT('Ctrl Pts',(0.0292030507476063,-0.258171428172075,
-0.834287918849444));
#27924=CARTESIAN_POINT('Ctrl Pts',(-0.0631860337195292,-0.252017518518398,
-0.836928070491373));
#27925=CARTESIAN_POINT('Ctrl Pts',(-0.131940132073209,-0.208511987030504,
-0.839568222133302));
#27926=CARTESIAN_POINT('Ctrl Pts',(-0.200694230426889,-0.16500645554261,
-0.84220837377523));
#27927=CARTESIAN_POINT('Ctrl Pts',(-0.245813342667112,-0.0841493022204997,
-0.844848525417158));
#27928=CARTESIAN_POINT('Ctrl Pts',(-0.246733969880713,-0.00279200533813568,
-0.847488677059087));
#27929=CARTESIAN_POINT('Ctrl Pts',(-0.246744436166267,-0.00186708297160882,
-0.847518692010397));
#27930=CARTESIAN_POINT('Ctrl Pts',(-0.246749189968755,-0.000942095963463235,
-0.847548706961707));
#27931=CARTESIAN_POINT('Ctrl Pts',(-0.24674826027019,-1.7099131415399E-5,
-0.847578721913017));
#27932=CARTESIAN_POINT('Ctrl Pts',(-0.246749580224057,5.88930587390795E-6,
-0.854721278086983));
#27933=CARTESIAN_POINT('Ctrl Pts',(-0.246720972501359,-0.0810385362230983,
-0.85209145304751));
#27934=CARTESIAN_POINT('Ctrl Pts',(-0.202914101569483,-0.162109483810441,
-0.849461628008038));
#27935=CARTESIAN_POINT('Ctrl Pts',(-0.13509588376053,-0.206481346958881,
-0.846831802968566));
#27936=CARTESIAN_POINT('Ctrl Pts',(-0.0670113623898996,-0.251027446257671,
-0.844191651326637));
#27937=CARTESIAN_POINT('Ctrl Pts',(0.0252734480549719,-0.258585680747039,
-0.841551499684708));
#27938=CARTESIAN_POINT('Ctrl Pts',(0.0996987971698373,-0.225711307412542,
-0.838911348042779));
#27939=CARTESIAN_POINT('Ctrl Pts',(0.174124146284703,-0.192836934078045,
-0.83627119640085));
#27940=CARTESIAN_POINT('Ctrl Pts',(0.230690034069562,-0.119529952919682,
-0.833631044758922));
#27941=CARTESIAN_POINT('Ctrl Pts',(0.24361597606379,-0.0392007736846921,
-0.830990893116994));
#27942=CARTESIAN_POINT('Ctrl Pts',(0.256541918058019,0.0411284055502995,
-0.828350741475065));
#27943=CARTESIAN_POINT('Ctrl Pts',(0.225827914261615,0.128479782861919,
-0.825710589833136));
#27944=CARTESIAN_POINT('Ctrl Pts',(0.165472187430463,0.183042070677671,
-0.823070438191208));
#27945=CARTESIAN_POINT('Ctrl Pts',(0.105116460599312,0.237604358493422,
-0.820430286549279));
#27946=CARTESIAN_POINT('Ctrl Pts',(0.0151190107334124,0.259377556813307,
-0.81779013490735));
#27947=CARTESIAN_POINT('Ctrl Pts',(-0.063502899844963,0.238438306826467,
-0.815149983265422));
#27948=CARTESIAN_POINT('Ctrl Pts',(-0.142124810423339,0.217499056839627,
-0.812509831623493));
#27949=CARTESIAN_POINT('Ctrl Pts',(-0.209371181714192,0.153847358546061,
-0.809869679981565));
#27950=CARTESIAN_POINT('Ctrl Pts',(-0.234593789178183,0.0764931273384339,
-0.807229528339636));
#27951=CARTESIAN_POINT('Ctrl Pts',(-0.242581286378397,0.0519965836691203,
-0.806393444922085));
#27952=CARTESIAN_POINT('Ctrl Pts',(-0.246354377081631,0.0261258640936213,
-0.805557361504533));
#27953=CARTESIAN_POINT('Ctrl Pts',(-0.246156246887236,0.000198954902853581,
-0.804721278086982));
#27954=CARTESIAN_POINT('Origin',(0.,0.,-0.58));
#27955=CARTESIAN_POINT('',(-0.246033746957446,-0.000140975359651019,-0.747578721913017));
#27956=CARTESIAN_POINT('',(-0.246056814395214,-0.000156261806827737,-0.754721278086983));
#27957=CARTESIAN_POINT('',(-0.24635,-3.0169173896995E-17,-0.58));
#27958=CARTESIAN_POINT('Ctrl Pts',(-0.246033746957446,-0.000140975359651019,
-0.747578721913017));
#27959=CARTESIAN_POINT('Ctrl Pts',(-0.245770202673151,0.0502046633637533,
-0.749200220591897));
#27960=CARTESIAN_POINT('Ctrl Pts',(-0.23074455683355,0.100694729418671,
-0.750821719270777));
#27961=CARTESIAN_POINT('Ctrl Pts',(-0.202065355776875,0.141615815436235,
-0.752443217949657));
#27962=CARTESIAN_POINT('Ctrl Pts',(-0.155369394352292,0.208244221518818,
-0.755083369591585));
#27963=CARTESIAN_POINT('Ctrl Pts',(-0.0724766230355756,0.249504395974772,
-0.757723521233513));
#27964=CARTESIAN_POINT('Ctrl Pts',(0.00883372608632075,0.246591590429067,
-0.760363672875442));
#27965=CARTESIAN_POINT('Ctrl Pts',(0.0901440752082165,0.243678784883362,
-0.763003824517371));
#27966=CARTESIAN_POINT('Ctrl Pts',(0.169872002135292,0.196592999335999,
-0.765643976159301));
#27967=CARTESIAN_POINT('Ctrl Pts',(0.211680685123689,0.126794064263554,
-0.768284127801229));
#27968=CARTESIAN_POINT('Ctrl Pts',(0.253489368112086,0.056995129191111,
-0.770924279443158));
#27969=CARTESIAN_POINT('Ctrl Pts',(0.257378807161808,-0.0355169554064133,
-0.773564431085085));
#27970=CARTESIAN_POINT('Ctrl Pts',(0.221576350469646,-0.108578856594908,
-0.776204582727014));
#27971=CARTESIAN_POINT('Ctrl Pts',(0.185773893777484,-0.181640757783402,
-0.778844734368942));
#27972=CARTESIAN_POINT('Ctrl Pts',(0.110279541343437,-0.235252475562867,
-0.781484886010872));
#27973=CARTESIAN_POINT('Ctrl Pts',(0.0295006198445558,-0.244979918800893,
-0.7841250376528));
#27974=CARTESIAN_POINT('Ctrl Pts',(-0.0512783016543263,-0.254707362038918,
-0.786765189294729));
#27975=CARTESIAN_POINT('Ctrl Pts',(-0.137341792218043,-0.220550530735504,
-0.789405340936657));
#27976=CARTESIAN_POINT('Ctrl Pts',(-0.189465531889949,-0.1580767516511,
-0.792045492578586));
#27977=CARTESIAN_POINT('Ctrl Pts',(-0.225879173287477,-0.114432573342958,
-0.79388990235673));
#27978=CARTESIAN_POINT('Ctrl Pts',(-0.245728794992044,-0.0569685387198996,
-0.795734312134873));
#27979=CARTESIAN_POINT('Ctrl Pts',(-0.246188793287857,0.000207412629416426,
-0.797578721913017));
#27980=CARTESIAN_POINT('Ctrl Pts',(-0.246156246887236,0.000198954902853581,
-0.804721278086982));
#27981=CARTESIAN_POINT('Ctrl Pts',(-0.24572872927297,-0.055745119630262,
-0.802917209862605));
#27982=CARTESIAN_POINT('Ctrl Pts',(-0.226811474403897,-0.111950809230771,
-0.801113141638227));
#27983=CARTESIAN_POINT('Ctrl Pts',(-0.191847619700623,-0.15517710934992,
-0.79930907341385));
#27984=CARTESIAN_POINT('Ctrl Pts',(-0.140679999121939,-0.218436350708962,
-0.796668921771921));
#27985=CARTESIAN_POINT('Ctrl Pts',(-0.0551459143274415,-0.253898069305357,
-0.794028770129993));
#27986=CARTESIAN_POINT('Ctrl Pts',(0.0257715968441432,-0.245400222589742,
-0.791388618488064));
#27987=CARTESIAN_POINT('Ctrl Pts',(0.106689108015727,-0.236902375874126,
-0.788748466846136));
#27988=CARTESIAN_POINT('Ctrl Pts',(0.182990045564397,-0.184444963846501,
-0.786108315204207));
#27989=CARTESIAN_POINT('Ctrl Pts',(0.219899473361048,-0.111935990934666,
-0.783468163562278));
#27990=CARTESIAN_POINT('Ctrl Pts',(0.256808901157699,-0.0394270180228303,
-0.780828011920349));
#27991=CARTESIAN_POINT('Ctrl Pts',(0.25432681920233,0.0531335157732174,
-0.778187860278422));
#27992=CARTESIAN_POINT('Ctrl Pts',(0.213584461844586,0.123560196299417,
-0.775547708636493));
#27993=CARTESIAN_POINT('Ctrl Pts',(0.172842104486842,0.193986876825616,
-0.772907556994564));
#27994=CARTESIAN_POINT('Ctrl Pts',(0.0938394717267237,0.242279704081969,
-0.770267405352635));
#27995=CARTESIAN_POINT('Ctrl Pts',(0.0125828250405317,0.24642872593306,
-0.767627253710706));
#27996=CARTESIAN_POINT('Ctrl Pts',(-0.0686738216456602,0.25057774778415,
-0.764987102068778));
#27997=CARTESIAN_POINT('Ctrl Pts',(-0.152184482257925,0.210582964229978,
-0.762346950426849));
#27998=CARTESIAN_POINT('Ctrl Pts',(-0.199888315315273,0.144672408742696,
-0.759706798784921));
#27999=CARTESIAN_POINT('Ctrl Pts',(-0.229915434881869,0.103185089936717,
-0.758044958552275));
#28000=CARTESIAN_POINT('Ctrl Pts',(-0.245755682841279,0.0514297928114553,
-0.756383118319629));
#28001=CARTESIAN_POINT('Ctrl Pts',(-0.246056814395214,-0.000156261806827737,
-0.754721278086983));
#28002=CARTESIAN_POINT('Origin',(0.,0.,-0.58));
#28003=CARTESIAN_POINT('',(-0.246694142079541,-0.000104913238225313,-0.697578721913017));
#28004=CARTESIAN_POINT('',(-0.24671395673833,-8.44291920866902E-5,-0.704721278086983));
#28005=CARTESIAN_POINT('',(-0.24635,-3.0169173896995E-17,-0.58));
#28006=CARTESIAN_POINT('Ctrl Pts',(-0.246694142079541,-0.000104913238225313,
-0.697578721913017));
#28007=CARTESIAN_POINT('Ctrl Pts',(-0.246288608374016,0.0753584670996666,
-0.700025977406992));
#28008=CARTESIAN_POINT('Ctrl Pts',(-0.209097267103025,0.151167615813192,
-0.702473232900967));
#28009=CARTESIAN_POINT('Ctrl Pts',(-0.148976321364386,0.196701557847517,
-0.704920488394942));
#28010=CARTESIAN_POINT('Ctrl Pts',(-0.0841165574382396,0.24582454975473,
-0.707560640036871));
#28011=CARTESIAN_POINT('Ctrl Pts',(0.00742995623837037,0.259711571262569,
-0.710200791678799));
#28012=CARTESIAN_POINT('Ctrl Pts',(0.0839399555978737,0.232033469657142,
-0.712840943320728));
#28013=CARTESIAN_POINT('Ctrl Pts',(0.160449954957377,0.204355368051715,
-0.715481094962656));
#28014=CARTESIAN_POINT('Ctrl Pts',(0.221923439999773,0.135112143333024,
-0.718121246604584));
#28015=CARTESIAN_POINT('Ctrl Pts',(0.240343238398454,0.0558621065038622,
-0.720761398246513));
#28016=CARTESIAN_POINT('Ctrl Pts',(0.258763036797135,-0.0233879303253011,
-0.723401549888442));
#28017=CARTESIAN_POINT('Ctrl Pts',(0.234129148552099,-0.112644779264936,
-0.726041701530371));
#28018=CARTESIAN_POINT('Ctrl Pts',(0.177668721295525,-0.171228714473122,
-0.728681853172299));
#28019=CARTESIAN_POINT('Ctrl Pts',(0.121208294038953,-0.229812649681307,
-0.731322004814228));
#28020=CARTESIAN_POINT('Ctrl Pts',(0.0329213277708455,-0.257723671158046,
-0.733962156456156));
#28021=CARTESIAN_POINT('Ctrl Pts',(-0.0469544856580573,-0.242241044134746,
-0.736602308098085));
#28022=CARTESIAN_POINT('Ctrl Pts',(-0.12683029908696,-0.226758417111446,
-0.739242459740013));
#28023=CARTESIAN_POINT('Ctrl Pts',(-0.198294959676658,-0.167882141588106,
-0.741882611381942));
#28024=CARTESIAN_POINT('Ctrl Pts',(-0.228777714205282,-0.0924456849718314,
-0.744522763023871));
#28025=CARTESIAN_POINT('Ctrl Pts',(-0.240538912967255,-0.0633399439099515,
-0.74554141598692));
#28026=CARTESIAN_POINT('Ctrl Pts',(-0.246199309945309,-0.0317689592304798,
-0.746560068949969));
#28027=CARTESIAN_POINT('Ctrl Pts',(-0.246033746957446,-0.000140975359651019,
-0.747578721913017));
#28028=CARTESIAN_POINT('Ctrl Pts',(-0.246056814395214,-0.000156261806827737,
-0.754721278086983));
#28029=CARTESIAN_POINT('Ctrl Pts',(-0.24623408801582,-0.0305245395759718,
-0.7537429666777));
#28030=CARTESIAN_POINT('Ctrl Pts',(-0.241026159380574,-0.0608341650313951,
-0.752764655268417));
#28031=CARTESIAN_POINT('Ctrl Pts',(-0.230157149346615,-0.0889557814626542,
-0.751786343859135));
#28032=CARTESIAN_POINT('Ctrl Pts',(-0.20082514481818,-0.164847088760323,
-0.749146192217206));
#28033=CARTESIAN_POINT('Ctrl Pts',(-0.130264130258884,-0.224803375935269,
-0.746506040575278));
#28034=CARTESIAN_POINT('Ctrl Pts',(-0.0506330129290607,-0.241498949175182,
-0.743865888933349));
#28035=CARTESIAN_POINT('Ctrl Pts',(0.028998104400764,-0.258194522415096,
-0.741225737291421));
#28036=CARTESIAN_POINT('Ctrl Pts',(0.117699324501114,-0.231629381719977,
-0.738585585649492));
#28037=CARTESIAN_POINT('Ctrl Pts',(0.175044155081566,-0.17391086286593,
-0.735945434007563));
#28038=CARTESIAN_POINT('Ctrl Pts',(0.232388985662017,-0.116192344011885,
-0.733305282365635));
#28039=CARTESIAN_POINT('Ctrl Pts',(0.258377426722569,-0.0273204469989132,
-0.730665130723706));
#28040=CARTESIAN_POINT('Ctrl Pts',(0.24116497927002,0.0522005481262653,
-0.728024979081777));
#28041=CARTESIAN_POINT('Ctrl Pts',(0.22395253181747,0.131721543251444,-0.725384827439849));
#28042=CARTESIAN_POINT('Ctrl Pts',(0.163539195851817,0.201891636488831,
-0.72274467579792));
#28043=CARTESIAN_POINT('Ctrl Pts',(0.0874589698670081,0.230730086986491,
-0.720104524155991));
#28044=CARTESIAN_POINT('Ctrl Pts',(0.0113787438821998,0.25956853748415,
-0.717464372514063));
#28045=CARTESIAN_POINT('Ctrl Pts',(-0.0803683721217641,0.247075345242084,
-0.714824220872134));
#28046=CARTESIAN_POINT('Ctrl Pts',(-0.145967687505829,0.198944410967467,
-0.712184069230205));
#28047=CARTESIAN_POINT('Ctrl Pts',(-0.207776509655161,0.153594602984812,
-0.709696472182465));
#28048=CARTESIAN_POINT('Ctrl Pts',(-0.246371999630066,0.0766065415301417,
-0.707208875134724));
#28049=CARTESIAN_POINT('Ctrl Pts',(-0.24671395673833,-8.44291920866902E-5,
-0.704721278086983));
#28050=CARTESIAN_POINT('Origin',(0.,0.,-0.58));
#28051=CARTESIAN_POINT('',(-0.246332988773408,0.00022261242931975,-0.647578721913017));
#28052=CARTESIAN_POINT('',(-0.246295889561636,0.000221807446104811,-0.654721278086982));
#28053=CARTESIAN_POINT('',(-0.24635,-3.0169173896995E-17,-0.58));
#28054=CARTESIAN_POINT('Ctrl Pts',(-0.246332988773408,0.00022261242931975,
-0.647578721913017));
#28055=CARTESIAN_POINT('Ctrl Pts',(-0.246510645363659,0.0198118416510094,
-0.648211582580158));
#28056=CARTESIAN_POINT('Ctrl Pts',(-0.244369383537724,0.0393627020095402,
-0.648844443247299));
#28057=CARTESIAN_POINT('Ctrl Pts',(-0.23976029777941,0.0583133500635451,
-0.64947730391444));
#28058=CARTESIAN_POINT('Ctrl Pts',(-0.220532233903086,0.137371169854126,
-0.652117455556369));
#28059=CARTESIAN_POINT('Ctrl Pts',(-0.158354907967284,0.2059830760525,-0.654757607198297));
#28060=CARTESIAN_POINT('Ctrl Pts',(-0.0815662750163546,0.232878487557055,
-0.657397758840226));
#28061=CARTESIAN_POINT('Ctrl Pts',(-0.00477764206542863,0.259773899061609,
-0.660037910482155));
#28062=CARTESIAN_POINT('Ctrl Pts',(0.0866222979006217,0.244952815872347,
-0.662678062124084));
#28063=CARTESIAN_POINT('Ctrl Pts',(0.15097708328857,0.195170098910107,-0.665318213766013));
#28064=CARTESIAN_POINT('Ctrl Pts',(0.215331868676519,0.145387381947866,
-0.667958365407941));
#28065=CARTESIAN_POINT('Ctrl Pts',(0.252641499486365,0.0606430312126439,
-0.67059851704987));
#28066=CARTESIAN_POINT('Ctrl Pts',(0.245901728193816,-0.0204398448673013,
-0.673238668691798));
#28067=CARTESIAN_POINT('Ctrl Pts',(0.239161956901268,-0.101522720947246,
-0.675878820333726));
#28068=CARTESIAN_POINT('Ctrl Pts',(0.188372783506328,-0.178944122371914,
-0.678518971975655));
#28069=CARTESIAN_POINT('Ctrl Pts',(0.116681895542094,-0.217418450090163,
-0.681159123617584));
#28070=CARTESIAN_POINT('Ctrl Pts',(0.0449910075778601,-0.255892777808412,
-0.683799275259513));
#28071=CARTESIAN_POINT('Ctrl Pts',(-0.0476015949556688,-0.255420031820241,
-0.686439426901442));
#28072=CARTESIAN_POINT('Ctrl Pts',(-0.118895882247883,-0.216215670966289,
-0.68907957854337));
#28073=CARTESIAN_POINT('Ctrl Pts',(-0.190190169540097,-0.177011310112337,
-0.691719730185299));
#28074=CARTESIAN_POINT('Ctrl Pts',(-0.240186141590997,-0.0990753343926033,
-0.694359881827227));
#28075=CARTESIAN_POINT('Ctrl Pts',(-0.246097620528605,-0.0179278653794423,
-0.697000033469156));
#28076=CARTESIAN_POINT('Ctrl Pts',(-0.246529528112119,-0.0119990263157112,
-0.69719292961711));
#28077=CARTESIAN_POINT('Ctrl Pts',(-0.246726106821209,-0.00605304387460213,
-0.697385825765063));
#28078=CARTESIAN_POINT('Ctrl Pts',(-0.246694142079541,-0.000104913238225313,
-0.697578721913017));
#28079=CARTESIAN_POINT('Ctrl Pts',(-0.24671395673833,-8.44291920866902E-5,
-0.704721278086983));
#28080=CARTESIAN_POINT('Ctrl Pts',(-0.246734927629869,-0.00478758637222922,
-0.704568723492795));
#28081=CARTESIAN_POINT('Ctrl Pts',(-0.246612031230182,-0.00948962622710204,
-0.704416168898608));
#28082=CARTESIAN_POINT('Ctrl Pts',(-0.246341798658231,-0.0141831831694928,
-0.70426361430442));
#28083=CARTESIAN_POINT('Ctrl Pts',(-0.241665079662402,-0.0954111667246658,
-0.701623462662492));
#28084=CARTESIAN_POINT('Ctrl Pts',(-0.19286012690658,-0.174098457527845,
-0.698983311020563));
#28085=CARTESIAN_POINT('Ctrl Pts',(-0.122170298983642,-0.214382514439119,
-0.696343159378634));
#28086=CARTESIAN_POINT('Ctrl Pts',(-0.0514804710607036,-0.254666571350394,
-0.693703007736705));
#28087=CARTESIAN_POINT('Ctrl Pts',(0.0410942320293508,-0.256547394369764,
-0.691062856094777));
#28088=CARTESIAN_POINT('Ctrl Pts',(0.113361938331161,-0.219167779084413,
-0.688422704452848));
#28089=CARTESIAN_POINT('Ctrl Pts',(0.185629644632971,-0.181788163799061,
-0.68578255281092));
#28090=CARTESIAN_POINT('Ctrl Pts',(0.237590354146535,-0.105148110208987,
-0.683142401168991));
#28091=CARTESIAN_POINT('Ctrl Pts',(0.245562439717473,-0.0241771100629151,
-0.680502249527062));
#28092=CARTESIAN_POINT('Ctrl Pts',(0.25353452528841,0.0567938900831571,
-0.677862097885134));
#28093=CARTESIAN_POINT('Ctrl Pts',(0.217517986916721,0.142095836785229,
-0.675221946243205));
#28094=CARTESIAN_POINT('Ctrl Pts',(0.153927731964037,0.192851491524954,
-0.672581794601276));
#28095=CARTESIAN_POINT('Ctrl Pts',(0.0903374770113528,0.243607146264678,
-0.669941642959348));
#28096=CARTESIAN_POINT('Ctrl Pts',(-0.000826494522324708,0.259816509042058,
-0.667301491317419));
#28097=CARTESIAN_POINT('Ctrl Pts',(-0.0780152660809326,0.234091996252142,
-0.66466133967549));
#28098=CARTESIAN_POINT('Ctrl Pts',(-0.15520403763954,0.208367483462227,
-0.662021188033562));
#28099=CARTESIAN_POINT('Ctrl Pts',(-0.218417609223077,0.140709095105016,
-0.659381036391633));
#28100=CARTESIAN_POINT('Ctrl Pts',(-0.23884574618786,0.0619528367305004,
-0.656740884749705));
#28101=CARTESIAN_POINT('Ctrl Pts',(-0.244054639099651,0.0418710780897904,
-0.656067682528797));
#28102=CARTESIAN_POINT('Ctrl Pts',(-0.246481710354252,0.0210677585852516,
-0.65539448030789));
#28103=CARTESIAN_POINT('Ctrl Pts',(-0.246295889561636,0.000221807446104811,
-0.654721278086982));
#28104=CARTESIAN_POINT('Origin',(0.,0.,-0.58));
#28105=CARTESIAN_POINT('',(-0.245967927871332,-6.88792904169344E-5,-0.597578721913017));
#28106=CARTESIAN_POINT('',(-0.245979910166711,-8.79836153418138E-5,-0.604721278086982));
#28107=CARTESIAN_POINT('',(-0.24635,-3.0169173896995E-17,-0.58));
#28108=CARTESIAN_POINT('Ctrl Pts',(-0.245967927871332,-6.88792904169344E-5,
-0.597578721913017));
#28109=CARTESIAN_POINT('Ctrl Pts',(-0.245853915264038,0.0452498307293128,
-0.599037339395253));
#28110=CARTESIAN_POINT('Ctrl Pts',(-0.233865752530936,0.0906246440450581,
-0.600495956877489));
#28111=CARTESIAN_POINT('Ctrl Pts',(-0.210374949312293,0.128948935198221,
-0.601954574359725));
#28112=CARTESIAN_POINT('Ctrl Pts',(-0.167855725839909,0.198317320978612,
-0.604594726001654));
#28113=CARTESIAN_POINT('Ctrl Pts',(-0.0876511603303029,0.244586546216524,
-0.607234877643583));
#28114=CARTESIAN_POINT('Ctrl Pts',(-0.00631530745783936,0.246668936184956,
-0.609875029285512));
#28115=CARTESIAN_POINT('Ctrl Pts',(0.0750205454146241,0.248751326153387,
-0.61251518092744));
#28116=CARTESIAN_POINT('Ctrl Pts',(0.157487685649946,0.206646880852338,
-0.615155332569368));
#28117=CARTESIAN_POINT('Ctrl Pts',(0.203500866899034,0.139545133767704,
-0.617795484211297));
#28118=CARTESIAN_POINT('Ctrl Pts',(0.249514048148123,0.0724433866830698,
-0.620435635853225));
#28119=CARTESIAN_POINT('Ctrl Pts',(0.259073270410978,-0.0196556621851494,
-0.623075787495155));
#28120=CARTESIAN_POINT('Ctrl Pts',(0.227821819939192,-0.0947769251795984,
-0.625715939137083));
#28121=CARTESIAN_POINT('Ctrl Pts',(0.196570369467406,-0.169898188174047,
-0.628356090779012));
#28122=CARTESIAN_POINT('Ctrl Pts',(0.124508246260982,-0.228041665294725,
-0.63099624242094));
#28123=CARTESIAN_POINT('Ctrl Pts',(0.0444785032671047,-0.242707869534597,
-0.633636394062869));
#28124=CARTESIAN_POINT('Ctrl Pts',(-0.0355512397267712,-0.257374073774469,
-0.636276545704797));
#28125=CARTESIAN_POINT('Ctrl Pts',(-0.123548602508098,-0.228563005133535,
-0.638916697346726));
#28126=CARTESIAN_POINT('Ctrl Pts',(-0.179407882990338,-0.169405604121676,
-0.641556848988655));
#28127=CARTESIAN_POINT('Ctrl Pts',(-0.22187734867914,-0.12442859777963,
-0.643564139963442));
#28128=CARTESIAN_POINT('Ctrl Pts',(-0.245769502229312,-0.0619099944166167,
-0.64557143093823));
#28129=CARTESIAN_POINT('Ctrl Pts',(-0.246332988773408,0.00022261242931975,
-0.647578721913017));
#28130=CARTESIAN_POINT('Ctrl Pts',(-0.246295889561636,0.000221807446104811,
-0.654721278086982));
#28131=CARTESIAN_POINT('Ctrl Pts',(-0.245752961910631,-0.0606854953677682,
-0.652754328665961));
#28132=CARTESIAN_POINT('Ctrl Pts',(-0.222904287268899,-0.121956736085764,
-0.65078737924494));
#28133=CARTESIAN_POINT('Ctrl Pts',(-0.181963421308779,-0.166657606356852,
-0.648820429823918));
#28134=CARTESIAN_POINT('Ctrl Pts',(-0.127010257118888,-0.226657662677861,
-0.64618027818199));
#28135=CARTESIAN_POINT('Ctrl Pts',(-0.0394612263930818,-0.256803646928059,
-0.643540126540062));
#28136=CARTESIAN_POINT('Ctrl Pts',(0.0407823007221384,-0.243356217095025,
-0.640899974898133));
#28137=CARTESIAN_POINT('Ctrl Pts',(0.121025827837359,-0.229908787261991,
-0.638259823256204));
#28138=CARTESIAN_POINT('Ctrl Pts',(0.193963851341991,-0.17286794334572,
-0.635619671614275));
#28139=CARTESIAN_POINT('Ctrl Pts',(0.22635411772979,-0.0982306359429682,
-0.632979519972347));
#28140=CARTESIAN_POINT('Ctrl Pts',(0.258744384117589,-0.0235933285402166,
-0.630339368330418));
#28141=CARTESIAN_POINT('Ctrl Pts',(0.250586893388558,0.0686404423490178,
-0.62769921668849));
#28142=CARTESIAN_POINT('Ctrl Pts',(0.205599505744543,0.136434188122301,
-0.625059065046561));
#28143=CARTESIAN_POINT('Ctrl Pts',(0.160612118100527,0.204227933895586,
-0.622418913404633));
#28144=CARTESIAN_POINT('Ctrl Pts',(0.0787948335415277,0.247581654552918,
-0.619778761762704));
#28145=CARTESIAN_POINT('Ctrl Pts',(-0.00256327998383143,0.246736446530942,
-0.617138610120775));
#28146=CARTESIAN_POINT('Ctrl Pts',(-0.0839213935091894,0.245891238508966,
-0.614498458478847));
#28147=CARTESIAN_POINT('Ctrl Pts',(-0.164820336000906,0.200847101807682,
-0.611858306836918));
#28148=CARTESIAN_POINT('Ctrl Pts',(-0.208389583341672,0.132133364468162,
-0.609218155194989));
#28149=CARTESIAN_POINT('Ctrl Pts',(-0.233126237083863,0.0931208032778008,
-0.607719196158987));
#28150=CARTESIAN_POINT('Ctrl Pts',(-0.245829826783415,0.0464784497949531,
-0.606220237122985));
#28151=CARTESIAN_POINT('Ctrl Pts',(-0.245979910166711,-8.79836153418138E-5,
-0.604721278086982));
#28152=CARTESIAN_POINT('Origin',(0.,0.,-0.58));
#28153=CARTESIAN_POINT('',(-0.246582462449767,-0.000173722512632146,-0.547578721913017));
#28154=CARTESIAN_POINT('',(-0.246614023415026,-0.000159075665185677,-0.554721278086982));
#28155=CARTESIAN_POINT('',(-0.24635,-3.0169173896995E-17,-0.58));
#28156=CARTESIAN_POINT('Ctrl Pts',(-0.246582462449767,-0.000173722512632146,
-0.547578721913017));
#28157=CARTESIAN_POINT('Ctrl Pts',(-0.246017207900454,0.0703510165357913,
-0.549863096210348));
#28158=CARTESIAN_POINT('Ctrl Pts',(-0.214171831893926,0.141321641909776,
-0.55214747050768));
#28159=CARTESIAN_POINT('Ctrl Pts',(-0.160766372533128,0.187188730027863,
-0.554431844805011));
#28160=CARTESIAN_POINT('Ctrl Pts',(-0.0990433390599819,0.240199336979155,
-0.557071996446939));
#28161=CARTESIAN_POINT('Ctrl Pts',(-0.00852155480020805,0.259678046051574,
-0.559712148088867));
#28162=CARTESIAN_POINT('Ctrl Pts',(0.0695427471374144,0.236747235480135,
-0.562352299730796));
#28163=CARTESIAN_POINT('Ctrl Pts',(0.147607049075037,0.213816424908696,
-0.564992451372724));
#28164=CARTESIAN_POINT('Ctrl Pts',(0.213213868690508,0.148476094693399,
-0.567632603014654));
#28165=CARTESIAN_POINT('Ctrl Pts',(0.236462223963698,0.0705057715725927,
-0.570272754656582));
#28166=CARTESIAN_POINT('Ctrl Pts',(0.259710579236889,-0.00746455154821403,
-0.572912906298511));
#28167=CARTESIAN_POINT('Ctrl Pts',(0.240600470167799,-0.0980648675745309,
-0.575553057940439));
#28168=CARTESIAN_POINT('Ctrl Pts',(0.18784152528326,-0.160003151738218,
-0.578193209582367));
#28169=CARTESIAN_POINT('Ctrl Pts',(0.13508258039872,-0.221941435901907,
-0.580833361224296));
#28170=CARTESIAN_POINT('Ctrl Pts',(0.0486747996987275,-0.255217688202964,
-0.583473512866225));
#28171=CARTESIAN_POINT('Ctrl Pts',(-0.0320005830935595,-0.244665914807472,
-0.586113664508154));
#28172=CARTESIAN_POINT('Ctrl Pts',(-0.112675965885844,-0.23411414141198,
-0.588753816150082));
#28173=CARTESIAN_POINT('Ctrl Pts',(-0.187618950770424,-0.17973434231994,
-0.591393967792011));
#28174=CARTESIAN_POINT('Ctrl Pts',(-0.222673502495132,-0.106310669612487,
-0.59403411943394));
#28175=CARTESIAN_POINT('Ctrl Pts',(-0.238361294687702,-0.0734517322483565,
-0.595215653593632));
#28176=CARTESIAN_POINT('Ctrl Pts',(-0.246060282304069,-0.0367787121380407,
-0.596397187753325));
#28177=CARTESIAN_POINT('Ctrl Pts',(-0.245967927871332,-6.88792904169344E-5,
-0.597578721913017));
#28178=CARTESIAN_POINT('Ctrl Pts',(-0.245979910166711,-8.79836153418138E-5,
-0.604721278086982));
#28179=CARTESIAN_POINT('Ctrl Pts',(-0.246094172159986,-0.0355400995276661,
-0.603580085481056));
#28180=CARTESIAN_POINT('Ctrl Pts',(-0.238932254481067,-0.0709482111534824,
-0.60243889287513));
#28181=CARTESIAN_POINT('Ctrl Pts',(-0.224264499901541,-0.10291199412558,
-0.601297700269203));
#28182=CARTESIAN_POINT('Ctrl Pts',(-0.190330616930831,-0.17686027740204,
-0.598657548627275));
#28183=CARTESIAN_POINT('Ctrl Pts',(-0.116223298799597,-0.232373505977202,
-0.596017396985346));
#28184=CARTESIAN_POINT('Ctrl Pts',(-0.0357177170523464,-0.244150955639253,
-0.593377245343418));
#28185=CARTESIAN_POINT('Ctrl Pts',(0.0447878646949057,-0.255928405301304,
-0.590737093701489));
#28186=CARTESIAN_POINT('Ctrl Pts',(0.131691710058175,-0.223970076050241,
-0.58809694205956));
#28187=CARTESIAN_POINT('Ctrl Pts',(0.185386498747934,-0.162841304750895,
-0.585456790417632));
#28188=CARTESIAN_POINT('Ctrl Pts',(0.239081287437692,-0.10171253345155,
-0.582816638775703));
#28189=CARTESIAN_POINT('Ctrl Pts',(0.259567019453941,-0.011413320103922,
-0.580176487133774));
#28190=CARTESIAN_POINT('Ctrl Pts',(0.237507111979875,0.0669015411628969,
-0.577536335491846));
#28191=CARTESIAN_POINT('Ctrl Pts',(0.215447204505809,0.145216402429716,
-0.574896183849917));
#28192=CARTESIAN_POINT('Ctrl Pts',(0.150841657541429,0.211546911615725,
-0.572256032207989));
#28193=CARTESIAN_POINT('Ctrl Pts',(0.0731351128100314,0.235662257744544,
-0.56961588056606));
#28194=CARTESIAN_POINT('Ctrl Pts',(-0.00457143192136621,0.259777603873362,
-0.566975728924132));
#28195=CARTESIAN_POINT('Ctrl Pts',(-0.0953789744197813,0.24167778694499,
-0.564335577282203));
#28196=CARTESIAN_POINT('Ctrl Pts',(-0.157901044323573,0.189611984464371,
-0.561695425640274));
#28197=CARTESIAN_POINT('Ctrl Pts',(-0.212953202934656,0.143766816177604,
-0.559370709789177));
#28198=CARTESIAN_POINT('Ctrl Pts',(-0.24607501730235,0.0715870779721306,
-0.55704599393808));
#28199=CARTESIAN_POINT('Ctrl Pts',(-0.246614023415026,-0.000159075665185677,
-0.554721278086982));
#28200=CARTESIAN_POINT('Origin',(0.,0.,-0.58));
#28201=CARTESIAN_POINT('',(-0.246483938463648,0.00020522848325015,-0.497578721913017));
#28202=CARTESIAN_POINT('',(-0.246447022145754,0.000212618034880898,-0.504721278086982));
#28203=CARTESIAN_POINT('',(-0.24635,-3.0169173896995E-17,-0.58));
#28204=CARTESIAN_POINT('Ctrl Pts',(-0.246483938463648,0.00020522848325015,
-0.497578721913017));
#28205=CARTESIAN_POINT('Ctrl Pts',(-0.246613670338324,0.0147298283212238,
-0.498048701383514));
#28206=CARTESIAN_POINT('Ctrl Pts',(-0.245439652456884,0.0292334866156357,
-0.498518680854012));
#28207=CARTESIAN_POINT('Ctrl Pts',(-0.242886894023589,0.0434902736077678,
-0.498988660324509));
#28208=CARTESIAN_POINT('Ctrl Pts',(-0.228546545578205,0.123579047583505,
-0.501628811966438));
#28209=CARTESIAN_POINT('Ctrl Pts',(-0.170696854848679,0.195877227472071,
-0.504268963608366));
#28210=CARTESIAN_POINT('Ctrl Pts',(-0.0957034126762081,0.227434175068375,
-0.506909115250295));
#28211=CARTESIAN_POINT('Ctrl Pts',(-0.0207099705037368,0.258991122664679,
-0.509549266892224));
#28212=CARTESIAN_POINT('Ctrl Pts',(0.0714272231116802,0.249806837968721,
-0.512189418534152));
#28213=CARTESIAN_POINT('Ctrl Pts',(0.138715695652291,0.204067153081053,
-0.514829570176081));
#28214=CARTESIAN_POINT('Ctrl Pts',(0.206004168192901,0.158327468193386,
-0.51746972181801));
#28215=CARTESIAN_POINT('Ctrl Pts',(0.248443919658705,0.0760323831140095,
-0.520109873459938));
#28216=CARTESIAN_POINT('Ctrl Pts',(0.246692597334613,-0.00531127171283383,
-0.522750025101867));
#28217=CARTESIAN_POINT('Ctrl Pts',(0.244941275010521,-0.0866549265396772,
-0.525390176743795));
#28218=CARTESIAN_POINT('Ctrl Pts',(0.198998878896533,-0.167047151113988,
-0.528030328385724));
#28219=CARTESIAN_POINT('Ctrl Pts',(0.129804127988899,-0.209848363214838,
-0.530670480027653));
#28220=CARTESIAN_POINT('Ctrl Pts',(0.0606093770812643,-0.252649575315688,
-0.533310631669581));
#28221=CARTESIAN_POINT('Ctrl Pts',(-0.031837728620016,-0.257859774943077,
-0.53595078331151));
#28222=CARTESIAN_POINT('Ctrl Pts',(-0.105403470980325,-0.223104360092322,
-0.538590934953439));
#28223=CARTESIAN_POINT('Ctrl Pts',(-0.178969213340635,-0.188348945241567,
-0.541231086595367));
#28224=CARTESIAN_POINT('Ctrl Pts',(-0.233653592359973,-0.113627915912667,
-0.543871238237295));
#28225=CARTESIAN_POINT('Ctrl Pts',(-0.244533640526383,-0.032996148833134,
-0.546511389879224));
#28226=CARTESIAN_POINT('Ctrl Pts',(-0.245999796706303,-0.0221305017520405,
-0.546867167223822));
#28227=CARTESIAN_POINT('Ctrl Pts',(-0.246670497393433,-0.011157519877363,
-0.547222944568419));
#28228=CARTESIAN_POINT('Ctrl Pts',(-0.246582462449767,-0.000173722512632146,
-0.547578721913017));
#28229=CARTESIAN_POINT('Ctrl Pts',(-0.246614023415026,-0.000159075665185677,
-0.554721278086982));
#28230=CARTESIAN_POINT('Ctrl Pts',(-0.246687160017649,-0.00989415993408876,
-0.554405842296151));
#28231=CARTESIAN_POINT('Ctrl Pts',(-0.246160407898964,-0.0196212613891677,
-0.55409040650532));
#28232=CARTESIAN_POINT('Ctrl Pts',(-0.245007155314066,-0.0292735084317024,
-0.553774970714488));
#28233=CARTESIAN_POINT('Ctrl Pts',(-0.235354599091597,-0.110061410814284,
-0.55113481907256));
#28234=CARTESIAN_POINT('Ctrl Pts',(-0.181812889337495,-0.18560542754658,
-0.548494667430631));
#28235=CARTESIAN_POINT('Ctrl Pts',(-0.108784210307416,-0.221475596937413,
-0.545854515788702));
#28236=CARTESIAN_POINT('Ctrl Pts',(-0.0357555312773367,-0.257345766328247,
-0.543214364146774));
#28237=CARTESIAN_POINT('Ctrl Pts',(0.0567601170287202,-0.253542088377617,
-0.540574212504845));
#28238=CARTESIAN_POINT('Ctrl Pts',(0.12659777747987,-0.211798128386795,
-0.537934060862917));
#28239=CARTESIAN_POINT('Ctrl Pts',(0.19643543793102,-0.170054168395972,
-0.535293909220988));
#28240=CARTESIAN_POINT('Ctrl Pts',(0.243595110527264,-0.090369926364956,
-0.532653757579059));
#28241=CARTESIAN_POINT('Ctrl Pts',(0.246583290010452,-0.0090623141974485,
-0.530013605937131));
#28242=CARTESIAN_POINT('Ctrl Pts',(0.24957146949364,0.0722452979700579,
-0.527373454295202));
#28243=CARTESIAN_POINT('Ctrl Pts',(0.208388155863774,0.155176280274057,
-0.524733302653273));
#28244=CARTESIAN_POINT('Ctrl Pts',(0.141803067384801,0.201933985577598,
-0.522093151011345));
#28245=CARTESIAN_POINT('Ctrl Pts',(0.0752179789058258,0.24869169088114,
-0.519452999369416));
#28246=CARTESIAN_POINT('Ctrl Pts',(-0.0167688844222544,0.259276119184221,
-0.516812847727488));
#28247=CARTESIAN_POINT('Ctrl Pts',(-0.0922335646544927,0.228863308553637,
-0.514172696085559));
#28248=CARTESIAN_POINT('Ctrl Pts',(-0.167698244886729,0.198450497923054,
-0.51153254444363));
#28249=CARTESIAN_POINT('Ctrl Pts',(-0.226640742023121,0.127040448358805,
-0.508892392801702));
#28250=CARTESIAN_POINT('Ctrl Pts',(-0.24219740747612,0.0471790235468913,
-0.506252241159773));
#28251=CARTESIAN_POINT('Ctrl Pts',(-0.24520439136372,0.0317424238221111,
-0.50574192013551));
#28252=CARTESIAN_POINT('Ctrl Pts',(-0.246590397311392,0.0159900644977801,
-0.505231599111246));
#28253=CARTESIAN_POINT('Ctrl Pts',(-0.246447022145754,0.000212618034880898,
-0.504721278086982));
#28254=CARTESIAN_POINT('Origin',(0.,0.,-0.58));
#28255=CARTESIAN_POINT('',(-0.245950337987333,1.22903161040577E-5,-0.447578721913017));
#28256=CARTESIAN_POINT('',(-0.245950012479873,-8.08252214897014E-6,-0.454721278086982));
#28257=CARTESIAN_POINT('',(-0.24635,-3.0169173896995E-17,-0.58));
#28258=CARTESIAN_POINT('Ctrl Pts',(-0.245950337987333,1.22903161040577E-5,
-0.447578721913017));
#28259=CARTESIAN_POINT('Ctrl Pts',(-0.245968336645111,0.0402775323416728,
-0.448874458198609));
#28260=CARTESIAN_POINT('Ctrl Pts',(-0.236630669927586,0.0805349102977895,
-0.450170194484202));
#28261=CARTESIAN_POINT('Ctrl Pts',(-0.217891563823453,0.115795999937283,
-0.451465930769794));
#28262=CARTESIAN_POINT('Ctrl Pts',(-0.179709348584739,0.187642890962127,
-0.454106082411723));
#28263=CARTESIAN_POINT('Ctrl Pts',(-0.102495308803444,0.238746761591991,
-0.456746234053651));
#28264=CARTESIAN_POINT('Ctrl Pts',(-0.0214405363315153,0.245816497796063,
-0.45938638569558));
#28265=CARTESIAN_POINT('Ctrl Pts',(0.0596142361404157,0.252886234000135,
-0.462026537337508));
#28266=CARTESIAN_POINT('Ctrl Pts',(0.144509741302979,0.215921835778419,
-0.464666688979437));
#28267=CARTESIAN_POINT('Ctrl Pts',(0.194553980544851,0.151770207356578,
-0.467306840621366));
#28268=CARTESIAN_POINT('Ctrl Pts',(0.244598219786722,0.0876185789347377,
-0.469946992263295));
#28269=CARTESIAN_POINT('Ctrl Pts',(0.259791193107898,-0.00372027968722727,
-0.472587143905223));
#28270=CARTESIAN_POINT('Ctrl Pts',(0.233208546839486,-0.0806177453661419,
-0.475227295547151));
#28271=CARTESIAN_POINT('Ctrl Pts',(0.206625900571073,-0.15751521104506,
-0.47786744718908));
#28272=CARTESIAN_POINT('Ctrl Pts',(0.138267634713071,-0.219971283780928,
-0.480507598831009));
#28273=CARTESIAN_POINT('Ctrl Pts',(0.0592887311763125,-0.239520966811692,
-0.483147750472938));
#28274=CARTESIAN_POINT('Ctrl Pts',(-0.0196901723604435,-0.259070649842456,
-0.485787902114866));
#28275=CARTESIAN_POINT('Ctrl Pts',(-0.109289713575953,-0.235713943168118,
-0.488428053756795));
#28276=CARTESIAN_POINT('Ctrl Pts',(-0.168673981103086,-0.180095905799495,
-0.491068205398723));
#28277=CARTESIAN_POINT('Ctrl Pts',(-0.217487118485629,-0.134378563276385,
-0.493238377570155));
#28278=CARTESIAN_POINT('Ctrl Pts',(-0.245884889948035,-0.0668634082301429,
-0.495408549741586));
#28279=CARTESIAN_POINT('Ctrl Pts',(-0.246483938463648,0.00020522848325015,
-0.497578721913017));
#28280=CARTESIAN_POINT('Ctrl Pts',(-0.246447022145754,0.000212618034880898,
-0.504721278086982));
#28281=CARTESIAN_POINT('Ctrl Pts',(-0.245848644256014,-0.065634734802945,
-0.502591447469317));
#28282=CARTESIAN_POINT('Ctrl Pts',(-0.218611204094641,-0.131919060374852,
-0.500461616851652));
#28283=CARTESIAN_POINT('Ctrl Pts',(-0.171393337184106,-0.17750991076525,
-0.498331786233988));
#28284=CARTESIAN_POINT('Ctrl Pts',(-0.112861767669489,-0.2340246202059,
-0.495691634592059));
#28285=CARTESIAN_POINT('Ctrl Pts',(-0.0236277948706488,-0.25874123902762,
-0.49305148295013));
#28286=CARTESIAN_POINT('Ctrl Pts',(0.0556392814066714,-0.240394914288013,
-0.490411331308201));
#28287=CARTESIAN_POINT('Ctrl Pts',(0.13490635768399,-0.222048589548406,
-0.487771179666273));
#28288=CARTESIAN_POINT('Ctrl Pts',(0.20420653743979,-0.160639321247473,
-0.485131028024344));
#28289=CARTESIAN_POINT('Ctrl Pts',(0.231955551828012,-0.0841550142722008,
-0.482490876382416));
#28290=CARTESIAN_POINT('Ctrl Pts',(0.259704566216234,-0.00767070729692744,
-0.479850724740487));
#28291=CARTESIAN_POINT('Ctrl Pts',(0.245902415236877,0.0838886383526858,
-0.477210573098558));
#28292=CARTESIAN_POINT('Ctrl Pts',(0.196839570988601,0.148793910305548,
-0.47457042145663));
#28293=CARTESIAN_POINT('Ctrl Pts',(0.147776726740325,0.213699182258409,
-0.471930269814701));
#28294=CARTESIAN_POINT('Ctrl Pts',(0.0634531892231296,0.251950380514519,
-0.469290118172773));
#28295=CARTESIAN_POINT('Ctrl Pts',(-0.0176997230818681,0.24611412851321,
-0.466649966530844));
#28296=CARTESIAN_POINT('Ctrl Pts',(-0.0988526353868669,0.240277876511901,
-0.464009814888915));
#28297=CARTESIAN_POINT('Ctrl Pts',(-0.176834922479668,0.190354174253172,
-0.461369663246987));
#28298=CARTESIAN_POINT('Ctrl Pts',(-0.216105355903885,0.119096261908789,
-0.458729511605058));
#28299=CARTESIAN_POINT('Ctrl Pts',(-0.235978591594914,0.0830354099295665,
-0.457393433765699));
#28300=CARTESIAN_POINT('Ctrl Pts',(-0.245937808335925,0.0415109145690796,
-0.456057355926341));
#28301=CARTESIAN_POINT('Ctrl Pts',(-0.245950012479873,-8.08252214897014E-6,
-0.454721278086982));
#28302=CARTESIAN_POINT('Origin',(0.,0.,-0.58));
#28303=CARTESIAN_POINT('',(-0.246439321146211,-0.000213893874535243,-0.397578721913017));
#28304=CARTESIAN_POINT('',(-0.24647636517194,-0.000206920082869883,-0.404721278086982));
#28305=CARTESIAN_POINT('',(-0.24635,-3.0169173896995E-17,-0.58));
#28306=CARTESIAN_POINT('Ctrl Pts',(-0.246439321146211,-0.000213893874535243,
-0.397578721913017));
#28307=CARTESIAN_POINT('Ctrl Pts',(-0.245841811704369,0.065380979190444,
-0.399700215013704));
#28308=CARTESIAN_POINT('Ctrl Pts',(-0.21884049345472,0.131410332468187,
-0.401821708114392));
#28309=CARTESIAN_POINT('Ctrl Pts',(-0.171950437287423,0.17697032040308,
-0.403943201215079));
#28310=CARTESIAN_POINT('Ctrl Pts',(-0.113596790631628,0.233668726310498,
-0.406583352857008));
#28311=CARTESIAN_POINT('Ctrl Pts',(-0.0244409450267208,0.258665700670919,
-0.409223504498936));
#28312=CARTESIAN_POINT('Ctrl Pts',(0.0548834069927918,0.240568615625082,
-0.411863656140865));
#28313=CARTESIAN_POINT('Ctrl Pts',(0.134207759012302,0.222471530579245,
-0.414503807782794));
#28314=CARTESIAN_POINT('Ctrl Pts',(0.20370061744642,0.161280386127154,-0.417143959424722));
#28315=CARTESIAN_POINT('Ctrl Pts',(0.231689898162049,0.0848836749708929,
-0.419784111066651));
#28316=CARTESIAN_POINT('Ctrl Pts',(0.259679178877679,0.00848696381463214,
-0.422424262708579));
#28317=CARTESIAN_POINT('Ctrl Pts',(0.246164881874822,-0.0831153140457956,
-0.425064414350508));
#28318=CARTESIAN_POINT('Ctrl Pts',(0.197306286845217,-0.148174479443182,
-0.427704565992436));
#28319=CARTESIAN_POINT('Ctrl Pts',(0.148447691815611,-0.213233644840569,
-0.430344717634365));
#28320=CARTESIAN_POINT('Ctrl Pts',(0.064244798759254,-0.251749697774912,
-0.432984869276294));
#28321=CARTESIAN_POINT('Ctrl Pts',(-0.0169260587951456,-0.246168551445078,
-0.435625020918222));
#28322=CARTESIAN_POINT('Ctrl Pts',(-0.0980969163495463,-0.240587405115244,
-0.438265172560151));
#28323=CARTESIAN_POINT('Ctrl Pts',(-0.176235738401991,-0.190909059521233,
-0.440905324202079));
#28324=CARTESIAN_POINT('Ctrl Pts',(-0.215729954080146,-0.119774931014312,
-0.443545475844008));
#28325=CARTESIAN_POINT('Ctrl Pts',(-0.235841158755259,-0.0835520818394694,
-0.444889891200344));
#28326=CARTESIAN_POINT('Ctrl Pts',(-0.245931663144173,-0.0417656627347477,
-0.446234306556681));
#28327=CARTESIAN_POINT('Ctrl Pts',(-0.245950337987333,1.22903161040577E-5,
-0.447578721913017));
#28328=CARTESIAN_POINT('Ctrl Pts',(-0.245950012479873,-8.08252214897014E-6,
-0.454721278086982));
#28329=CARTESIAN_POINT('Ctrl Pts',(-0.245961924289152,-0.0405325451100766,
-0.453417204284412));
#28330=CARTESIAN_POINT('Ctrl Pts',(-0.236497652040484,-0.0810517696819681,
-0.452113130481842));
#28331=CARTESIAN_POINT('Ctrl Pts',(-0.217526516708852,-0.116480294382806,
-0.450809056679272));
#28332=CARTESIAN_POINT('Ctrl Pts',(-0.179118664333969,-0.188206815899989,
-0.448168905037344));
#28333=CARTESIAN_POINT('Ctrl Pts',(-0.101744379828568,-0.239067736504317,
-0.445528753395415));
#28334=CARTESIAN_POINT('Ctrl Pts',(-0.0206677882238031,-0.245882669134951,
-0.442888601753486));
#28335=CARTESIAN_POINT('Ctrl Pts',(0.0604088033809579,-0.252697601765584,
-0.440248450111558));
#28336=CARTESIAN_POINT('Ctrl Pts',(0.14518770208508,-0.215466546422527,
-0.437608298469629));
#28337=CARTESIAN_POINT('Ctrl Pts',(0.195030053868572,-0.151157939053871,
-0.4349681468277));
#28338=CARTESIAN_POINT('Ctrl Pts',(0.244872405652064,-0.0868493316852137,
-0.432327995185772));
#28339=CARTESIAN_POINT('Ctrl Pts',(0.259778210514923,0.00453682770904573,
-0.429687843543843));
#28340=CARTESIAN_POINT('Ctrl Pts',(0.232953994763222,0.0813503581728361,
-0.427047691901915));
#28341=CARTESIAN_POINT('Ctrl Pts',(0.20612977901152,0.158163888636627,-0.424407540259986));
#28342=CARTESIAN_POINT('Ctrl Pts',(0.137575542645258,0.220404790169951,
-0.421767388618057));
#28343=CARTESIAN_POINT('Ctrl Pts',(0.0585355831476179,0.239706132496772,
-0.419127236976129));
#28344=CARTESIAN_POINT('Ctrl Pts',(-0.0205043763500208,0.259007474823592,
-0.4164870853342));
#28345=CARTESIAN_POINT('Ctrl Pts',(-0.110030058979036,0.235369257943911,
-0.413846933692272));
#28346=CARTESIAN_POINT('Ctrl Pts',(-0.169239215181842,0.179564842036591,
-0.411206782050343));
#28347=CARTESIAN_POINT('Ctrl Pts',(-0.217721432531556,0.133870527261602,
-0.409044947395889));
#28348=CARTESIAN_POINT('Ctrl Pts',(-0.245876960799228,0.0666093509869193,
-0.406883112741436));
#28349=CARTESIAN_POINT('Ctrl Pts',(-0.24647636517194,-0.000206920082869883,
-0.404721278086982));
#28350=CARTESIAN_POINT('Origin',(0.,0.,-0.58));
#28351=CARTESIAN_POINT('',(-0.246620278596279,0.000155836006318556,-0.347578721913017));
#28352=CARTESIAN_POINT('',(-0.246589150649816,0.000170838254374723,-0.354721278086982));
#28353=CARTESIAN_POINT('',(-0.24635,-3.0169173896995E-17,-0.58));
#28354=CARTESIAN_POINT('Ctrl Pts',(-0.246620278596279,0.000155836006318556,
-0.347578721913017));
#28355=CARTESIAN_POINT('Ctrl Pts',(-0.246690378530408,0.00963297541655684,
-0.34788582018687));
#28356=CARTESIAN_POINT('Ctrl Pts',(-0.2461911898936,0.0191026624362393,
-0.348192918460724));
#28357=CARTESIAN_POINT('Ctrl Pts',(-0.245097962003322,0.028503266632493,
-0.348500016734578));
#28358=CARTESIAN_POINT('Ctrl Pts',(-0.235699382931871,0.10932111133222,
-0.351140168376506));
#28359=CARTESIAN_POINT('Ctrl Pts',(-0.182395383747831,0.185033047007441,
-0.353780320018435));
#28360=CARTESIAN_POINT('Ctrl Pts',(-0.109479809672547,0.221132581183705,
-0.356420471660364));
#28361=CARTESIAN_POINT('Ctrl Pts',(-0.0365642355972628,0.257232115359969,
-0.359060623302293));
#28362=CARTESIAN_POINT('Ctrl Pts',(0.0559629133692657,0.253719248037275,
-0.361700774944221));
#28363=CARTESIAN_POINT('Ctrl Pts',(0.125931438551998,0.21219500458571,-0.364340926586149));
#28364=CARTESIAN_POINT('Ctrl Pts',(0.195899963734732,0.170670761134143,
-0.366981078228078));
#28365=CARTESIAN_POINT('Ctrl Pts',(0.243309865133668,0.0911351415537013,
-0.369621229870007));
#28366=CARTESIAN_POINT('Ctrl Pts',(0.246553593143224,0.00983732153943592,
-0.372261381511935));
#28367=CARTESIAN_POINT('Ctrl Pts',(0.249797321152781,-0.0714604984748272,
-0.374901533153864));
#28368=CARTESIAN_POINT('Ctrl Pts',(0.208874875772961,-0.154520518922914,
-0.377541684795793));
#28369=CARTESIAN_POINT('Ctrl Pts',(0.142437081882846,-0.201487282208094,
-0.380181836437721));
#28370=CARTESIAN_POINT('Ctrl Pts',(0.0759992879927318,-0.248454045493275,
-0.38282198807965));
#28371=CARTESIAN_POINT('Ctrl Pts',(-0.0159538544076767,-0.259327551615548,
-0.385462139721579));
#28372=CARTESIAN_POINT('Ctrl Pts',(-0.091513756032631,-0.229152088455909,
-0.388102291363507));
#28373=CARTESIAN_POINT('Ctrl Pts',(-0.167073657657585,-0.19897662529627,
-0.390742443005436));
#28374=CARTESIAN_POINT('Ctrl Pts',(-0.226240318507085,-0.127752192854718,
-0.393382594647364));
#28375=CARTESIAN_POINT('Ctrl Pts',(-0.242047925078493,-0.047940057906735,
-0.396022746289293));
#28376=CARTESIAN_POINT('Ctrl Pts',(-0.245153333887077,-0.0322609412877993,
-0.396541404830534));
#28377=CARTESIAN_POINT('Ctrl Pts',(-0.246585399102055,-0.0162504019196318,
-0.397060063371776));
#28378=CARTESIAN_POINT('Ctrl Pts',(-0.246439321146211,-0.000213893874535243,
-0.397578721913017));
#28379=CARTESIAN_POINT('Ctrl Pts',(-0.24647636517194,-0.000206920082869883,
-0.404721278086982));
#28380=CARTESIAN_POINT('Ctrl Pts',(-0.246608986458792,-0.0149903622053166,
-0.404242961099507));
#28381=CARTESIAN_POINT('Ctrl Pts',(-0.245392629983733,-0.0297520245146864,
-0.403764644112032));
#28382=CARTESIAN_POINT('Ctrl Pts',(-0.242748991676294,-0.044253491287515,
-0.403286327124557));
#28383=CARTESIAN_POINT('Ctrl Pts',(-0.228156982191341,-0.124296793769336,
-0.400646175482628));
#28384=CARTESIAN_POINT('Ctrl Pts',(-0.170080333444842,-0.196412783798022,
-0.398006023840699));
#28385=CARTESIAN_POINT('Ctrl Pts',(-0.0949880747257705,-0.227733858068762,
-0.395365872198771));
#28386=CARTESIAN_POINT('Ctrl Pts',(-0.019895816006696,-0.259054932339504,
-0.392725720556842));
#28387=CARTESIAN_POINT('Ctrl Pts',(0.072212052684949,-0.249581090852299,
-0.390085568914914));
#28388=CARTESIAN_POINT('Ctrl Pts',(0.139356423966682,-0.203630134189933,
-0.387445417272985));
#28389=CARTESIAN_POINT('Ctrl Pts',(0.206500795248412,-0.157679177527568,
-0.384805265631057));
#28390=CARTESIAN_POINT('Ctrl Pts',(0.248681669120229,-0.0752511056900446,
-0.382165113989128));
#28391=CARTESIAN_POINT('Ctrl Pts',(0.246674678989956,0.00608664079719441,
-0.379524962347199));
#28392=CARTESIAN_POINT('Ctrl Pts',(0.244667688859683,0.0874243872844334,
-0.376884810705271));
#28393=CARTESIAN_POINT('Ctrl Pts',(0.19847283472732,0.167671808421389,-0.374244659063342));
#28394=CARTESIAN_POINT('Ctrl Pts',(0.1291438959245,0.210255317641276,-0.371604507421414));
#28395=CARTESIAN_POINT('Ctrl Pts',(0.0598149571216795,0.252838826861163,
-0.368964355779485));
#28396=CARTESIAN_POINT('Ctrl Pts',(-0.0326480663515998,0.257758424163981,
-0.366324204137556));
#28397=CARTESIAN_POINT('Ctrl Pts',(-0.106104201672608,0.222771952539835,
-0.363684052495628));
#28398=CARTESIAN_POINT('Ctrl Pts',(-0.179560336993617,0.187785480915688,
-0.361043900853699));
#28399=CARTESIAN_POINT('Ctrl Pts',(-0.234009584162354,0.112892940364575,
-0.358403749211771));
#28400=CARTESIAN_POINT('Ctrl Pts',(-0.244636139423289,0.0322273756154709,
-0.355763597569842));
#28401=CARTESIAN_POINT('Ctrl Pts',(-0.246034577478672,0.0216119134328442,
-0.355416157742222));
#28402=CARTESIAN_POINT('Ctrl Pts',(-0.246674087650934,0.0108964731602588,
-0.355068717914602));
#28403=CARTESIAN_POINT('Ctrl Pts',(-0.246589150649816,0.000170838254374723,
-0.354721278086982));
#28404=CARTESIAN_POINT('Origin',(0.,0.,-0.58));
#28405=CARTESIAN_POINT('',(-0.245982758627801,9.18475011218029E-5,-0.297578721913017));
#28406=CARTESIAN_POINT('',(-0.245970157583507,7.28788751880308E-5,-0.304721278086982));
#28407=CARTESIAN_POINT('',(-0.24635,-3.0169173896995E-17,-0.58));
#28408=CARTESIAN_POINT('Ctrl Pts',(-0.245982758627801,9.18475011218029E-5,
-0.297578721913017));
#28409=CARTESIAN_POINT('Ctrl Pts',(-0.246101246457855,0.0352839351195487,
-0.298711577001966));
#28410=CARTESIAN_POINT('Ctrl Pts',(-0.239047653887906,0.0704307209063493,
-0.299844432090914));
#28411=CARTESIAN_POINT('Ctrl Pts',(-0.224586866480519,0.102206587808051,
-0.300977287179863));
#28412=CARTESIAN_POINT('Ctrl Pts',(-0.190885582009419,0.176261167244235,
-0.303617438821791));
#28413=CARTESIAN_POINT('Ctrl Pts',(-0.116953115508088,0.232007054354664,
-0.30625759046372));
#28414=CARTESIAN_POINT('Ctrl Pts',(-0.0364849480944337,0.24403748840998,
-0.308897742105649));
#28415=CARTESIAN_POINT('Ctrl Pts',(0.0439832193192205,0.256067922465295,
-0.311537893747577));
#28416=CARTESIAN_POINT('Ctrl Pts',(0.130987087645194,0.224382903465497,
-0.314178045389506));
#28417=CARTESIAN_POINT('Ctrl Pts',(0.184873750101168,0.163423204320673,
-0.316818197031434));
#28418=CARTESIAN_POINT('Ctrl Pts',(0.238760412557142,0.102463505175849,
-0.319458348673363));
#28419=CARTESIAN_POINT('Ctrl Pts',(0.259529869143112,0.0122291258859946,
-0.322098500315292));
#28420=CARTESIAN_POINT('Ctrl Pts',(0.237716226654917,-0.0661546882076611,
-0.32473865195722));
#28421=CARTESIAN_POINT('Ctrl Pts',(0.215902584166721,-0.144538502301317,
-0.327378803599149));
#28422=CARTESIAN_POINT('Ctrl Pts',(0.151505842604362,-0.211071751198777,
-0.330018955241077));
#28423=CARTESIAN_POINT('Ctrl Pts',(0.0738754784841004,-0.235431223217419,
-0.332659106883006));
#28424=CARTESIAN_POINT('Ctrl Pts',(-0.00375488563616382,-0.259790695236061,
-0.335299258524935));
#28425=CARTESIAN_POINT('Ctrl Pts',(-0.0946188723143317,-0.241976390375881,
-0.337939410166864));
#28426=CARTESIAN_POINT('Ctrl Pts',(-0.157304286173984,-0.190107361083673,
-0.340579561808792));
#28427=CARTESIAN_POINT('Ctrl Pts',(-0.212698231586755,-0.144271655449523,
-0.342912615176867));
#28428=CARTESIAN_POINT('Ctrl Pts',(-0.246087723055121,-0.0718428494415446,
-0.345245668544942));
#28429=CARTESIAN_POINT('Ctrl Pts',(-0.246620278596279,0.000155836006318556,
-0.347578721913017));
#28430=CARTESIAN_POINT('Ctrl Pts',(-0.246589150649816,0.000170838254374723,
-0.354721278086982));
#28431=CARTESIAN_POINT('Ctrl Pts',(-0.246028662040124,-0.0706062802847878,
-0.352428566272674));
#28432=CARTESIAN_POINT('Ctrl Pts',(-0.21392201658485,-0.141827325604046,
-0.350135854458365));
#28433=CARTESIAN_POINT('Ctrl Pts',(-0.16017720978418,-0.187693116327548,
-0.347843142644056));
#28434=CARTESIAN_POINT('Ctrl Pts',(-0.0982878615310032,-0.240509454574367,
-0.345202991002127));
#28435=CARTESIAN_POINT('Ctrl Pts',(-0.00770530167151524,-0.259703542120912,
-0.342562839360199));
#28436=CARTESIAN_POINT('Ctrl Pts',(0.0702865375815846,-0.236527476386538,
-0.33992268771827));
#28437=CARTESIAN_POINT('Ctrl Pts',(0.148278376834687,-0.213351410652164,
-0.337282536076342));
#28438=CARTESIAN_POINT('Ctrl Pts',(0.213679495481401,-0.147805191636868,
-0.334642384434413));
#28439=CARTESIAN_POINT('Ctrl Pts',(0.236682661831279,-0.0697621820147013,
-0.332002232792484));
#28440=CARTESIAN_POINT('Ctrl Pts',(0.259685828181155,0.00828082760746218,
-0.329362081150556));
#28441=CARTESIAN_POINT('Ctrl Pts',(0.240291042234199,0.0988206278364971,
-0.326721929508627));
#28442=CARTESIAN_POINT('Ctrl Pts',(0.18733767692882,0.160592774600555,-0.324081777866698));
#28443=CARTESIAN_POINT('Ctrl Pts',(0.134384311623439,0.222364921364616,
-0.32144162622477));
#28444=CARTESIAN_POINT('Ctrl Pts',(0.0478723669596356,0.255369414663697,
-0.318801474582841));
#28445=CARTESIAN_POINT('Ctrl Pts',(-0.0327694495428521,0.24456411762082,
-0.316161322940913));
#28446=CARTESIAN_POINT('Ctrl Pts',(-0.113411266045338,0.233758820577943,
-0.313521171298984));
#28447=CARTESIAN_POINT('Ctrl Pts',(-0.188182954386505,0.179143733193108,
-0.310881019657055));
#28448=CARTESIAN_POINT('Ctrl Pts',(-0.223006549473582,0.105610242604011,
-0.308240868015127));
#28449=CARTESIAN_POINT('Ctrl Pts',(-0.238481010938067,0.0729343754620719,
-0.307067671372412));
#28450=CARTESIAN_POINT('Ctrl Pts',(-0.246067235702702,0.0365228395984935,
-0.305894474729697));
#28451=CARTESIAN_POINT('Ctrl Pts',(-0.245970157583507,7.28788751880308E-5,
-0.304721278086982));
#28452=CARTESIAN_POINT('Origin',(0.,0.,-0.58));
#28453=CARTESIAN_POINT('',(-0.246288309719265,-0.000221392196024267,-0.247578721913017));
#28454=CARTESIAN_POINT('',(-0.246325271707252,-0.000222610671457577,-0.254721278086982));
#28455=CARTESIAN_POINT('',(-0.24635,-3.0169173896995E-17,-0.58));
#28456=CARTESIAN_POINT('Ctrl Pts',(-0.246288309719265,-0.000221392196024267,
-0.247578721913017));
#28457=CARTESIAN_POINT('Ctrl Pts',(-0.245750103398489,0.0604324982965131,
-0.24953733381706));
#28458=CARTESIAN_POINT('Ctrl Pts',(-0.223113577325142,0.121445534342942,
-0.251495945721104));
#28459=CARTESIAN_POINT('Ctrl Pts',(-0.182486358855138,0.1660848458429,-0.253454557625148));
#28460=CARTESIAN_POINT('Ctrl Pts',(-0.127722054947289,0.226257333974859,
-0.256094709267076));
#28461=CARTESIAN_POINT('Ctrl Pts',(-0.0402682085204694,0.256678351015285,
-0.258734860909005));
#28462=CARTESIAN_POINT('Ctrl Pts',(0.0400171915015985,0.243483205932552,
-0.261375012550933));
#28463=CARTESIAN_POINT('Ctrl Pts',(0.12030259152367,0.230288060849818,-0.264015164192862));
#28464=CARTESIAN_POINT('Ctrl Pts',(0.193419545140986,0.173476753643925,
-0.266655315834791));
#28465=CARTESIAN_POINT('Ctrl Pts',(0.226044249609935,0.0989416211976409,
-0.269295467476719));
#28466=CARTESIAN_POINT('Ctrl Pts',(0.258668954078883,0.0244064887513605,
-0.271935619118648));
#28467=CARTESIAN_POINT('Ctrl Pts',(0.250801409399463,-0.0678524689353101,
-0.274575770760577));
#28468=CARTESIAN_POINT('Ctrl Pts',(0.206027329882984,-0.135787284118156,
-0.277215922402505));
#28469=CARTESIAN_POINT('Ctrl Pts',(0.161253250366504,-0.203722099301003,
-0.279856074044434));
#28470=CARTESIAN_POINT('Ctrl Pts',(0.0795726360129633,-0.247332771980028,
-0.282496225686362));
#28471=CARTESIAN_POINT('Ctrl Pts',(-0.00178773407926969,-0.246743290068368,
-0.285136377328291));
#28472=CARTESIAN_POINT('Ctrl Pts',(-0.0831481041715026,-0.246153808156707,
-0.28777652897022));
#28473=CARTESIAN_POINT('Ctrl Pts',(-0.164188230002428,-0.201364171654361,
-0.290416680612148));
#28474=CARTESIAN_POINT('Ctrl Pts',(-0.207973241697457,-0.132787717522219,
-0.293056832254077));
#28475=CARTESIAN_POINT('Ctrl Pts',(-0.232970668417953,-0.0936365372311268,
-0.294564128807057));
#28476=CARTESIAN_POINT('Ctrl Pts',(-0.245825107133315,-0.0467322457804416,
-0.296071425360037));
#28477=CARTESIAN_POINT('Ctrl Pts',(-0.245982758627801,9.18475011218029E-5,
-0.297578721913017));
#28478=CARTESIAN_POINT('Ctrl Pts',(-0.245970157583507,7.28788751880308E-5,
-0.304721278086982));
#28479=CARTESIAN_POINT('Ctrl Pts',(-0.245848771937587,-0.0455038387503123,
-0.303254323087769));
#28480=CARTESIAN_POINT('Ctrl Pts',(-0.233714706137793,-0.0911406328242931,
-0.301787368088555));
#28481=CARTESIAN_POINT('Ctrl Pts',(-0.209968597656244,-0.129609538419296,
-0.300320413089341));
#28482=CARTESIAN_POINT('Ctrl Pts',(-0.16723154891884,-0.198843935060144,
-0.297680261447412));
#28483=CARTESIAN_POINT('Ctrl Pts',(-0.0868819496110477,-0.244860834548482,
-0.295040109805483));
#28484=CARTESIAN_POINT('Ctrl Pts',(-0.00553995505069527,-0.246687562209828,
-0.292399958163555));
#28485=CARTESIAN_POINT('Ctrl Pts',(0.0758020395096583,-0.248514289871173,
-0.289759806521626));
#28486=CARTESIAN_POINT('Ctrl Pts',(0.158136429322571,-0.206150845705526,
-0.287119654879698));
#28487=CARTESIAN_POINT('Ctrl Pts',(0.203938470407728,-0.138904804592017,
-0.284479503237769));
#28488=CARTESIAN_POINT('Ctrl Pts',(0.249740511492885,-0.0716587634785091,
-0.281839351595841));
#28489=CARTESIAN_POINT('Ctrl Pts',(0.259010203850289,0.0204698745828584,
-0.279199199953912));
#28490=CARTESIAN_POINT('Ctrl Pts',(0.227522789960257,0.0954925363559746,
-0.276559048311983));
#28491=CARTESIAN_POINT('Ctrl Pts',(0.196035376070226,0.17051519812909,-0.273918896670055));
#28492=CARTESIAN_POINT('Ctrl Pts',(0.123790855932758,0.228431883613956,
-0.271278745028126));
#28493=CARTESIAN_POINT('Ctrl Pts',(0.0437154117701946,0.242846468421408,
-0.268638593386197));
#28494=CARTESIAN_POINT('Ctrl Pts',(-0.0363600323923712,0.257261053228861,
-0.265998441744269));
#28495=CARTESIAN_POINT('Ctrl Pts',(-0.124266400580035,0.228173537358901,
-0.26335829010234));
#28496=CARTESIAN_POINT('Ctrl Pts',(-0.17993946242722,0.168840854985951,
-0.260718138460411));
#28497=CARTESIAN_POINT('Ctrl Pts',(-0.22209153343667,0.123917954078675,
-0.258719185002602));
#28498=CARTESIAN_POINT('Ctrl Pts',(-0.245765710234638,0.0616568694570882,
-0.256720231544792));
#28499=CARTESIAN_POINT('Ctrl Pts',(-0.246325271707252,-0.000222610671457577,
-0.254721278086982));
#28500=CARTESIAN_POINT('Origin',(0.,0.,-0.58));
#28501=CARTESIAN_POINT('',(-0.246717581299304,8.00647905813846E-5,-0.197578721913017));
#28502=CARTESIAN_POINT('',(-0.246698535278583,0.000100771421362301,-0.204721278086982));
#28503=CARTESIAN_POINT('',(-0.24635,-3.0169173896995E-17,-0.58));
#28504=CARTESIAN_POINT('Ctrl Pts',(-0.246717581299304,8.00647905813846E-5,
-0.197578721913017));
#28505=CARTESIAN_POINT('Ctrl Pts',(-0.246736504680948,0.00452600816889543,
-0.197722938990227));
#28506=CARTESIAN_POINT('Ctrl Pts',(-0.246626683453427,0.00897099792437958,
-0.197867156067437));
#28507=CARTESIAN_POINT('Ctrl Pts',(-0.246385167424414,0.0134088205603487,
-0.198011373144647));
#28508=CARTESIAN_POINT('Ctrl Pts',(-0.241963784375424,0.0946511043842296,
-0.200651524786575));
#28509=CARTESIAN_POINT('Ctrl Pts',(-0.193406398690778,0.173491410284751,
-0.203291676428504));
#28510=CARTESIAN_POINT('Ctrl Pts',(-0.122843537789156,0.213997458887118,
-0.205931828070432));
#28511=CARTESIAN_POINT('Ctrl Pts',(-0.0522806768875334,0.254503507489485,
-0.208571979712361));
#28512=CARTESIAN_POINT('Ctrl Pts',(0.0402876592310675,0.2566752987937,-0.21121213135429));
#28513=CARTESIAN_POINT('Ctrl Pts',(0.112672500456431,0.219523016619024,
-0.213852282996218));
#28514=CARTESIAN_POINT('Ctrl Pts',(0.185057341681796,0.182370734444347,
-0.216492434638147));
#28515=CARTESIAN_POINT('Ctrl Pts',(0.237258688013924,0.105894378790777,
-0.219132586280076));
#28516=CARTESIAN_POINT('Ctrl Pts',(0.2454852395792,0.0249488343818461,-0.221772737922004));
#28517=CARTESIAN_POINT('Ctrl Pts',(0.253711791144477,-0.0559967100270831,
-0.224412889563933));
#28518=CARTESIAN_POINT('Ctrl Pts',(0.217963547942906,-0.141411443191371,
-0.227053041205861));
#28519=CARTESIAN_POINT('Ctrl Pts',(0.154533139065134,-0.192366722999149,
-0.22969319284779));
#28520=CARTESIAN_POINT('Ctrl Pts',(0.0911027301873629,-0.243322002806927,
-0.232333344489719));
#28521=CARTESIAN_POINT('Ctrl Pts',(-9.84436660830812E-6,-0.259817829258193,
-0.234973496131648));
#28522=CARTESIAN_POINT('Ctrl Pts',(-0.0772790927469542,-0.234336059988257,
-0.237613647773576));
#28523=CARTESIAN_POINT('Ctrl Pts',(-0.1545483411273,-0.208854290718321,
-0.240253799415505));
#28524=CARTESIAN_POINT('Ctrl Pts',(-0.217974263334022,-0.141394925727183,
-0.242893951057433));
#28525=CARTESIAN_POINT('Ctrl Pts',(-0.238649843742943,-0.0627032636198674,
-0.245534102699361));
#28526=CARTESIAN_POINT('Ctrl Pts',(-0.243987124158482,-0.042389470307912,
-0.246215642437246));
#28527=CARTESIAN_POINT('Ctrl Pts',(-0.246475589799629,-0.0213271745833612,
-0.246897182175132));
#28528=CARTESIAN_POINT('Ctrl Pts',(-0.246288309719265,-0.000221392196024267,
-0.247578721913017));
#28529=CARTESIAN_POINT('Ctrl Pts',(-0.246325271707252,-0.000222610671457577,
-0.254721278086982));
#28530=CARTESIAN_POINT('Ctrl Pts',(-0.246504760528635,-0.0200715021689657,
-0.254080079902863));
#28531=CARTESIAN_POINT('Ctrl Pts',(-0.244305953528097,-0.0398811298345366,
-0.253438881718744));
#28532=CARTESIAN_POINT('Ctrl Pts',(-0.239575819577798,-0.0590666667812709,
-0.252797683534626));
#28533=CARTESIAN_POINT('Ctrl Pts',(-0.220099359374485,-0.138063657299604,
-0.250157531892697));
#28534=CARTESIAN_POINT('Ctrl Pts',(-0.157706683461156,-0.206479789460333,
-0.247517380250768));
#28535=CARTESIAN_POINT('Ctrl Pts',(-0.080833894847107,-0.233133708190821,
-0.24487722860884));
#28536=CARTESIAN_POINT('Ctrl Pts',(-0.00396110623305791,-0.259787626921309,
-0.242237076966911));
#28537=CARTESIAN_POINT('Ctrl Pts',(0.0873917950817112,-0.244679332221555,
-0.239596925324982));
#28538=CARTESIAN_POINT('Ctrl Pts',(0.151589785853267,-0.194694584608596,
-0.236956773683054));
#28539=CARTESIAN_POINT('Ctrl Pts',(0.215787776624823,-0.144709836995635,
-0.234316622041125));
#28540=CARTESIAN_POINT('Ctrl Pts',(0.252830856853165,-0.0598486364694672,
-0.231676470399197));
#28541=CARTESIAN_POINT('Ctrl Pts',(0.24583626217839,0.0212126530485721,
-0.229036318757268));
#28542=CARTESIAN_POINT('Ctrl Pts',(0.238841667503615,0.10227394256661,-0.22639616711534));
#28543=CARTESIAN_POINT('Ctrl Pts',(0.187809397925725,0.17953532107652,-0.223756015473411));
#28544=CARTESIAN_POINT('Ctrl Pts',(0.115997934563216,0.217784121615343,
-0.221115863831482));
#28545=CARTESIAN_POINT('Ctrl Pts',(0.044186471200707,0.256032922154165,
-0.218475712189554));
#28546=CARTESIAN_POINT('Ctrl Pts',(-0.0484041859464199,0.255269144721901,
-0.215835560547625));
#28547=CARTESIAN_POINT('Ctrl Pts',(-0.119574893702499,0.215840888727965,
-0.213195408905696));
#28548=CARTESIAN_POINT('Ctrl Pts',(-0.190745601458579,0.176412632734028,
-0.210555257263768));
#28549=CARTESIAN_POINT('Ctrl Pts',(-0.240496359823611,0.098319898178419,
-0.207915105621839));
#28550=CARTESIAN_POINT('Ctrl Pts',(-0.246152749572341,0.0171542510864486,
-0.20527495397991));
#28551=CARTESIAN_POINT('Ctrl Pts',(-0.246548156992019,0.0114804024818092,
-0.205090395348934));
#28552=CARTESIAN_POINT('Ctrl Pts',(-0.246728090793561,0.00579153763806257,
-0.204905836717958));
#28553=CARTESIAN_POINT('Ctrl Pts',(-0.246698535278583,0.000100771421362301,
-0.204721278086982));
#28554=CARTESIAN_POINT('Origin',(0.,0.,-0.58));
#28555=CARTESIAN_POINT('',(-0.246061894210452,0.000159263489505596,-0.147578721913017));
#28556=CARTESIAN_POINT('',(-0.246038304346645,0.000144234873082875,-0.154721278086982));
#28557=CARTESIAN_POINT('',(-0.24635,-3.0169173896995E-17,-0.58));
#28558=CARTESIAN_POINT('Ctrl Pts',(-0.246061894210452,0.000159263489505596,
-0.147578721913017));
#28559=CARTESIAN_POINT('Ctrl Pts',(-0.246241265808746,0.0302671727973585,
-0.148548695805322));
#28560=CARTESIAN_POINT('Ctrl Pts',(-0.241124310761266,0.0603162330277041,
-0.149518669697626));
#28561=CARTESIAN_POINT('Ctrl Pts',(-0.230435621126537,0.0882319217573935,
-0.150488643589931));
#28562=CARTESIAN_POINT('Ctrl Pts',(-0.201342300457734,0.164215050808554,
-0.15312879523186));
#28563=CARTESIAN_POINT('Ctrl Pts',(-0.130970083701752,0.224392828920623,
-0.155768946873788));
#28564=CARTESIAN_POINT('Ctrl Pts',(-0.0513918344865268,0.24133861398937,
-0.158409098515717));
#28565=CARTESIAN_POINT('Ctrl Pts',(0.0281864147286988,0.258284399058117,
-0.161049250157646));
#28566=CARTESIAN_POINT('Ctrl Pts',(0.116970696403168,0.231998191083541,
-0.163689401799574));
#28567=CARTESIAN_POINT('Ctrl Pts',(0.174496663610151,0.174460200189865,
-0.166329553441503));
#28568=CARTESIAN_POINT('Ctrl Pts',(0.232022630817135,0.116922209296188,
-0.168969705083432));
#28569=CARTESIAN_POINT('Ctrl Pts',(0.25829028355663,0.0281324354834098,
-0.17160985672536));
#28570=CARTESIAN_POINT('Ctrl Pts',(0.241327868439501,-0.0514422701154425,
-0.174250008367289));
#28571=CARTESIAN_POINT('Ctrl Pts',(0.224365453322372,-0.131016975714293,
-0.176890160009218));
#28572=CARTESIAN_POINT('Ctrl Pts',(0.164172970348623,-0.201376613099217,
-0.179530311651146));
#28573=CARTESIAN_POINT('Ctrl Pts',(0.0881837624159238,-0.230454054503992,
-0.182170463293075));
#28574=CARTESIAN_POINT('Ctrl Pts',(0.012194554483225,-0.259531495908768,
-0.184810614935003));
#28575=CARTESIAN_POINT('Ctrl Pts',(-0.0795913784084228,-0.247326741333394,
-0.187450766576932));
#28576=CARTESIAN_POINT('Ctrl Pts',(-0.14534165464758,-0.199402233172087,
-0.19009091821886));
#28577=CARTESIAN_POINT('Ctrl Pts',(-0.207500352087109,-0.154095579373379,
-0.192586852783579));
#28578=CARTESIAN_POINT('Ctrl Pts',(-0.246390078320868,-0.0768649403738304,
-0.195082787348298));
#28579=CARTESIAN_POINT('Ctrl Pts',(-0.246717581299304,8.00647905813846E-5,
-0.197578721913017));
#28580=CARTESIAN_POINT('Ctrl Pts',(-0.246698535278583,0.000100771421362301,
-0.204721278086982));
#28581=CARTESIAN_POINT('Ctrl Pts',(-0.246305292677956,-0.0756161196000796,
-0.202265685076029));
#28582=CARTESIAN_POINT('Ctrl Pts',(-0.208826396508379,-0.151669608495989,
-0.199810092065077));
#28583=CARTESIAN_POINT('Ctrl Pts',(-0.148357316731195,-0.197168838869184,
-0.197354499054125));
#28584=CARTESIAN_POINT('Ctrl Pts',(-0.0833434730088882,-0.246087722104518,
-0.194714347412196));
#28585=CARTESIAN_POINT('Ctrl Pts',(0.00824623556815356,-0.259686928946854,
-0.192074195770267));
#28586=CARTESIAN_POINT('Ctrl Pts',(0.0846688584477465,-0.231768481161568,
-0.189434044128339));
#28587=CARTESIAN_POINT('Ctrl Pts',(0.161091481327338,-0.203850033376283,
-0.18679389248641));
#28588=CARTESIAN_POINT('Ctrl Pts',(0.222347018509481,-0.134413930963373,
-0.184153740844482));
#28589=CARTESIAN_POINT('Ctrl Pts',(0.240517629577363,-0.0551063909376154,
-0.181513589202553));
#28590=CARTESIAN_POINT('Ctrl Pts',(0.258688240645247,0.024201149088146,
-0.178873437560624));
#28591=CARTESIAN_POINT('Ctrl Pts',(0.233773925598868,0.113380126726757,
-0.176233285918696));
#28592=CARTESIAN_POINT('Ctrl Pts',(0.177129639592286,0.171786306822376,
-0.173593134276767));
#28593=CARTESIAN_POINT('Ctrl Pts',(0.120485353585707,0.230192486917993,
-0.170952982634838));
#28594=CARTESIAN_POINT('Ctrl Pts',(0.0321110966189257,0.257825869470619,
-0.16831283099291));
#28595=CARTESIAN_POINT('Ctrl Pts',(-0.0477156560646856,0.242092256426266,
-0.165672679350981));
#28596=CARTESIAN_POINT('Ctrl Pts',(-0.127542408748298,0.226358643381913,
-0.163032527709053));
#28597=CARTESIAN_POINT('Ctrl Pts',(-0.19882165714874,0.16725803474058,-0.160392376067124));
#28598=CARTESIAN_POINT('Ctrl Pts',(-0.2290671510981,0.0917261401792469,
-0.157752224425195));
#28599=CARTESIAN_POINT('Ctrl Pts',(-0.240641292986694,0.0628221035571004,
-0.156741908979124));
#28600=CARTESIAN_POINT('Ctrl Pts',(-0.246206500009256,0.0315118887000048,
-0.155731593533053));
#28601=CARTESIAN_POINT('Ctrl Pts',(-0.246038304346645,0.000144234873082875,
-0.154721278086982));
#28602=CARTESIAN_POINT('Origin',(0.,0.,-0.58));
#28603=CARTESIAN_POINT('',(-0.246149652364137,-0.000196946980918933,-0.0975787219130166));
#28604=CARTESIAN_POINT('',(-0.246181916821291,-0.000205804393626753,-0.104721278086982));
#28605=CARTESIAN_POINT('',(-0.24635,-3.0169173896995E-17,-0.58));
#28606=CARTESIAN_POINT('Ctrl Pts',(-0.246149652364137,-0.000196946980918933,
-0.0975787219130166));
#28607=CARTESIAN_POINT('Ctrl Pts',(-0.245729114976462,0.0554922919781312,
-0.0993744526204165));
#28608=CARTESIAN_POINT('Ctrl Pts',(-0.227001298186543,0.111437622002477,
-0.101170183327816));
#28609=CARTESIAN_POINT('Ctrl Pts',(-0.192334463664016,0.154573316616123,
-0.102965914035216));
#28610=CARTESIAN_POINT('Ctrl Pts',(-0.141365963928531,0.217993056831428,
-0.105606065677145));
#28611=CARTESIAN_POINT('Ctrl Pts',(-0.0559436839388203,0.253723489525969,
-0.108246217319073));
#28612=CARTESIAN_POINT('Ctrl Pts',(0.0250001579011069,0.245480031317822,
-0.110886368961002));
#28613=CARTESIAN_POINT('Ctrl Pts',(0.105943999741037,0.237236573109673,
-0.11352652060293));
#28614=CARTESIAN_POINT('Ctrl Pts',(0.182409403431186,0.185019223998827,
-0.116166672244859));
#28615=CARTESIAN_POINT('Ctrl Pts',(0.219546547681062,0.112626614966495,
-0.118806823886788));
#28616=CARTESIAN_POINT('Ctrl Pts',(0.256683691930939,0.0402340059341607,
-0.121446975528716));
#28617=CARTESIAN_POINT('Ctrl Pts',(0.254492576740548,-0.0523338630196622,
-0.124087127170645));
#28618=CARTESIAN_POINT('Ctrl Pts',(0.213971787489004,-0.122888254505354,
-0.126727278812574));
#28619=CARTESIAN_POINT('Ctrl Pts',(0.173450998237462,-0.193442645991044,
-0.129367430454502));
#28620=CARTESIAN_POINT('Ctrl Pts',(0.0946005349247738,-0.241983560008603,
-0.132007582096431));
#28621=CARTESIAN_POINT('Ctrl Pts',(0.0133573261733158,-0.246387965892067,
-0.13464773373836));
#28622=CARTESIAN_POINT('Ctrl Pts',(-0.0678858825781422,-0.250792371775532,
-0.137287885380288));
#28623=CARTESIAN_POINT('Ctrl Pts',(-0.151521836768367,-0.211060269524901,
-0.139928037022217));
#28624=CARTESIAN_POINT('Ctrl Pts',(-0.199432601572667,-0.14529997840446,
-0.142568188664145));
#28625=CARTESIAN_POINT('Ctrl Pts',(-0.229741274784008,-0.103699574361793,
-0.144238366413769));
#28626=CARTESIAN_POINT('Ctrl Pts',(-0.245753038008484,-0.0516829155759291,
-0.145908544163393));
#28627=CARTESIAN_POINT('Ctrl Pts',(-0.246061894210452,0.000159263489505596,
-0.147578721913017));
#28628=CARTESIAN_POINT('Ctrl Pts',(-0.246038304346645,0.000144234873082875,
-0.154721278086982));
#28629=CARTESIAN_POINT('Ctrl Pts',(-0.245766971883129,-0.0504579189245854,
-0.153091441891125));
#28630=CARTESIAN_POINT('Ctrl Pts',(-0.230575036347777,-0.101209551856495,
-0.151461605695267));
#28631=CARTESIAN_POINT('Ctrl Pts',(-0.201619231011091,-0.142250237299355,
-0.149831769499409));
#28632=CARTESIAN_POINT('Ctrl Pts',(-0.154714077476446,-0.208731539735291,
-0.147191617857481));
#28633=CARTESIAN_POINT('Ctrl Pts',(-0.0716920309088846,-0.24973096412583,
-0.144551466215552));
#28634=CARTESIAN_POINT('Ctrl Pts',(0.00960875972723208,-0.246562601087141,
-0.141911314573624));
#28635=CARTESIAN_POINT('Ctrl Pts',(0.0909095503633488,-0.243394238048452,
-0.139271162931695));
#28636=CARTESIAN_POINT('Ctrl Pts',(0.170489085068021,-0.19605808758053,
-0.136631011289766));
#28637=CARTESIAN_POINT('Ctrl Pts',(0.21207817024949,-0.126128087551106,
-0.133990859647838));
#28638=CARTESIAN_POINT('Ctrl Pts',(0.253667255430958,-0.0561980875216845,
-0.131350708005909));
#28639=CARTESIAN_POINT('Ctrl Pts',(0.25726589108923,0.0363257620692371,
-0.128710556363981));
#28640=CARTESIAN_POINT('Ctrl Pts',(0.221233967996605,0.109274768183429,
-0.126070404722052));
#28641=CARTESIAN_POINT('Ctrl Pts',(0.185202044903979,0.182223774297623,
-0.123430253080123));
#28642=CARTESIAN_POINT('Ctrl Pts',(0.109539563060456,0.235597936935084,
-0.120790101438195));
#28643=CARTESIAN_POINT('Ctrl Pts',(0.0287304645584095,0.24507142952619,
-0.118149949796266));
#28644=CARTESIAN_POINT('Ctrl Pts',(-0.052078633943639,0.254544922117296,
-0.115509798154338));
#28645=CARTESIAN_POINT('Ctrl Pts',(-0.138034349104214,0.220117744662039,
-0.112869646512409));
#28646=CARTESIAN_POINT('Ctrl Pts',(-0.189961459263067,0.157480443860448,
-0.11022949487048));
#28647=CARTESIAN_POINT('Ctrl Pts',(-0.226073751091705,0.113919835943204,
-0.108393422609314));
#28648=CARTESIAN_POINT('Ctrl Pts',(-0.245728464227458,0.0567156970941223,
-0.106557350348148));
#28649=CARTESIAN_POINT('Ctrl Pts',(-0.246181916821291,-0.000205804393626753,
-0.104721278086982));
#28650=CARTESIAN_POINT('Origin',(0.,0.,-0.58));
#28651=CARTESIAN_POINT('',(-0.246745528500925,-8.72836701185098E-6,-0.0475787219130168));
#28652=CARTESIAN_POINT('',(-0.246748421001242,1.25335797698571E-5,-0.0547212780869822));
#28653=CARTESIAN_POINT('',(-0.24635,-3.0169173896995E-17,-0.58));
#28654=CARTESIAN_POINT('Ctrl Pts',(-0.246745528500925,-8.72836701185098E-6,
-0.0475787219130168));
#28655=CARTESIAN_POINT('Ctrl Pts',(-0.246691462824838,0.080780672528638,
-0.0502002094355115));
#28656=CARTESIAN_POINT('Ctrl Pts',(-0.203208326166415,0.161612112961239,
-0.0528216969580061));
#28657=CARTESIAN_POINT('Ctrl Pts',(-0.135746111999613,0.206054714378708,
-0.0554431844805008));
#28658=CARTESIAN_POINT('Ctrl Pts',(-0.0678035893012281,0.250813732339722,
-0.0580833361224295));
#28659=CARTESIAN_POINT('Ctrl Pts',(0.0244606725130793,0.258663913880818,
-0.0607234877643582));
#28660=CARTESIAN_POINT('Ctrl Pts',(0.0989898525822783,0.226024087587752,
-0.0633636394062869));
#28661=CARTESIAN_POINT('Ctrl Pts',(0.173519032651475,0.193384261294688,
-0.0660037910482156));
#28662=CARTESIAN_POINT('Ctrl Pts',(0.230313130975565,0.120254427167465,
-0.0686439426901442));
#28663=CARTESIAN_POINT('Ctrl Pts',(0.243491040779466,0.039966032231016,
-0.0712840943320728));
#28664=CARTESIAN_POINT('Ctrl Pts',(0.256668950583366,-0.0403223627054333,
-0.0739242459740013));
#28665=CARTESIAN_POINT('Ctrl Pts',(0.226230671867078,-0.127769318451109,
-0.0765643976159299));
#28666=CARTESIAN_POINT('Ctrl Pts',(0.166046980319095,-0.182520920142066,
-0.0792045492578585));
#28667=CARTESIAN_POINT('Ctrl Pts',(0.105863288771112,-0.237272521833022,
-0.0818447008997871));
#28668=CARTESIAN_POINT('Ctrl Pts',(0.0159341843914353,-0.25932876946926,
-0.0844848525417159));
#28669=CARTESIAN_POINT('Ctrl Pts',(-0.0627532815273662,-0.238636810281684,
-0.0871250041836445));
#28670=CARTESIAN_POINT('Ctrl Pts',(-0.141440747446168,-0.217944851094108,
-0.089765155825573));
#28671=CARTESIAN_POINT('Ctrl Pts',(-0.208886574904093,-0.15450468508272,
-0.0924053074675015));
#28672=CARTESIAN_POINT('Ctrl Pts',(-0.234352128892428,-0.0772300782089907,
-0.0950454591094301));
#28673=CARTESIAN_POINT('Ctrl Pts',(-0.242496981845425,-0.0525147191684789,
-0.0958898800439589));
#28674=CARTESIAN_POINT('Ctrl Pts',(-0.24634740505191,-0.0263841469943832,
-0.0967343009784877));
#28675=CARTESIAN_POINT('Ctrl Pts',(-0.246149652364137,-0.000196946980918933,
-0.0975787219130166));
#28676=CARTESIAN_POINT('Ctrl Pts',(-0.246181916821291,-0.000205804393626753,
-0.104721278086982));
#28677=CARTESIAN_POINT('Ctrl Pts',(-0.246380499354541,-0.0251336934731506,
-0.103917198706219));
#28678=CARTESIAN_POINT('Ctrl Pts',(-0.242896536971094,-0.0500073764876101,
-0.103113119325457));
#28679=CARTESIAN_POINT('Ctrl Pts',(-0.235499587892452,-0.0736571948666213,
-0.102309039944694));
#28680=CARTESIAN_POINT('Ctrl Pts',(-0.211212101205851,-0.151310108644177,
-0.0996688883027656));
#28681=CARTESIAN_POINT('Ctrl Pts',(-0.144738622675513,-0.215768512051366,
-0.0970287366608371));
#28682=CARTESIAN_POINT('Ctrl Pts',(-0.0663750455930597,-0.237654800632327,
-0.0943885850189085));
#28683=CARTESIAN_POINT('Ctrl Pts',(0.0119885314893938,-0.259541089213289,
-0.0917484333769799));
#28684=CARTESIAN_POINT('Ctrl Pts',(0.102242207123963,-0.238855262968024,
-0.0891082817350513));
#28685=CARTESIAN_POINT('Ctrl Pts',(0.163251794345776,-0.185025147060926,
-0.0864681300931226));
#28686=CARTESIAN_POINT('Ctrl Pts',(0.224261381567592,-0.131195031153826,
-0.0838279784511939));
#28687=CARTESIAN_POINT('Ctrl Pts',(0.256026880376651,-0.0442206255848928,
-0.0811878268092653));
#28688=CARTESIAN_POINT('Ctrl Pts',(0.244071117874901,0.0362586807743849,
-0.0785476751673366));
#28689=CARTESIAN_POINT('Ctrl Pts',(0.232115355373152,0.11673798713366,-0.0759075235254081));
#28690=CARTESIAN_POINT('Ctrl Pts',(0.176438331560597,0.19072219428328,-0.0732673718834795));
#28691=CARTESIAN_POINT('Ctrl Pts',(0.102414890955883,0.224492068861293,
-0.0706272202415508));
#28692=CARTESIAN_POINT('Ctrl Pts',(0.0283914503511699,0.258261943439305,
-0.0679870685996222));
#28693=CARTESIAN_POINT('Ctrl Pts',(-0.0639784070457014,0.251817485445711,
-0.0653469169576935));
#28694=CARTESIAN_POINT('Ctrl Pts',(-0.132595160836082,0.208096147537468,
-0.0627067653157649));
#28695=CARTESIAN_POINT('Ctrl Pts',(-0.201211914626462,0.164374809629225,
-0.0600666136738363));
#28696=CARTESIAN_POINT('Ctrl Pts',(-0.24607556481035,0.0833765918063334,
-0.0574264620319078));
#28697=CARTESIAN_POINT('Ctrl Pts',(-0.246740958917921,0.00201664698560347,
-0.0547863103899792));
#28698=CARTESIAN_POINT('Ctrl Pts',(-0.246746422254512,0.00134862669725098,
-0.0547646329556469));
#28699=CARTESIAN_POINT('Ctrl Pts',(-0.246748905955546,0.000680582022990077,
-0.0547429555213145));
#28700=CARTESIAN_POINT('Ctrl Pts',(-0.246748421001242,1.25335797698571E-5,
-0.0547212780869822));
#28701=CARTESIAN_POINT('Origin',(0.,0.,-0.58));
#28702=CARTESIAN_POINT('',(-0.24635,-3.0169173896995E-17,0.));
#28703=CARTESIAN_POINT('',(-0.246160120813712,0.000192360259597545,-0.00472127808698222));
#28704=CARTESIAN_POINT('',(-0.24635,-3.0169173896995E-17,-0.58));
#28705=CARTESIAN_POINT('',(-0.235034375322676,0.0738049111962042,0.));
#28706=CARTESIAN_POINT('Origin',(0.,0.,0.));
#28707=CARTESIAN_POINT('Ctrl Pts',(-0.235034375322676,0.0738049111962042,
0.));
#28708=CARTESIAN_POINT('Ctrl Pts',(-0.21054802840921,0.151782557364509,
-0.0026401516419286));
#28709=CARTESIAN_POINT('Ctrl Pts',(-0.144434507356266,0.21595452844779,
-0.00528030328385723));
#28710=CARTESIAN_POINT('Ctrl Pts',(-0.0661699330088478,0.237693665813309,
-0.00792045492578582));
#28711=CARTESIAN_POINT('Ctrl Pts',(0.0120946413385708,0.259432803178828,
-0.0105606065677144));
#28712=CARTESIAN_POINT('Ctrl Pts',(0.102510268980464,0.238739106826586,
-0.0132007582096429));
#28713=CARTESIAN_POINT('Ctrl Pts',(0.163505372344248,0.184863010201967,
-0.0158409098515715));
#28714=CARTESIAN_POINT('Ctrl Pts',(0.224500475708032,0.130986913577347,
-0.0184810614935001));
#28715=CARTESIAN_POINT('Ctrl Pts',(0.256075054793706,0.0439284166803513,
-0.0211212131354288));
#28716=CARTESIAN_POINT('Ctrl Pts',(0.244005633311165,-0.0365487101329756,
-0.0237613647773574));
#28717=CARTESIAN_POINT('Ctrl Pts',(0.231936211828623,-0.117025836946305,
-0.0264015164192861));
#28718=CARTESIAN_POINT('Ctrl Pts',(0.176222789777864,-0.190921593675964,
-0.0290416680612148));
#28719=CARTESIAN_POINT('Ctrl Pts',(0.10217255517054,-0.224601453711439,
-0.0316818197031434));
#28720=CARTESIAN_POINT('Ctrl Pts',(0.0281223205632187,-0.258281313746913,
-0.034321971345072));
#28721=CARTESIAN_POINT('Ctrl Pts',(-0.064264726600667,-0.251745277088204,
-0.0369621229870006));
#28722=CARTESIAN_POINT('Ctrl Pts',(-0.132837988199004,-0.207949054077961,
-0.0396022746289292));
#28723=CARTESIAN_POINT('Ctrl Pts',(-0.201411249797341,-0.164152831067718,
-0.0422424262708578));
#28724=CARTESIAN_POINT('Ctrl Pts',(-0.246170725830129,-0.0830964217059404,
-0.0448825779127865));
#28725=CARTESIAN_POINT('Ctrl Pts',(-0.246740072055293,-0.001734289834587,
-0.0475227295547151));
#28726=CARTESIAN_POINT('Ctrl Pts',(-0.246744096955142,-0.00115911357481157,
-0.047541393674149));
#28727=CARTESIAN_POINT('Ctrl Pts',(-0.24674591343056,-0.000583922036396745,
-0.0475600577935829));
#28728=CARTESIAN_POINT('Ctrl Pts',(-0.246745528500925,-8.72836701185098E-6,
-0.0475787219130168));
#28729=CARTESIAN_POINT('Ctrl Pts',(-0.246748421001242,1.25335797698571E-5,
-0.0547212780869822));
#28730=CARTESIAN_POINT('Ctrl Pts',(-0.246689842097585,-0.0806827918530022,
-0.0521028038793859));
#28731=CARTESIAN_POINT('Ctrl Pts',(-0.203316033568085,-0.16143310963746,
-0.0494843296717896));
#28732=CARTESIAN_POINT('Ctrl Pts',(-0.135979279895863,-0.205901704836232,
-0.0468658554641934));
#28733=CARTESIAN_POINT('Ctrl Pts',(-0.0680850687349815,-0.25073844001877,
-0.0442257038222647));
#28734=CARTESIAN_POINT('Ctrl Pts',(0.0241704916180333,-0.258690238565275,
-0.041585552180336));
#28735=CARTESIAN_POINT('Ctrl Pts',(0.0987340617504916,-0.226135213676908,
-0.0389454005384073));
#28736=CARTESIAN_POINT('Ctrl Pts',(0.173297631882948,-0.193580188788542,
-0.0363052488964788));
#28737=CARTESIAN_POINT('Ctrl Pts',(0.230169211794848,-0.120518340465306,
-0.0336650972545502));
#28738=CARTESIAN_POINT('Ctrl Pts',(0.243442143508976,-0.0402441251670753,
-0.0310249456126216));
#28739=CARTESIAN_POINT('Ctrl Pts',(0.256715075223104,0.0400300901311557,
-0.028384793970693));
#28740=CARTESIAN_POINT('Ctrl Pts',(0.226389358739459,0.127516672404382,
-0.0257446423287643));
#28741=CARTESIAN_POINT('Ctrl Pts',(0.166261259011876,0.182334672033693,
-0.0231044906868356));
#28742=CARTESIAN_POINT('Ctrl Pts',(0.106133159284294,0.237152671663005,
-0.020464339044907));
#28743=CARTESIAN_POINT('Ctrl Pts',(0.0162026763127736,0.259302088648401,
-0.0178241874029785));
#28744=CARTESIAN_POINT('Ctrl Pts',(-0.0624958806646685,0.238703388389264,
-0.0151840357610499));
#28745=CARTESIAN_POINT('Ctrl Pts',(-0.141194437642113,0.218104688130128,
-0.0125438841191213));
#28746=CARTESIAN_POINT('Ctrl Pts',(-0.208661068625478,0.154757870626456,
-0.00990373247719252));
#28747=CARTESIAN_POINT('Ctrl Pts',(-0.234238261452687,0.0775047438993852,
-0.00726358083526382));
#28748=CARTESIAN_POINT('Ctrl Pts',(-0.242448013067616,0.052708082819708,
-0.00641614658583661));
#28749=CARTESIAN_POINT('Ctrl Pts',(-0.246341989476513,0.0264786857761341,
-0.00556871233640941));
#28750=CARTESIAN_POINT('Ctrl Pts',(-0.246160120813712,0.000192360259597545,
-0.00472127808698222));
#28751=CARTESIAN_POINT('Origin',(0.,0.,-1.25608093797092));
#28752=CARTESIAN_POINT('',(-0.218124649763706,-7.71593311516547E-6,-0.0310809379709236));
#28753=CARTESIAN_POINT('',(-0.217607145566089,0.000170047718830516,-0.0212190620290759));
#28754=CARTESIAN_POINT('',(-0.217775,1.66341393608259E-15,-1.25608093797092));
#28755=CARTESIAN_POINT('',(0.157411390703589,0.150985252349406,2.08166817117217E-17));
#28756=CARTESIAN_POINT('Ctrl Pts',(-0.218124649763706,-7.71593311514433E-6,
-0.0310809379709236));
#28757=CARTESIAN_POINT('Ctrl Pts',(-0.218124990044004,-0.0005161908726374,
-0.0310622738514896));
#28758=CARTESIAN_POINT('Ctrl Pts',(-0.21789623761169,-0.0729512274990299,
-0.0284034580901269));
#28759=CARTESIAN_POINT('Ctrl Pts',(-0.138481185433633,-0.216766561130641,
-0.0231044906868355));
#28760=CARTESIAN_POINT('Ctrl Pts',(0.106531063757949,-0.234100257700769,
-0.0151840357610497));
#28761=CARTESIAN_POINT('Ctrl Pts',(0.250199565624991,-0.0435448713522292,
-0.0074825388654379));
#28762=CARTESIAN_POINT('Ctrl Pts',(0.202824236587796,0.103068069205317,
-0.00242119361175455));
#28763=CARTESIAN_POINT('Ctrl Pts',(0.157411390703589,0.150985252349406,
2.64816380629584E-17));
#28764=CARTESIAN_POINT('',(0.193653104151514,-0.0996214127458699,0.));
#28765=CARTESIAN_POINT('Origin',(0.,0.,0.));
#28766=CARTESIAN_POINT('Ctrl Pts',(-0.217607145566089,0.000170047718830547,
-0.0212190620290759));
#28767=CARTESIAN_POINT('Ctrl Pts',(-0.21726703576361,-0.0489876072703885,
-0.0194263446365745));
#28768=CARTESIAN_POINT('Ctrl Pts',(-0.176554978527624,-0.171097090088319,
-0.0149934756021445));
#28769=CARTESIAN_POINT('Ctrl Pts',(0.0261231005236458,-0.255800095598605,
-0.00792045492578602));
#28770=CARTESIAN_POINT('Ctrl Pts',(0.160601584503721,-0.163869943260562,
-0.0026401516419286));
#28771=CARTESIAN_POINT('Ctrl Pts',(0.193653104151514,-0.0996214127458699,
0.));
#28772=CARTESIAN_POINT('Origin',(0.,0.,-1.25608093797092));
#28773=CARTESIAN_POINT('',(-0.217597891388674,-0.00017410241024964,-0.0810809379709236));
#28774=CARTESIAN_POINT('',(-0.218127206752773,1.10797659262985E-5,-0.071219062029076));
#28775=CARTESIAN_POINT('',(-0.217775,1.66341393608259E-15,-1.25608093797092));
#28776=CARTESIAN_POINT('Ctrl Pts',(-0.217597891388674,-0.000174102410249656,
-0.0810809379709236));
#28777=CARTESIAN_POINT('Ctrl Pts',(-0.217772706049037,-0.023323757303425,
-0.0802365170363945));
#28778=CARTESIAN_POINT('Ctrl Pts',(-0.203726648457932,-0.118646141873473,
-0.0767519444599368));
#28779=CARTESIAN_POINT('Ctrl Pts',(-0.0654119898536204,-0.248746182667544,
-0.0706272202415509));
#28780=CARTESIAN_POINT('Ctrl Pts',(0.173081747182517,-0.190252584181875,
-0.0627067653157647));
#28781=CARTESIAN_POINT('Ctrl Pts',(0.253804655411944,0.0416584463135328,
-0.0547863103899791));
#28782=CARTESIAN_POINT('Ctrl Pts',(0.103185600053364,0.235600191315231,
-0.0468658554641932));
#28783=CARTESIAN_POINT('Ctrl Pts',(-0.140924429342837,0.214830415357785,
-0.0389640646578413));
#28784=CARTESIAN_POINT('Ctrl Pts',(-0.218076855354893,0.0714106391716104,
-0.0337024254934182));
#28785=CARTESIAN_POINT('Ctrl Pts',(-0.218124649763706,-7.71593311514433E-6,
-0.0310809379709236));
#28786=CARTESIAN_POINT('Ctrl Pts',(-0.218127206752773,1.10797659263097E-5,
-0.071219062029076));
#28787=CARTESIAN_POINT('Ctrl Pts',(-0.218075422621483,-0.0713241120186178,
-0.0686005878214797));
#28788=CARTESIAN_POINT('Ctrl Pts',(-0.141072539660443,-0.214682684397483,
-0.0633419619719547));
#28789=CARTESIAN_POINT('Ctrl Pts',(0.102921386109171,-0.235713292600032,
-0.055443184480501));
#28790=CARTESIAN_POINT('Ctrl Pts',(0.253745924148315,-0.0419518472751756,
-0.0475227295547153));
#28791=CARTESIAN_POINT('Ctrl Pts',(0.173321533153074,0.190064273543398,
-0.0396022746289292));
#28792=CARTESIAN_POINT('Ctrl Pts',(-0.0651758599354944,0.248804958958394,
-0.0316818197031436));
#28793=CARTESIAN_POINT('Ctrl Pts',(-0.203601252094894,0.118832438807541,
-0.025554082169859));
#28794=CARTESIAN_POINT('Ctrl Pts',(-0.21776791864521,0.0234073302005182,
-0.0220664962785031));
#28795=CARTESIAN_POINT('Ctrl Pts',(-0.217607145566089,0.000170047718830547,
-0.0212190620290759));
#28796=CARTESIAN_POINT('Origin',(0.,0.,-1.25608093797092));
#28797=CARTESIAN_POINT('',(-0.217520312610843,0.000140789959117709,-0.131080937970923));
#28798=CARTESIAN_POINT('',(-0.21762641337835,-0.000181932420623115,-0.121219062029076));
#28799=CARTESIAN_POINT('',(-0.217775,1.66341393608259E-15,-1.25608093797092));
#28800=CARTESIAN_POINT('Ctrl Pts',(-0.217520312610843,0.000140789959117728,
-0.131080937970923));
#28801=CARTESIAN_POINT('Ctrl Pts',(-0.217247281722338,-0.0456880330405798,
-0.129410760221299));
#28802=CARTESIAN_POINT('Ctrl Pts',(-0.180717894981605,-0.164359326083748,
-0.125100430829747));
#28803=CARTESIAN_POINT('Ctrl Pts',(0.0139231655990339,-0.256825521944582,
-0.118149949796266));
#28804=CARTESIAN_POINT('Ctrl Pts',(0.223036130664036,-0.128094072175867,
-0.11022949487048));
#28805=CARTESIAN_POINT('Ctrl Pts',(0.228847010841678,0.117397719925839,
-0.102309039944694));
#28806=CARTESIAN_POINT('Ctrl Pts',(0.0260592703673014,0.255879147195341,
-0.0943885850189083));
#28807=CARTESIAN_POINT('Ctrl Pts',(-0.176330078465526,0.171223727000115,
-0.0873125510276516));
#28808=CARTESIAN_POINT('Ctrl Pts',(-0.217226133606649,0.0490555465213744,
-0.0828766686783232));
#28809=CARTESIAN_POINT('Ctrl Pts',(-0.217597891388674,-0.000174102410249656,
-0.0810809379709236));
#28810=CARTESIAN_POINT('Ctrl Pts',(-0.21762641337835,-0.000181932420623089,
-0.121219062029076));
#28811=CARTESIAN_POINT('Ctrl Pts',(-0.217801961627503,-0.0222183482691874,
-0.120414982648313));
#28812=CARTESIAN_POINT('Ctrl Pts',(-0.204609608685256,-0.116404900586581,
-0.116970751625622));
#28813=CARTESIAN_POINT('Ctrl Pts',(-0.0691868957427056,-0.24772241328998,
-0.110886368961002));
#28814=CARTESIAN_POINT('Ctrl Pts',(0.170167610585507,-0.192863199035107,
-0.102965914035216));
#28815=CARTESIAN_POINT('Ctrl Pts',(0.254410332361144,0.0377946191841849,
-0.0950454591094304));
#28816=CARTESIAN_POINT('Ctrl Pts',(0.106753780372761,0.234002178088288,
-0.0871250041836445));
#28817=CARTESIAN_POINT('Ctrl Pts',(-0.138212881221763,0.216911349922406,
-0.0792045492578586));
#28818=CARTESIAN_POINT('Ctrl Pts',(-0.217858031003544,0.0731175399198877,
-0.0739025685396692));
#28819=CARTESIAN_POINT('Ctrl Pts',(-0.218127635455527,0.000601638928588284,
-0.0712407394634083));
#28820=CARTESIAN_POINT('Ctrl Pts',(-0.218127206752773,1.10797659263097E-5,
-0.071219062029076));
#28821=CARTESIAN_POINT('Origin',(0.,0.,-1.25608093797092));
#28822=CARTESIAN_POINT('',(-0.218099944255961,7.07777948932365E-5,-0.181080937970924));
#28823=CARTESIAN_POINT('',(-0.217499459018025,0.000127504564585532,-0.171219062029076));
#28824=CARTESIAN_POINT('',(-0.217775,1.66341393608259E-15,-1.25608093797092));
#28825=CARTESIAN_POINT('Ctrl Pts',(-0.218099944255961,7.07777948932352E-5,
-0.181080937970924));
#28826=CARTESIAN_POINT('Ctrl Pts',(-0.217810429495954,-0.0679491065147507,
-0.178585003406205));
#28827=CARTESIAN_POINT('Ctrl Pts',(-0.147066455741474,-0.20843871206212,
-0.173448917199557));
#28828=CARTESIAN_POINT('Ctrl Pts',(0.0919194261743976,-0.240216610307221,
-0.165672679350981));
#28829=CARTESIAN_POINT('Ctrl Pts',(0.25155106383961,-0.0536214810419249,
-0.157752224425195));
#28830=CARTESIAN_POINT('Ctrl Pts',(0.181888736963096,0.181850729131537,
-0.149831769499409));
#28831=CARTESIAN_POINT('Ctrl Pts',(-0.0535689079525661,0.251562264853035,
-0.141911314573623));
#28832=CARTESIAN_POINT('Ctrl Pts',(-0.200843250451035,0.125622751888632,
-0.135661037397461));
#28833=CARTESIAN_POINT('Ctrl Pts',(-0.217678878268721,0.0267563773328428,
-0.132050911863228));
#28834=CARTESIAN_POINT('Ctrl Pts',(-0.217520312610843,0.000140789959117728,
-0.131080937970923));
#28835=CARTESIAN_POINT('Ctrl Pts',(-0.217499459018025,0.000127504564585532,
-0.171219062029076));
#28836=CARTESIAN_POINT('Ctrl Pts',(-0.217259599358021,-0.0446051280446579,
-0.169589225833218));
#28837=CARTESIAN_POINT('Ctrl Pts',(-0.182075110663368,-0.162145796313866,
-0.165319237995432));
#28838=CARTESIAN_POINT('Ctrl Pts',(0.0100158074287402,-0.257007551691304,
-0.158409098515717));
#28839=CARTESIAN_POINT('Ctrl Pts',(0.221062284030839,-0.131471158330418,
-0.150488643589931));
#28840=CARTESIAN_POINT('Ctrl Pts',(0.230605935914093,0.113903893563196,
-0.142568188664146));
#28841=CARTESIAN_POINT('Ctrl Pts',(0.0299475598214531,0.255453212845186,
-0.13464773373836));
#28842=CARTESIAN_POINT('Ctrl Pts',(-0.174866704728409,0.173420540348032,
-0.127531358193336));
#28843=CARTESIAN_POINT('Ctrl Pts',(-0.217225558340306,0.0501370445897034,
-0.123055134290242));
#28844=CARTESIAN_POINT('Ctrl Pts',(-0.21762641337835,-0.000181932420623089,
-0.121219062029076));
#28845=CARTESIAN_POINT('Origin',(0.,0.,-1.25608093797092));
#28846=CARTESIAN_POINT('',(-0.217720465391163,-0.00019571213919499,-0.231080937970923));
#28847=CARTESIAN_POINT('',(-0.218083107449943,8.90825909709205E-5,-0.221219062029075));
#28848=CARTESIAN_POINT('',(-0.217775,1.66341393608259E-15,-1.25608093797092));
#28849=CARTESIAN_POINT('Ctrl Pts',(-0.217720465391163,-0.000195712139194972,
-0.231080937970923));
#28850=CARTESIAN_POINT('Ctrl Pts',(-0.217886022198555,-0.01885336084795,
-0.230399398233038));
#28851=CARTESIAN_POINT('Ctrl Pts',(-0.207164530811011,-0.109599730208546,
-0.227077706853224));
#28852=CARTESIAN_POINT('Ctrl Pts',(-0.0805528101499051,-0.244263066255845,
-0.221115863831482));
#28853=CARTESIAN_POINT('Ctrl Pts',(0.161079512847755,-0.200515813094597,
-0.213195408905696));
#28854=CARTESIAN_POINT('Ctrl Pts',(0.255884550354012,0.0260057235181914,
-0.20527495397991));
#28855=CARTESIAN_POINT('Ctrl Pts',(0.117445562765472,0.228822508812962,
-0.197354499054125));
#28856=CARTESIAN_POINT('Ctrl Pts',(-0.128047468266331,0.223062875957976,
-0.189434044128339));
#28857=CARTESIAN_POINT('Ctrl Pts',(-0.216242317834423,0.079865114777898,
-0.184009523767272));
#28858=CARTESIAN_POINT('Ctrl Pts',(-0.218116672648238,0.00400102061694045,
-0.181225155048133));
#28859=CARTESIAN_POINT('Ctrl Pts',(-0.218099944255961,7.07777948932352E-5,
-0.181080937970924));
#28860=CARTESIAN_POINT('Ctrl Pts',(-0.218083107449943,8.90825909709344E-5,
-0.221219062029075));
#28861=CARTESIAN_POINT('Ctrl Pts',(-0.217735478436945,-0.0668451408398962,
-0.218763469018123));
#28862=CARTESIAN_POINT('Ctrl Pts',(-0.148982183502457,-0.206361735170698,
-0.213667724365242));
#28863=CARTESIAN_POINT('Ctrl Pts',(0.0882556230412838,-0.241586718983118,
-0.205931828070432));
#28864=CARTESIAN_POINT('Ctrl Pts',(0.250706501180205,-0.0574408224581984,
-0.198011373144647));
#28865=CARTESIAN_POINT('Ctrl Pts',(0.184633252234903,0.179063563844805,
-0.190090918218861));
#28866=CARTESIAN_POINT('Ctrl Pts',(-0.0497369991668516,0.252347832796275,
-0.182170463293075));
#28867=CARTESIAN_POINT('Ctrl Pts',(-0.199872383158113,0.127864301170981,
-0.175879844563147));
#28868=CARTESIAN_POINT('Ctrl Pts',(-0.217648145076176,0.0278567142749893,
-0.172229377475147));
#28869=CARTESIAN_POINT('Ctrl Pts',(-0.217499459018025,0.000127504564585532,
-0.171219062029076));
#28870=CARTESIAN_POINT('Origin',(0.,0.,-1.25608093797092));
#28871=CARTESIAN_POINT('',(-0.217450356241808,8.11937875190503E-5,-0.281080937970923));
#28872=CARTESIAN_POINT('',(-0.217753140028605,-0.000196789279391762,-0.271219062029075));
#28873=CARTESIAN_POINT('',(-0.217775,1.66341393608259E-15,-1.25608093797092));
#28874=CARTESIAN_POINT('Ctrl Pts',(-0.217450356241808,8.11937875190537E-5,
-0.281080937970923));
#28875=CARTESIAN_POINT('Ctrl Pts',(-0.217310991296762,-0.0413116087876461,
-0.279573641417943));
#28876=CARTESIAN_POINT('Ctrl Pts',(-0.186043658368974,-0.155402323209727,
-0.275426193223034));
#28877=CARTESIAN_POINT('Ctrl Pts',(-0.00186346654402013,-0.257195894705197,
-0.268638593386197));
#28878=CARTESIAN_POINT('Ctrl Pts',(0.214755114225321,-0.141539541029435,
-0.260718138460412));
#28879=CARTESIAN_POINT('Ctrl Pts',(0.235619996010104,0.103133012372812,
-0.252797683534625));
#28880=CARTESIAN_POINT('Ctrl Pts',(0.0417124103716506,0.25379770602124,
-0.24487722860884));
#28881=CARTESIAN_POINT('Ctrl Pts',(-0.170259828869626,0.180062686173349,
-0.237638313420939));
#28882=CARTESIAN_POINT('Ctrl Pts',(-0.217244687508043,0.0534227209925802,
-0.233039549874966));
#28883=CARTESIAN_POINT('Ctrl Pts',(-0.217720465391163,-0.000195712139194972,
-0.231080937970923));
#28884=CARTESIAN_POINT('Ctrl Pts',(-0.217753140028605,-0.000196789279391723,
-0.271219062029075));
#28885=CARTESIAN_POINT('Ctrl Pts',(-0.217911809312456,-0.0177433382782513,
-0.270577863844957));
#28886=CARTESIAN_POINT('Ctrl Pts',(-0.207964564278322,-0.107360671848747,
-0.267296514018909));
#28887=CARTESIAN_POINT('Ctrl Pts',(-0.084258201720026,-0.243009780113768,
-0.261375012550933));
#28888=CARTESIAN_POINT('Ctrl Pts',(0.158011472529912,-0.202942288192858,
-0.253454557625148));
#28889=CARTESIAN_POINT('Ctrl Pts',(0.256250443060382,0.0221112690783347,
-0.245534102699361));
#28890=CARTESIAN_POINT('Ctrl Pts',(0.120911869802921,0.227009950283883,
-0.237613647773576));
#28891=CARTESIAN_POINT('Ctrl Pts',(-0.124640357031449,0.224984397651718,
-0.22969319284779));
#28892=CARTESIAN_POINT('Ctrl Pts',(-0.215674746029958,0.0820896034994043,
-0.224228330932957));
#28893=CARTESIAN_POINT('Ctrl Pts',(-0.218109234717141,0.00511975688706352,
-0.221403620660052));
#28894=CARTESIAN_POINT('Ctrl Pts',(-0.218083107449943,8.90825909709344E-5,
-0.221219062029075));
#28895=CARTESIAN_POINT('Origin',(0.,0.,-1.25608093797092));
#28896=CARTESIAN_POINT('',(-0.218013928034523,0.000137760041710202,-0.331080937970923));
#28897=CARTESIAN_POINT('',(-0.217439216836811,6.44253989956767E-5,-0.321219062029076));
#28898=CARTESIAN_POINT('',(-0.217775,1.66341393608259E-15,-1.25608093797092));
#28899=CARTESIAN_POINT('Ctrl Pts',(-0.218013928034523,0.000137760041710215,
-0.331080937970923));
#28900=CARTESIAN_POINT('Ctrl Pts',(-0.217543145477283,-0.0635095455130215,
-0.328747884602848));
#28901=CARTESIAN_POINT('Ctrl Pts',(-0.154624849848435,-0.199992517491552,
-0.323774679592845));
#28902=CARTESIAN_POINT('Ctrl Pts',(0.0770050110794473,-0.245404623080814,
-0.316161322940912));
#28903=CARTESIAN_POINT('Ctrl Pts',(0.247786424439417,-0.0689571506394352,
-0.308240868015127));
#28904=CARTESIAN_POINT('Ctrl Pts',(0.192705420891506,0.170346181406604,
-0.300320413089341));
#28905=CARTESIAN_POINT('Ctrl Pts',(-0.038030533133535,0.254375469159979,
-0.292399958163555));
#28906=CARTESIAN_POINT('Ctrl Pts',(-0.196787847617761,0.1346707203534,-0.285986799790749));
#28907=CARTESIAN_POINT('Ctrl Pts',(-0.217555100253134,0.0311912278086411,
-0.282213793059872));
#28908=CARTESIAN_POINT('Ctrl Pts',(-0.217450356241808,8.11937875190537E-5,
-0.281080937970923));
#28909=CARTESIAN_POINT('Ctrl Pts',(-0.217439216836811,6.44253989956801E-5,
-0.321219062029076));
#28910=CARTESIAN_POINT('Ctrl Pts',(-0.217331911137438,-0.0402256889947239,
-0.319752107029862));
#28911=CARTESIAN_POINT('Ctrl Pts',(-0.187300136972098,-0.153176608816098,
-0.315645000388719));
#28912=CARTESIAN_POINT('Ctrl Pts',(-0.00577464009454566,-0.257137806088364,
-0.308897742105649));
#28913=CARTESIAN_POINT('Ctrl Pts',(0.212577765931518,-0.144789126731672,
-0.300977287179862));
#28914=CARTESIAN_POINT('Ctrl Pts',(0.237161170678426,0.0995378164850663,
-0.293056832254077));
#28915=CARTESIAN_POINT('Ctrl Pts',(0.0455672956274394,0.253133994867042,
-0.285136377328291));
#28916=CARTESIAN_POINT('Ctrl Pts',(-0.168689180999164,0.182238236202396,
-0.277857120586624));
#28917=CARTESIAN_POINT('Ctrl Pts',(-0.217258484052562,0.0545050730506043,
-0.273218015486885));
#28918=CARTESIAN_POINT('Ctrl Pts',(-0.217753140028605,-0.000196789279391723,
-0.271219062029075));
#28919=CARTESIAN_POINT('Origin',(0.,0.,-1.25608093797092));
#28920=CARTESIAN_POINT('',(-0.217853960473376,-0.000189083574295208,-0.381080937970923));
#28921=CARTESIAN_POINT('',(-0.217986410727679,0.000151022126422644,-0.371219062029075));
#28922=CARTESIAN_POINT('',(-0.217775,1.66341393608259E-15,-1.25608093797092));
#28923=CARTESIAN_POINT('Ctrl Pts',(-0.217853960473376,-0.000189083574295203,
-0.381080937970923));
#28924=CARTESIAN_POINT('Ctrl Pts',(-0.217983094335092,-0.0143654608404639,
-0.380562279429682));
#28925=CARTESIAN_POINT('Ctrl Pts',(-0.210272990147377,-0.100564696279621,
-0.377403469246512));
#28926=CARTESIAN_POINT('Ctrl Pts',(-0.0953904860153474,-0.238859489948667,
-0.371604507421413));
#28927=CARTESIAN_POINT('Ctrl Pts',(0.148471039289085,-0.210022739847858,
-0.363684052495628));
#28928=CARTESIAN_POINT('Ctrl Pts',(0.256998161788665,0.0102540527612222,
-0.355763597569842));
#28929=CARTESIAN_POINT('Ctrl Pts',(0.13126617952173,0.221184065598206,-0.347843142644056));
#28930=CARTESIAN_POINT('Ctrl Pts',(-0.11411762238027,0.230500258184359,
-0.33992268771827));
#28931=CARTESIAN_POINT('Ctrl Pts',(-0.213840835196708,0.0888553987055005,
-0.334335286160559));
#28932=CARTESIAN_POINT('Ctrl Pts',(-0.21807589683158,0.00851561283271852,
-0.331388036244777));
#28933=CARTESIAN_POINT('Ctrl Pts',(-0.218013928034523,0.000137760041710215,
-0.331080937970923));
#28934=CARTESIAN_POINT('Ctrl Pts',(-0.217986410727679,0.000151022126422642,
-0.371219062029075));
#28935=CARTESIAN_POINT('Ctrl Pts',(-0.217490935156433,-0.0624164103471532,
-0.368926350214767));
#28936=CARTESIAN_POINT('Ctrl Pts',(-0.156424859230848,-0.197877144388145,
-0.36399348675853));
#28937=CARTESIAN_POINT('Ctrl Pts',(0.0732640345114102,-0.246547316017172,
-0.356420471660364));
#28938=CARTESIAN_POINT('Ctrl Pts',(0.246709075468843,-0.0727174660550607,
-0.348500016734578));
#28939=CARTESIAN_POINT('Ctrl Pts',(0.195273725240327,0.167395848272668,
-0.340579561808792));
#28940=CARTESIAN_POINT('Ctrl Pts',(-0.0341576376477591,0.254924407577,-0.332659106883006));
#28941=CARTESIAN_POINT('Ctrl Pts',(-0.195727025771613,0.136910137110939,
-0.326205606956434));
#28942=CARTESIAN_POINT('Ctrl Pts',(-0.217525034524685,0.0322864274144955,
-0.322392258671791));
#28943=CARTESIAN_POINT('Ctrl Pts',(-0.217439216836811,6.44253989956801E-5,
-0.321219062029076));
#28944=CARTESIAN_POINT('Origin',(0.,0.,-1.25608093797092));
#28945=CARTESIAN_POINT('',(-0.217421696185068,1.08647192597108E-5,-0.431080937970923));
#28946=CARTESIAN_POINT('',(-0.217886707632715,-0.000182918697169548,-0.421219062029076));
#28947=CARTESIAN_POINT('',(-0.217775,1.66341393608259E-15,-1.25608093797092));
#28948=CARTESIAN_POINT('Ctrl Pts',(-0.217421696185068,1.0864719259724E-5,
-0.431080937970923));
#28949=CARTESIAN_POINT('Ctrl Pts',(-0.217405187502425,-0.0369211171181637,
-0.429736522614587));
#28950=CARTESIAN_POINT('Ctrl Pts',(-0.190967954382265,-0.146401997414083,
-0.425751955616322));
#28951=CARTESIAN_POINT('Ctrl Pts',(-0.0176430849829593,-0.256596808852072,
-0.419127236976129));
#28952=CARTESIAN_POINT('Ctrl Pts',(0.205664628051519,-0.154451486005192,
-0.411206782050343));
#28953=CARTESIAN_POINT('Ctrl Pts',(0.241504807022057,0.0884795397028073,
-0.403286327124557));
#28954=CARTESIAN_POINT('Ctrl Pts',(0.0572083924230321,0.250759647066977,
-0.395365872198771));
#28955=CARTESIAN_POINT('Ctrl Pts',(-0.163751546468412,0.188808241753342,
-0.387964075814226));
#28956=CARTESIAN_POINT('Ctrl Pts',(-0.217325758246069,0.0577972102423321,
-0.38320243107161));
#28957=CARTESIAN_POINT('Ctrl Pts',(-0.217853960473376,-0.000189083574295203,
-0.381080937970923));
#28958=CARTESIAN_POINT('Ctrl Pts',(-0.217886707632715,-0.000182918697169543,
-0.421219062029076));
#28959=CARTESIAN_POINT('Ctrl Pts',(-0.218003945711644,-0.0132515775492716,
-0.420740745041601));
#28960=CARTESIAN_POINT('Ctrl Pts',(-0.210993560192625,-0.0983293864088883,
-0.417622276412197));
#28961=CARTESIAN_POINT('Ctrl Pts',(-0.0990119847176032,-0.237381180110053,
-0.411863656140865));
#28962=CARTESIAN_POINT('Ctrl Pts',(0.145259877725951,-0.212256367893173,
-0.403943201215079));
#28963=CARTESIAN_POINT('Ctrl Pts',(0.25712437710612,0.00634448468750714,
-0.396022746289293));
#28964=CARTESIAN_POINT('Ctrl Pts',(0.134614723864691,0.219162209121448,
-0.388102291363507));
#28965=CARTESIAN_POINT('Ctrl Pts',(-0.11059901597976,0.232209077024282,
-0.380181836437722));
#28966=CARTESIAN_POINT('Ctrl Pts',(-0.213200284022019,0.0910855532474006,
-0.374554093326244));
#28967=CARTESIAN_POINT('Ctrl Pts',(-0.218061495588318,0.00963255304434301,
-0.371566501856695));
#28968=CARTESIAN_POINT('Ctrl Pts',(-0.217986410727679,0.000151022126422642,
-0.371219062029075));
#28969=CARTESIAN_POINT('Origin',(0.,0.,-1.25608093797092));
#28970=CARTESIAN_POINT('',(-0.217893402471771,0.000181423312113251,-0.481080937970923));
#28971=CARTESIAN_POINT('',(-0.217421408434359,-7.14500207714408E-6,-0.471219062029076));
#28972=CARTESIAN_POINT('',(-0.217775,1.66341393608259E-15,-1.25608093797092));
#28973=CARTESIAN_POINT('Ctrl Pts',(-0.217893402471771,0.000181423312113252,
-0.481080937970923));
#28974=CARTESIAN_POINT('Ctrl Pts',(-0.217363839693254,-0.0591076871415457,
-0.478910765799492));
#28975=CARTESIAN_POINT('Ctrl Pts',(-0.161719648021016,-0.191400681792459,
-0.474100441986132));
#28976=CARTESIAN_POINT('Ctrl Pts',(0.0618003361169582,-0.249667617476944,
-0.466649966530844));
#28977=CARTESIAN_POINT('Ctrl Pts',(0.243087789097186,-0.0840328956577408,
-0.458729511605058));
#28978=CARTESIAN_POINT('Ctrl Pts',(0.202795727822344,0.158199537097262,
-0.450809056679272));
#28979=CARTESIAN_POINT('Ctrl Pts',(-0.0223488060129853,0.256229841413087,
-0.442888601753486));
#28980=CARTESIAN_POINT('Ctrl Pts',(-0.192363820390413,0.143705936117005,
-0.436312562184037));
#28981=CARTESIAN_POINT('Ctrl Pts',(-0.217437607115442,0.0356056001855403,
-0.432376674256515));
#28982=CARTESIAN_POINT('Ctrl Pts',(-0.217421696185068,1.0864719259724E-5,
-0.431080937970923));
#28983=CARTESIAN_POINT('Ctrl Pts',(-0.217421408434359,-7.14500207711632E-6,
-0.471219062029076));
#28984=CARTESIAN_POINT('Ctrl Pts',(-0.217431938551127,-0.035831033129075,
-0.469914988226506));
#28985=CARTESIAN_POINT('Ctrl Pts',(-0.19212717751519,-0.144167867511391,
-0.465970762782007));
#28986=CARTESIAN_POINT('Ctrl Pts',(-0.0215433225451699,-0.256298815919768,
-0.45938638569558));
#28987=CARTESIAN_POINT('Ctrl Pts',(0.203291968690357,-0.157561331722472,
-0.451465930769794));
#28988=CARTESIAN_POINT('Ctrl Pts',(0.242822453618414,0.0847965436022809,
-0.443545475844009));
#28989=CARTESIAN_POINT('Ctrl Pts',(0.0610152830318996,0.24986062719984,
-0.435625020918222));
#28990=CARTESIAN_POINT('Ctrl Pts',(-0.162070523658039,0.19095741053108,
-0.428182882979912));
#28991=CARTESIAN_POINT('Ctrl Pts',(-0.217356830274212,0.0588830988884751,
-0.423380896683529));
#28992=CARTESIAN_POINT('Ctrl Pts',(-0.217886707632715,-0.000182918697169543,
-0.421219062029076));
#28993=CARTESIAN_POINT('Origin',(0.,0.,-1.25608093797092));
#28994=CARTESIAN_POINT('',(-0.217980498315397,-0.00015357182946072,-0.531080937970923));
#28995=CARTESIAN_POINT('',(-0.217860768206988,0.000187955723751763,-0.521219062029076));
#28996=CARTESIAN_POINT('',(-0.217775,1.66341393608259E-15,-1.25608093797092));
#28997=CARTESIAN_POINT('Ctrl Pts',(-0.217980498315397,-0.000153571829460759,
-0.531080937970923));
#28998=CARTESIAN_POINT('Ctrl Pts',(-0.218058321777369,-0.00986332003771939,
-0.530725160626326));
#28999=CARTESIAN_POINT('Ctrl Pts',(-0.213065599226933,-0.0915466328813675,
-0.527729231639799));
#29000=CARTESIAN_POINT('Ctrl Pts',(-0.109868600748205,-0.232555566113592,
-0.522093151011346));
#29001=CARTESIAN_POINT('Ctrl Pts',(0.135302924854754,-0.21873801518376,
-0.514172696085558));
#29002=CARTESIAN_POINT('Ctrl Pts',(0.257143054512441,-0.0055362692125341,
-0.506252241159774));
#29003=CARTESIAN_POINT('Ctrl Pts',(0.144592006708923,0.212711899894362,
-0.498331786233987));
#29004=CARTESIAN_POINT('Ctrl Pts',(-0.0997576260038526,0.237068801858992,
-0.490411331308202));
#29005=CARTESIAN_POINT('Ctrl Pts',(-0.211140091175798,0.0978675476797122,
-0.484661048553847));
#29006=CARTESIAN_POINT('Ctrl Pts',(-0.218008086291571,0.013021263903609,
-0.481550917441421));
#29007=CARTESIAN_POINT('Ctrl Pts',(-0.217893402471771,0.000181423312113252,
-0.481080937970923));
#29008=CARTESIAN_POINT('Ctrl Pts',(-0.217860768206988,0.000187955723751776,
-0.521219062029076));
#29009=CARTESIAN_POINT('Ctrl Pts',(-0.217331798266099,-0.0580215318518826,
-0.519089231411411));
#29010=CARTESIAN_POINT('Ctrl Pts',(-0.163406389880727,-0.189253002387909,
-0.514319249151818));
#29011=CARTESIAN_POINT('Ctrl Pts',(0.0579962873891273,-0.250578587347838,
-0.506909115250295));
#29012=CARTESIAN_POINT('Ctrl Pts',(0.241781714379012,-0.087720011286514,
-0.49898866032451));
#29013=CARTESIAN_POINT('Ctrl Pts',(0.205178141054117,0.155097157361885,
-0.491068205398723));
#29014=CARTESIAN_POINT('Ctrl Pts',(-0.0184495234412028,0.256540080441542,
-0.483147750472938));
#29015=CARTESIAN_POINT('Ctrl Pts',(-0.191209471905011,0.145940397476656,
-0.476531369349722));
#29016=CARTESIAN_POINT('Ctrl Pts',(-0.217410619891846,0.0366959180851669,
-0.472555139868434));
#29017=CARTESIAN_POINT('Ctrl Pts',(-0.217421408434359,-7.14500207711632E-6,
-0.471219062029076));
#29018=CARTESIAN_POINT('Origin',(0.,0.,-1.25608093797092));
#29019=CARTESIAN_POINT('',(-0.217437245756766,-6.08897400841611E-5,-0.581080937970923));
#29020=CARTESIAN_POINT('',(-0.218008398413668,-0.000140623921195487,-0.571219062029076));
#29021=CARTESIAN_POINT('',(-0.217775,1.66341393608259E-15,-1.25608093797092));
#29022=CARTESIAN_POINT('Ctrl Pts',(-0.217437245756766,-6.08897400841621E-5,
-0.581080937970923));
#29023=CARTESIAN_POINT('Ctrl Pts',(-0.217518887675132,-0.0325126204013041,
-0.579899403811231));
#29024=CARTESIAN_POINT('Ctrl Pts',(-0.195504947923748,-0.13737285598521,
-0.57607771800961));
#29025=CARTESIAN_POINT('Ctrl Pts',(-0.033356200274203,-0.255030517123049,
-0.569615880566061));
#29026=CARTESIAN_POINT('Ctrl Pts',(0.195798917752269,-0.166781247650396,
-0.561695425640274));
#29027=CARTESIAN_POINT('Ctrl Pts',(0.246479299353905,0.0734925557508373,
-0.553774970714489));
#29028=CARTESIAN_POINT('Ctrl Pts',(0.0724887354193506,0.246776384603724,
-0.545854515788701));
#29029=CARTESIAN_POINT('Ctrl Pts',(-0.156793344004563,0.197438880298673,
-0.538289838207515));
#29030=CARTESIAN_POINT('Ctrl Pts',(-0.217480809622574,0.0621907555351431,
-0.533365312268254));
#29031=CARTESIAN_POINT('Ctrl Pts',(-0.217980498315397,-0.000153571829460759,
-0.531080937970923));
#29032=CARTESIAN_POINT('Ctrl Pts',(-0.218008398413668,-0.000140623921195505,
-0.571219062029076));
#29033=CARTESIAN_POINT('Ctrl Pts',(-0.218073051645397,-0.008746501642567,
-0.570903626238245));
#29034=CARTESIAN_POINT('Ctrl Pts',(-0.21370995744866,-0.089316201135509,
-0.567948038805485));
#29035=CARTESIAN_POINT('Ctrl Pts',(-0.113392555850513,-0.230857804862319,
-0.562352299730795));
#29036=CARTESIAN_POINT('Ctrl Pts',(0.131960746075832,-0.220770376824587,
-0.554431844805011));
#29037=CARTESIAN_POINT('Ctrl Pts',(0.25702911668245,-0.00944621435284863,
-0.546511389879224));
#29038=CARTESIAN_POINT('Ctrl Pts',(0.14781016650087,0.21048836658387,-0.538590934953439));
#29039=CARTESIAN_POINT('Ctrl Pts',(-0.096140787360785,0.238558476675654,
-0.530670480027653));
#29040=CARTESIAN_POINT('Ctrl Pts',(-0.210423490408626,0.100102627577536,
-0.524879855719531));
#29041=CARTESIAN_POINT('Ctrl Pts',(-0.217987512784609,0.0141353208686995,
-0.521729383053339));
#29042=CARTESIAN_POINT('Ctrl Pts',(-0.217860768206988,0.000187955723751776,
-0.521219062029076));
#29043=CARTESIAN_POINT('Origin',(0.,0.,-1.25608093797092));
#29044=CARTESIAN_POINT('',(-0.217759961965208,0.000196790833347493,-0.631080937970923));
#29045=CARTESIAN_POINT('',(-0.217447838183704,-7.77780874032519E-5,-0.621219062029076));
#29046=CARTESIAN_POINT('',(-0.217775,1.66341393608259E-15,-1.25608093797092));
#29047=CARTESIAN_POINT('Ctrl Pts',(-0.217759961965208,0.00019679083334749,
-0.631080937970923));
#29048=CARTESIAN_POINT('Ctrl Pts',(-0.217261836200481,-0.0547288371588338,
-0.629073646996136));
#29049=CARTESIAN_POINT('Ctrl Pts',(-0.168361205872163,-0.182687127116978,
-0.62442620437942));
#29050=CARTESIAN_POINT('Ctrl Pts',(0.046362713408588,-0.252989524617473,
-0.617138610120775));
#29051=CARTESIAN_POINT('Ctrl Pts',(0.237472868244547,-0.0987918903984044,
-0.609218155194989));
#29052=CARTESIAN_POINT('Ctrl Pts',(0.212121624547043,0.145456581701572,
-0.601297700269203));
#29053=CARTESIAN_POINT('Ctrl Pts',(-0.00658283818582227,0.257118391022893,
-0.593377245343417));
#29054=CARTESIAN_POINT('Ctrl Pts',(-0.187556770995067,0.152716308596067,
-0.586638324577325));
#29055=CARTESIAN_POINT('Ctrl Pts',(-0.217336457871426,0.0400011442544223,
-0.58253955545316));
#29056=CARTESIAN_POINT('Ctrl Pts',(-0.217437245756766,-6.08897400841621E-5,
-0.581080937970923));
#29057=CARTESIAN_POINT('Ctrl Pts',(-0.217447838183704,-7.77780874032311E-5,
-0.621219062029076));
#29058=CARTESIAN_POINT('Ctrl Pts',(-0.21754884652787,-0.0314176788091657,
-0.620077869423149));
#29059=CARTESIAN_POINT('Ctrl Pts',(-0.196570461683961,-0.135133614342587,
-0.616296525175294));
#29060=CARTESIAN_POINT('Ctrl Pts',(-0.0372308004467332,-0.254493743118089,
-0.609875029285512));
#29061=CARTESIAN_POINT('Ctrl Pts',(0.193239890732311,-0.169739631253061,
-0.601954574359726));
#29062=CARTESIAN_POINT('Ctrl Pts',(0.247568451193101,0.0697356419774633,
-0.594034119433939));
#29063=CARTESIAN_POINT('Ctrl Pts',(0.0762332818385088,0.245645444753797,
-0.586113664508155));
#29064=CARTESIAN_POINT('Ctrl Pts',(-0.154999187721833,0.199556042356295,
-0.578508645373198));
#29065=CARTESIAN_POINT('Ctrl Pts',(-0.217531913509314,0.063283441872864,
-0.573543777880173));
#29066=CARTESIAN_POINT('Ctrl Pts',(-0.218008398413668,-0.000140623921195505,
-0.571219062029076));
#29067=CARTESIAN_POINT('Origin',(0.,0.,-1.25608093797092));
#29068=CARTESIAN_POINT('',(-0.218079223833456,-9.27439839933367E-5,-0.681080937970923));
#29069=CARTESIAN_POINT('',(-0.217727166021048,0.000196079222951083,-0.671219062029076));
#29070=CARTESIAN_POINT('',(-0.217775,1.66341393608259E-15,-1.25608093797092));
#29071=CARTESIAN_POINT('Ctrl Pts',(-0.218079223833456,-9.27439839933141E-5,
-0.681080937970923));
#29072=CARTESIAN_POINT('Ctrl Pts',(-0.218107480872696,-0.00535093009861154,
-0.680888041822969));
#29073=CARTESIAN_POINT('Ctrl Pts',(-0.215555236352238,-0.0825495299588023,
-0.678054994033087));
#29074=CARTESIAN_POINT('Ctrl Pts',(-0.12393258111715,-0.225375056513412,
-0.672581794601276));
#29075=CARTESIAN_POINT('Ctrl Pts',(0.121624804919859,-0.226628788085249,
-0.664661339675491));
#29076=CARTESIAN_POINT('Ctrl Pts',(0.256318682363535,-0.0213057229917977,
-0.656740884749704));
#29077=CARTESIAN_POINT('Ctrl Pts',(0.157372814497323,0.203437946357048,
-0.648820429823919));
#29078=CARTESIAN_POINT('Ctrl Pts',(-0.0850216071723404,0.242743747755972,
-0.640899974898132));
#29079=CARTESIAN_POINT('Ctrl Pts',(-0.208127415665775,0.106898018501751,
-0.634986810947134));
#29080=CARTESIAN_POINT('Ctrl Pts',(-0.217917011544838,0.0175137966939258,
-0.631713798638064));
#29081=CARTESIAN_POINT('Ctrl Pts',(-0.217759961965208,0.00019679083334749,
-0.631080937970923));
#29082=CARTESIAN_POINT('Ctrl Pts',(-0.217727166021048,0.000196079222951085,
-0.671219062029076));
#29083=CARTESIAN_POINT('Ctrl Pts',(-0.217247214451338,-0.0536463720467488,
-0.669252112608055));
#29084=CARTESIAN_POINT('Ctrl Pts',(-0.169937424913778,-0.180512789837971,
-0.664645011545105));
#29085=CARTESIAN_POINT('Ctrl Pts',(0.0425099313519794,-0.253665337649058,
-0.657397758840227));
#29086=CARTESIAN_POINT('Ctrl Pts',(0.235942990845232,-0.102391908172312,
-0.64947730391444));
#29087=CARTESIAN_POINT('Ctrl Pts',(0.21430916648743,0.142213849352388,-0.641556848988655));
#29088=CARTESIAN_POINT('Ctrl Pts',(-0.00267186632973278,0.257188761260045,
-0.633636394062868));
#29089=CARTESIAN_POINT('Ctrl Pts',(-0.18630534750758,0.154942534370808,
-0.62685713174301));
#29090=CARTESIAN_POINT('Ctrl Pts',(-0.217315163498106,0.0410872514881082,
-0.622718021065078));
#29091=CARTESIAN_POINT('Ctrl Pts',(-0.217447838183704,-7.77780874032311E-5,
-0.621219062029076));
#29092=CARTESIAN_POINT('Origin',(0.,0.,-1.25608093797092));
#29093=CARTESIAN_POINT('',(-0.217495430256374,-0.000124623133544632,-0.731080937970923));
#29094=CARTESIAN_POINT('',(-0.218096740120519,-7.46359541664299E-5,-0.721219062029076));
#29095=CARTESIAN_POINT('',(-0.217775,1.66341393608259E-15,-1.25608093797092));
#29096=CARTESIAN_POINT('Ctrl Pts',(-0.217495430256374,-0.000124623133544624,
-0.731080937970923));
#29097=CARTESIAN_POINT('Ctrl Pts',(-0.217641789012947,-0.0280839662935587,
-0.730062285007874));
#29098=CARTESIAN_POINT('Ctrl Pts',(-0.199669006852885,-0.128327541509715,
-0.726403480402897));
#29099=CARTESIAN_POINT('Ctrl Pts',(-0.0489435840216807,-0.252502923436333,
-0.720104524155992));
#29100=CARTESIAN_POINT('Ctrl Pts',(0.18519517074638,-0.178482350648465,
-0.712184069230205));
#29101=CARTESIAN_POINT('Ctrl Pts',(0.250524722350552,0.0582285518621306,
-0.70426361430442));
#29102=CARTESIAN_POINT('Ctrl Pts',(0.0874958422396386,0.241862932983866,
-0.696343159378634));
#29103=CARTESIAN_POINT('Ctrl Pts',(-0.149374512656238,0.205931212802491,
-0.688615600600802));
#29104=CARTESIAN_POINT('Ctrl Pts',(-0.217720729403906,0.0666173743561128,
-0.683528193464898));
#29105=CARTESIAN_POINT('Ctrl Pts',(-0.218079223833456,-9.27439839933141E-5,
-0.681080937970923));
#29106=CARTESIAN_POINT('Ctrl Pts',(-0.218096740120519,-7.46359541664186E-5,
-0.721219062029076));
#29107=CARTESIAN_POINT('Ctrl Pts',(-0.218115278524842,-0.0042322574475895,
-0.721066507434889));
#29108=CARTESIAN_POINT('Ctrl Pts',(-0.216126462641042,-0.0803247351229268,
-0.718273801198772));
#29109=CARTESIAN_POINT('Ctrl Pts',(-0.127345709562336,-0.223464243323681,
-0.712840943320728));
#29110=CARTESIAN_POINT('Ctrl Pts',(0.118164206801822,-0.228452222617896,
-0.704920488394942));
#29111=CARTESIAN_POINT('Ctrl Pts',(0.255965020858851,-0.0252013072059438,
-0.697000033469156));
#29112=CARTESIAN_POINT('Ctrl Pts',(0.160448459333854,0.201021117511452,
-0.68907957854337));
#29113=CARTESIAN_POINT('Ctrl Pts',(-0.0813201694554329,0.244008663427961,
-0.681159123617584));
#29114=CARTESIAN_POINT('Ctrl Pts',(-0.20733152168619,0.109136913690184,
-0.67520561811282));
#29115=CARTESIAN_POINT('Ctrl Pts',(-0.217891432808594,0.0186240354207517,
-0.671892264249983));
#29116=CARTESIAN_POINT('Ctrl Pts',(-0.217727166021048,0.000196079222951085,
-0.671219062029076));
#29117=CARTESIAN_POINT('Origin',(0.,0.,-1.25608093797092));
#29118=CARTESIAN_POINT('',(-0.217632492219457,0.000183354111511343,-0.781080937970924));
#29119=CARTESIAN_POINT('',(-0.21751582202118,-0.000138136452134785,-0.771219062029076));
#29120=CARTESIAN_POINT('',(-0.217775,1.66341393608259E-15,-1.25608093797092));
#29121=CARTESIAN_POINT('Ctrl Pts',(-0.217632492219457,0.000183354111511339,
-0.781080937970924));
#29122=CARTESIAN_POINT('Ctrl Pts',(-0.217225850738349,-0.0503605582290492,
-0.77923652819278));
#29123=CARTESIAN_POINT('Ctrl Pts',(-0.174560998031809,-0.173873973729166,
-0.774751966772707));
#29124=CARTESIAN_POINT('Ctrl Pts',(0.0307503329195962,-0.255357823036844,
-0.767627253710707));
#29125=CARTESIAN_POINT('Ctrl Pts',(0.230962826542383,-0.113178502889618,
-0.759706798784921));
#29126=CARTESIAN_POINT('Ctrl Pts',(0.220647958398849,0.132165348012261,
-0.751786343859134));
#29127=CARTESIAN_POINT('Ctrl Pts',(0.00920794273158324,0.257037768725599,
-0.743865888933349));
#29128=CARTESIAN_POINT('Ctrl Pts',(-0.182352457983248,0.161687891688101,
-0.736964086970612));
#29129=CARTESIAN_POINT('Ctrl Pts',(-0.217262455397384,0.0443812484840306,
-0.732702436649803));
#29130=CARTESIAN_POINT('Ctrl Pts',(-0.217495430256374,-0.000124623133544624,
-0.731080937970923));
#29131=CARTESIAN_POINT('Ctrl Pts',(-0.21751582202118,-0.000138136452134743,
-0.771219062029076));
#29132=CARTESIAN_POINT('Ctrl Pts',(-0.217672533053156,-0.0269838912366882,
-0.770240750619793));
#29133=CARTESIAN_POINT('Ctrl Pts',(-0.200644381604158,-0.126086035057239,
-0.766622287568582));
#29134=CARTESIAN_POINT('Ctrl Pts',(-0.0527779420396886,-0.251729391653449,
-0.760363672875443));
#29135=CARTESIAN_POINT('Ctrl Pts',(0.182459421962995,-0.181278120922218,
-0.752443217949657));
#29136=CARTESIAN_POINT('Ctrl Pts',(0.251381274026667,0.0544118815782901,
-0.744522763023871));
#29137=CARTESIAN_POINT('Ctrl Pts',(0.0911639299237252,0.240504336071146,
-0.736602308098085));
#29138=CARTESIAN_POINT('Ctrl Pts',(-0.147464756036621,0.208010300530612,
-0.728834407766487));
#29139=CARTESIAN_POINT('Ctrl Pts',(-0.217794447815865,0.0677206802586771,
-0.723706659076817));
#29140=CARTESIAN_POINT('Ctrl Pts',(-0.218096740120519,-7.46359541664186E-5,
-0.721219062029076));
#29141=CARTESIAN_POINT('Origin',(0.,0.,-1.25608093797092));
#29142=CARTESIAN_POINT('',(-0.218127064665478,-1.51157432300434E-5,-0.831080937970924));
#29143=CARTESIAN_POINT('',(-0.217603720989924,0.0001758774262937,-0.821219062029076));
#29144=CARTESIAN_POINT('',(-0.217775,1.66341393608259E-15,-1.25608093797092));
#29145=CARTESIAN_POINT('Ctrl Pts',(-0.218127064665478,-1.51157432300175E-5,
-0.831080937970924));
#29146=CARTESIAN_POINT('Ctrl Pts',(-0.218127886525049,-0.000832818950451307,
-0.831050923019614));
#29147=CARTESIAN_POINT('Ctrl Pts',(-0.217754036594478,-0.0735759187401932,
-0.828380756426375));
#29148=CARTESIAN_POINT('Ctrl Pts',(-0.137529414910091,-0.217345027077388,
-0.823070438191206));
#29149=CARTESIAN_POINT('Ctrl Pts',(0.107488237249403,-0.233665315384629,
-0.815149983265423));
#29150=CARTESIAN_POINT('Ctrl Pts',(0.254528152697761,-0.0369948678203813,
-0.807229528339635));
#29151=CARTESIAN_POINT('Ctrl Pts',(0.169560427414887,0.193397161860414,
-0.79930907341385));
#29152=CARTESIAN_POINT('Ctrl Pts',(-0.0699651112530573,0.247503704958389,
-0.791388618488063));
#29153=CARTESIAN_POINT('Ctrl Pts',(-0.204789490261868,0.115941739323129,
-0.785312573340423));
#29154=CARTESIAN_POINT('Ctrl Pts',(-0.217807931351206,0.021989737641606,
-0.781876679834709));
#29155=CARTESIAN_POINT('Ctrl Pts',(-0.217632492219457,0.000183354111511339,
-0.781080937970924));
#29156=CARTESIAN_POINT('Ctrl Pts',(-0.217603720989924,0.000175877426293707,
-0.821219062029076));
#29157=CARTESIAN_POINT('Ctrl Pts',(-0.21722579264226,-0.0492790478079207,
-0.819414993804698));
#29158=CARTESIAN_POINT('Ctrl Pts',(-0.176029688244654,-0.171678173502806,
-0.814970773938393));
#29159=CARTESIAN_POINT('Ctrl Pts',(0.026863340058709,-0.25579593184617,
-0.807886402430158));
#29160=CARTESIAN_POINT('Ctrl Pts',(0.229214913121365,-0.116677853043863,
-0.799965947504372));
#29161=CARTESIAN_POINT('Ctrl Pts',(0.222632383413667,0.128794486076502,
-0.792045492578587));
#29162=CARTESIAN_POINT('Ctrl Pts',(0.0131158620091436,0.256868004920654,
-0.7841250376528));
#29163=CARTESIAN_POINT('Ctrl Pts',(-0.181000476366041,0.163902138278909,
-0.777182894136297));
#29164=CARTESIAN_POINT('Ctrl Pts',(-0.217249619771706,0.0454642708727976,
-0.772880902261722));
#29165=CARTESIAN_POINT('Ctrl Pts',(-0.21751582202118,-0.000138136452134743,
-0.771219062029076));
#29166=CARTESIAN_POINT('Origin',(0.,0.,-1.25608093797092));
#29167=CARTESIAN_POINT('',(-0.217590234620949,-0.000171676759354653,-0.881080937970924));
#29168=CARTESIAN_POINT('',(-0.21812823151327,5.20618463971455E-6,-0.871219062029076));
#29169=CARTESIAN_POINT('',(-0.217775,1.66341393608259E-15,-1.25608093797092));
#29170=CARTESIAN_POINT('Ctrl Pts',(-0.217590234620949,-0.000171676759354655,
-0.881080937970924));
#29171=CARTESIAN_POINT('Ctrl Pts',(-0.217764472112696,-0.0236346228518696,
-0.880225166204519));
#29172=CARTESIAN_POINT('Ctrl Pts',(-0.203474532729487,-0.119276866693917,
-0.876729242796186));
#29173=CARTESIAN_POINT('Ctrl Pts',(-0.0643464817567947,-0.249023555203761,
-0.870593167745921));
#29174=CARTESIAN_POINT('Ctrl Pts',(0.173893356378981,-0.189510689323927,
-0.862672712820138));
#29175=CARTESIAN_POINT('Ctrl Pts',(0.253625827354345,0.042745063570017,
-0.85475225789435));
#29176=CARTESIAN_POINT('Ctrl Pts',(0.102173145688224,0.236037812777863,
-0.846831802968565));
#29177=CARTESIAN_POINT('Ctrl Pts',(-0.141485588421475,0.214260087681797,
-0.838941362994089));
#29178=CARTESIAN_POINT('Ctrl Pts',(-0.218055594757132,0.0710933502062712,
-0.833691074661543));
#29179=CARTESIAN_POINT('Ctrl Pts',(-0.218127064665478,-1.51157432300175E-5,
-0.831080937970924));
#29180=CARTESIAN_POINT('Ctrl Pts',(-0.21812823151327,5.20618463970728E-6,
-0.871219062029076));
#29181=CARTESIAN_POINT('Ctrl Pts',(-0.218102942100602,-0.0716385923522861,
-0.868589236989604));
#29182=CARTESIAN_POINT('Ctrl Pts',(-0.140499760598608,-0.21525449840371,
-0.863319260308203));
#29183=CARTESIAN_POINT('Ctrl Pts',(0.103922264034112,-0.235272949626989,
-0.855409131984872));
#29184=CARTESIAN_POINT('Ctrl Pts',(0.25393610059609,-0.0408614072470928,
-0.847488677059087));
#29185=CARTESIAN_POINT('Ctrl Pts',(0.172481964081841,0.1907961473789,-0.839568222133301));
#29186=CARTESIAN_POINT('Ctrl Pts',(-0.0661930265154354,0.248539093562536,
-0.831647767207517));
#29187=CARTESIAN_POINT('Ctrl Pts',(-0.203910920659895,0.11818294676327,
-0.825531380506107));
#29188=CARTESIAN_POINT('Ctrl Pts',(-0.217778869368591,0.0230954335416578,
-0.822055145446627));
#29189=CARTESIAN_POINT('Ctrl Pts',(-0.217603720989924,0.000175877426293707,
-0.821219062029076));
#29190=CARTESIAN_POINT('Origin',(0.,0.,-1.25608093797092));
#29191=CARTESIAN_POINT('',(-0.217526565113027,0.000144321015786189,-0.931080937970924));
#29192=CARTESIAN_POINT('',(-0.217618267924705,-0.000179898412300761,-0.921219062029076));
#29193=CARTESIAN_POINT('',(-0.217775,1.66341393608259E-15,-1.25608093797092));
#29194=CARTESIAN_POINT('Ctrl Pts',(-0.217526565113027,0.000144321015786177,
-0.931080937970924));
#29195=CARTESIAN_POINT('Ctrl Pts',(-0.217244272156895,-0.0459926317880253,
-0.929399409389424));
#29196=CARTESIAN_POINT('Ctrl Pts',(-0.180331437388558,-0.164981497104693,
-0.925077729165994));
#29197=CARTESIAN_POINT('Ctrl Pts',(0.0150220433400717,-0.256763585765983,
-0.918115897300639));
#29198=CARTESIAN_POINT('Ctrl Pts',(0.22358220268487,-0.127138504801763,
-0.910195442374852));
#29199=CARTESIAN_POINT('Ctrl Pts',(0.228342590551659,0.118375935480206,
-0.902274987449066));
#29200=CARTESIAN_POINT('Ctrl Pts',(0.0249640155933997,0.255988278415915,
-0.894354532523281));
#29201=CARTESIAN_POINT('Ctrl Pts',(-0.176736969944704,0.170604861907604,
-0.887289849363898));
#29202=CARTESIAN_POINT('Ctrl Pts',(-0.217226929957205,0.0487511908457016,
-0.882865317846447));
#29203=CARTESIAN_POINT('Ctrl Pts',(-0.217590234620949,-0.000171676759354655,
-0.881080937970924));
#29204=CARTESIAN_POINT('Ctrl Pts',(-0.217618267924705,-0.000179898412300724,
-0.921219062029077));
#29205=CARTESIAN_POINT('Ctrl Pts',(-0.217793826238208,-0.0225295119375463,
-0.920403631816438));
#29206=CARTESIAN_POINT('Ctrl Pts',(-0.20436332104689,-0.117035495875518,
-0.916948049961871));
#29207=CARTESIAN_POINT('Ctrl Pts',(-0.0681261445426857,-0.248016181363272,
-0.910852316465374));
#29208=CARTESIAN_POINT('Ctrl Pts',(0.170991197855606,-0.192133308002639,
-0.902931861539589));
#29209=CARTESIAN_POINT('Ctrl Pts',(0.254246550215305,0.0388830231818767,
-0.895011406613802));
#29210=CARTESIAN_POINT('Ctrl Pts',(0.105750948292417,0.234456679843913,
-0.887090951688017));
#29211=CARTESIAN_POINT('Ctrl Pts',(-0.139138815762931,0.216318255670307,
-0.879170496762231));
#29212=CARTESIAN_POINT('Ctrl Pts',(-0.218000660033129,0.072492888641203,
-0.873879866875917));
#29213=CARTESIAN_POINT('Ctrl Pts',(-0.218128330817865,0.000286531753771226,
-0.871229388631533));
#29214=CARTESIAN_POINT('Ctrl Pts',(-0.21812823151327,5.20618463970728E-6,
-0.871219062029076));
#29215=CARTESIAN_POINT('Origin',(0.,0.,-1.25608093797092));
#29216=CARTESIAN_POINT('',(-0.218104054822873,6.54679023023512E-5,-0.981080937970924));
#29217=CARTESIAN_POINT('',(-0.2175051044321,0.000131354540280196,-0.971219062029076));
#29218=CARTESIAN_POINT('',(-0.217775,1.66341393608259E-15,-1.25608093797092));
#29219=CARTESIAN_POINT('Ctrl Pts',(-0.218104054822873,6.54679023023327E-5,
-0.981080937970924));
#29220=CARTESIAN_POINT('Ctrl Pts',(-0.217832592967684,-0.0682603177041455,
-0.978573652574329));
#29221=CARTESIAN_POINT('Ctrl Pts',(-0.146522207495947,-0.209021230560728,
-0.973426215535804));
#29222=CARTESIAN_POINT('Ctrl Pts',(0.092946507651719,-0.239821073941797,
-0.965638626855354));
#29223=CARTESIAN_POINT('Ctrl Pts',(0.251778214672948,-0.05254456561971,
-0.957718171929568));
#29224=CARTESIAN_POINT('Ctrl Pts',(0.181108905951714,0.182627393722108,
-0.949797717003781));
#29225=CARTESIAN_POINT('Ctrl Pts',(-0.0546448916053246,0.251330731481492,
-0.941877262077996));
#29226=CARTESIAN_POINT('Ctrl Pts',(-0.201112491437176,0.124992019589862,
-0.93563833573371));
#29227=CARTESIAN_POINT('Ctrl Pts',(-0.217687497576811,0.026446548276287,
-0.932039561031353));
#29228=CARTESIAN_POINT('Ctrl Pts',(-0.217526565113027,0.000144321015786177,
-0.931080937970924));
#29229=CARTESIAN_POINT('Ctrl Pts',(-0.2175051044321,0.000131354540280217,
-0.971219062029076));
#29230=CARTESIAN_POINT('Ctrl Pts',(-0.217255883023214,-0.0449098808917798,
-0.969577875001342));
#29231=CARTESIAN_POINT('Ctrl Pts',(-0.18169579707604,-0.162768967076207,
-0.96529653633168));
#29232=CARTESIAN_POINT('Ctrl Pts',(0.0111154911491714,-0.256962338971068,
-0.958375046020089));
#29233=CARTESIAN_POINT('Ctrl Pts',(0.221622841759585,-0.130523997019855,
-0.950454591094304));
#29234=CARTESIAN_POINT('Ctrl Pts',(0.230116418626786,0.114889649949471,
-0.942534136168517));
#29235=CARTESIAN_POINT('Ctrl Pts',(0.0288541519363172,0.255579020471033,
-0.934613681242733));
#29236=CARTESIAN_POINT('Ctrl Pts',(-0.175281056344178,0.172802918894569,
-0.927508656529584));
#29237=CARTESIAN_POINT('Ctrl Pts',(-0.21722541392963,0.0498327428950334,
-0.923043783458366));
#29238=CARTESIAN_POINT('Ctrl Pts',(-0.217618267924705,-0.000179898412300724,
-0.921219062029077));
#29239=CARTESIAN_POINT('Origin',(0.,0.,-1.25608093797092));
#29240=CARTESIAN_POINT('',(-0.217711384278981,-0.000195092093718535,-1.03108093797092));
#29241=CARTESIAN_POINT('',(-0.218088181886173,8.40274599361677E-5,-1.02121906202908));
#29242=CARTESIAN_POINT('',(-0.217775,1.66341393608259E-15,-1.25608093797092));
#29243=CARTESIAN_POINT('Ctrl Pts',(-0.217711384278981,-0.000195092093718539,
-1.03108093797092));
#29244=CARTESIAN_POINT('Ctrl Pts',(-0.217878581251591,-0.0191654947610302,
-1.03038804740116));
#29245=CARTESIAN_POINT('Ctrl Pts',(-0.206935794297685,-0.110229868580331,
-1.02705500518947));
#29246=CARTESIAN_POINT('Ctrl Pts',(-0.0795068333803697,-0.244605521341649,
-1.02108181133586));
#29247=CARTESIAN_POINT('Ctrl Pts',(0.161936074723358,-0.199824697090791,
-1.01316135641007));
#29248=CARTESIAN_POINT('Ctrl Pts',(0.25577092546644,0.0271004554068604,
-1.00524090148428));
#29249=CARTESIAN_POINT('Ctrl Pts',(0.116465321567834,0.229322980077886,
-0.997320446558497));
#29250=CARTESIAN_POINT('Ctrl Pts',(-0.129000815316647,0.222512899840908,
-0.98939999163271));
#29251=CARTESIAN_POINT('Ctrl Pts',(-0.216398828568288,0.0792394791905274,
-0.98398682210352));
#29252=CARTESIAN_POINT('Ctrl Pts',(-0.218118440148731,0.00368619277284598,
-0.981213804216257));
#29253=CARTESIAN_POINT('Ctrl Pts',(-0.218104054822873,6.54679023023327E-5,
-0.981080937970924));
#29254=CARTESIAN_POINT('Ctrl Pts',(-0.218088181886173,8.40274599361686E-5,
-1.02121906202908));
#29255=CARTESIAN_POINT('Ctrl Pts',(-0.217755967501094,-0.0671554398934883,
-1.01875211818625));
#29256=CARTESIAN_POINT('Ctrl Pts',(-0.148446081963974,-0.206947166699799,
-1.01364502270149));
#29257=CARTESIAN_POINT('Ctrl Pts',(0.0892886006322762,-0.241206848519812,
-1.0058977755748));
#29258=CARTESIAN_POINT('Ctrl Pts',(0.250950003708668,-0.0563674856785394,
-0.997977320649019));
#29259=CARTESIAN_POINT('Ctrl Pts',(0.183865322083874,0.179851997660945,
-0.990056865723231));
#29260=CARTESIAN_POINT('Ctrl Pts',(-0.0508163781729916,0.252132690320144,
-0.982136410797448));
#29261=CARTESIAN_POINT('Ctrl Pts',(-0.200147761824428,0.127233622778126,
-0.975857142899395));
#29262=CARTESIAN_POINT('Ctrl Pts',(-0.217656801566168,0.0275472429283243,
-0.972218026643271));
#29263=CARTESIAN_POINT('Ctrl Pts',(-0.2175051044321,0.000131354540280217,
-0.971219062029076));
#29264=CARTESIAN_POINT('Origin',(0.,0.,-1.25608093797092));
#29265=CARTESIAN_POINT('',(-0.217453911095485,8.60469890504272E-5,-1.08108093797092));
#29266=CARTESIAN_POINT('',(-0.217743889400727,-0.000196664163112259,-1.07121906202908));
#29267=CARTESIAN_POINT('',(-0.217775,1.66341393608259E-15,-1.25608093797092));
#29268=CARTESIAN_POINT('Ctrl Pts',(-0.217453911095485,8.60469890503895E-5,
-1.08108093797092));
#29269=CARTESIAN_POINT('Ctrl Pts',(-0.217305410614029,-0.0416168581794606,
-1.07956229058607));
#29270=CARTESIAN_POINT('Ctrl Pts',(-0.185685765260903,-0.156028526245301,
-1.07540349155928));
#29271=CARTESIAN_POINT('Ctrl Pts',(-0.000762821507371324,-0.25720122800503,
-1.06860454089057));
#29272=CARTESIAN_POINT('Ctrl Pts',(0.215358791521507,-0.140619426360152,
-1.06068408596478));
#29273=CARTESIAN_POINT('Ctrl Pts',(0.235176530521566,0.104140400581766,
-1.052763631039));
#29274=CARTESIAN_POINT('Ctrl Pts',(0.0406259830504325,0.253973834313976,
-1.04484317611321));
#29275=CARTESIAN_POINT('Ctrl Pts',(-0.17069690156357,0.1794495265795,-1.03761561175719));
#29276=CARTESIAN_POINT('Ctrl Pts',(-0.217241503217881,0.0531182711551457,
-1.03302819904309));
#29277=CARTESIAN_POINT('Ctrl Pts',(-0.217711384278981,-0.000195092093718539,
-1.03108093797092));
#29278=CARTESIAN_POINT('Ctrl Pts',(-0.217743889400727,-0.000196664163112275,
-1.07121906202908));
#29279=CARTESIAN_POINT('Ctrl Pts',(-0.217904661477969,-0.0180557774320445,
-1.07056651301308));
#29280=CARTESIAN_POINT('Ctrl Pts',(-0.207741505551685,-0.107990640708861,
-1.06727381235516));
#29281=CARTESIAN_POINT('Ctrl Pts',(-0.0832175410220989,-0.243368068736343,
-1.06134096005531));
#29282=CARTESIAN_POINT('Ctrl Pts',(0.158878438899101,-0.202264296402348,
-1.05342050512952));
#29283=CARTESIAN_POINT('Ctrl Pts',(0.25615348338552,0.0232076117179531,
-1.04550005020373));
#29284=CARTESIAN_POINT('Ctrl Pts',(0.119939351168713,0.227525266045112,
-1.03757959527795));
#29285=CARTESIAN_POINT('Ctrl Pts',(-0.125601956730251,0.224448986095295,
-1.02965914035216));
#29286=CARTESIAN_POINT('Ctrl Pts',(-0.215836233287728,0.081463554320085,
-1.0242056292692));
#29287=CARTESIAN_POINT('Ctrl Pts',(-0.21811150715263,0.00480501054465392,
-1.02139226982818));
#29288=CARTESIAN_POINT('Ctrl Pts',(-0.218088181886173,8.40274599361686E-5,
-1.02121906202908));
#29289=CARTESIAN_POINT('Origin',(0.,0.,-1.25608093797092));
#29290=CARTESIAN_POINT('',(-0.21801873929181,0.00014895038204359,-1.13108093797092));
#29291=CARTESIAN_POINT('',(-0.217441534898734,7.07751596318168E-5,-1.12121906202908));
#29292=CARTESIAN_POINT('',(-0.217775,1.66341393608259E-15,-1.25608093797092));
#29293=CARTESIAN_POINT('Ctrl Pts',(-0.21801873929181,0.000148950382043584,
-1.13108093797092));
#29294=CARTESIAN_POINT('Ctrl Pts',(-0.217555670191414,-0.0637989277634247,
-1.12873653377097));
#29295=CARTESIAN_POINT('Ctrl Pts',(-0.154117328807783,-0.200610241566758,
-1.12375197792909));
#29296=CARTESIAN_POINT('Ctrl Pts',(0.0780566987792774,-0.245059402025012,
-1.11612727044528));
#29297=CARTESIAN_POINT('Ctrl Pts',(0.248078039310978,-0.0679032867325597,
-1.1082068155195));
#29298=CARTESIAN_POINT('Ctrl Pts',(0.191975348375761,0.171172964635631,
-1.10028636059371));
#29299=CARTESIAN_POINT('Ctrl Pts',(-0.0391190265108933,0.254208440109437,
-1.09236590566793));
#29300=CARTESIAN_POINT('Ctrl Pts',(-0.197082164878129,0.134040930345383,
-1.085964098127));
#29301=CARTESIAN_POINT('Ctrl Pts',(-0.217563577054673,0.0308831801123549,
-1.082202442228));
#29302=CARTESIAN_POINT('Ctrl Pts',(-0.217453911095485,8.60469890503895E-5,
-1.08108093797092));
#29303=CARTESIAN_POINT('Ctrl Pts',(-0.217441534898734,7.07751596318099E-5,
-1.12121906202908));
#29304=CARTESIAN_POINT('Ctrl Pts',(-0.217325562139716,-0.0405305200113168,
-1.11974075619799));
#29305=CARTESIAN_POINT('Ctrl Pts',(-0.186950053002431,-0.153805877485014,
-1.11562229872497));
#29306=CARTESIAN_POINT('Ctrl Pts',(-0.00467359635069057,-0.257158283796502,
-1.10886368961002));
#29307=CARTESIAN_POINT('Ctrl Pts',(0.213195046788718,-0.143879137770345,
-1.10094323468424));
#29308=CARTESIAN_POINT('Ctrl Pts',(0.236733244856063,0.100552273737884,
-1.09302277975845));
#29309=CARTESIAN_POINT('Ctrl Pts',(0.0444835839728878,0.253326392640624,
-1.08510232483266));
#29310=CARTESIAN_POINT('Ctrl Pts',(-0.169133800272843,0.181626810356099,
-1.07783441892287));
#29311=CARTESIAN_POINT('Ctrl Pts',(-0.217254192849094,0.054200506869408,
-1.07320666465501));
#29312=CARTESIAN_POINT('Ctrl Pts',(-0.217743889400727,-0.000196664163112275,
-1.07121906202908));
#29313=CARTESIAN_POINT('Origin',(0.03,0.28,0.6));
#29314=CARTESIAN_POINT('',(0.03,0.28,0.6));
#29315=CARTESIAN_POINT('',(-0.03,0.28,0.6));
#29316=CARTESIAN_POINT('',(0.015,0.28,0.6));
#29317=CARTESIAN_POINT('',(0.03,0.28,0.57));
#29318=CARTESIAN_POINT('',(0.03,0.28,0.6));
#29319=CARTESIAN_POINT('',(-0.03,0.28,0.57));
#29320=CARTESIAN_POINT('',(-0.03,0.28,0.57));
#29321=CARTESIAN_POINT('',(-0.03,0.28,0.6));
#29322=CARTESIAN_POINT('Origin',(0.03,0.42,0.6));
#29323=CARTESIAN_POINT('',(0.03,0.42,0.6));
#29324=CARTESIAN_POINT('',(0.03,0.21,0.6));
#29325=CARTESIAN_POINT('',(0.03,0.42,0.57));
#29326=CARTESIAN_POINT('',(0.03,0.42,0.6));
#29327=CARTESIAN_POINT('',(0.03,0.28,0.57));
#29328=CARTESIAN_POINT('Origin',(-0.03,0.42,0.6));
#29329=CARTESIAN_POINT('',(-0.03,0.42,0.6));
#29330=CARTESIAN_POINT('',(-0.015,0.42,0.6));
#29331=CARTESIAN_POINT('',(-0.03,0.42,0.57));
#29332=CARTESIAN_POINT('',(-0.03,0.42,0.6));
#29333=CARTESIAN_POINT('',(0.03,0.42,0.57));
#29334=CARTESIAN_POINT('Origin',(-0.03,0.28,0.6));
#29335=CARTESIAN_POINT('',(-0.03,0.14,0.6));
#29336=CARTESIAN_POINT('',(-0.03,0.42,0.57));
#29337=CARTESIAN_POINT('Origin',(0.,0.35,0.57));
#29338=CARTESIAN_POINT('Origin',(0.,0.,-1.2));
#29339=CARTESIAN_POINT('',(-0.151,-1.8492166667125E-17,-1.2));
#29340=CARTESIAN_POINT('Origin',(0.,0.,-1.2));
#29341=CARTESIAN_POINT('',(-0.151,-1.8492166667125E-17,-1.05));
#29342=CARTESIAN_POINT('',(-0.151,-1.8492166667125E-17,-1.2));
#29343=CARTESIAN_POINT('Origin',(0.,0.,-1.05));
#29344=CARTESIAN_POINT('Origin',(0.,0.,-1.05));
#29345=CARTESIAN_POINT('Ctrl Pts',(-0.0944853208817847,0.196210282000883,
-1.18014778394209));
#29346=CARTESIAN_POINT('Ctrl Pts',(-0.159582249462734,0.164862769920135,
-1.17750763230016));
#29347=CARTESIAN_POINT('Ctrl Pts',(-0.255023143260422,0.0328527272961977,
-1.17222732901631));
#29348=CARTESIAN_POINT('Ctrl Pts',(-0.166183579550698,-0.196528621075993,
-1.16430687409052));
#29349=CARTESIAN_POINT('Ctrl Pts',(0.0743494844831576,-0.246142736672221,
-1.15638641916474));
#29350=CARTESIAN_POINT('Ctrl Pts',(0.247001644414856,-0.0717076563344237,
-1.14846596423895));
#29351=CARTESIAN_POINT('Ctrl Pts',(0.194564222666998,0.168254406153596,
-1.14054550931316));
#29352=CARTESIAN_POINT('Ctrl Pts',(-0.0352527091661894,0.254763023235567,
-1.13262505438738));
#29353=CARTESIAN_POINT('Ctrl Pts',(-0.232920168884155,0.109095201333321,
-1.12470459946159));
#29354=CARTESIAN_POINT('Ctrl Pts',(-0.218284479061633,-0.136038973337895,
-1.11678414453581));
#29355=CARTESIAN_POINT('Ctrl Pts',(-0.00467359635069057,-0.257158283796502,
-1.10886368961002));
#29356=CARTESIAN_POINT('Ctrl Pts',(0.213195046788718,-0.143879137770345,
-1.10094323468424));
#29357=CARTESIAN_POINT('Ctrl Pts',(0.236733244856063,0.100552273737884,
-1.09302277975845));
#29358=CARTESIAN_POINT('Ctrl Pts',(0.0444835839728878,0.253326392640624,
-1.08510232483266));
#29359=CARTESIAN_POINT('Ctrl Pts',(-0.188313439582864,0.175189262533144,
-1.07718186990688));
#29360=CARTESIAN_POINT('Ctrl Pts',(-0.249459071805079,-0.0626369865404807,
-1.06926141498109));
#29361=CARTESIAN_POINT('Ctrl Pts',(-0.0832175410220989,-0.243368068736343,
-1.06134096005531));
#29362=CARTESIAN_POINT('Ctrl Pts',(0.158878438899101,-0.202264296402348,
-1.05342050512952));
#29363=CARTESIAN_POINT('Ctrl Pts',(0.25615348338552,0.0232076117179531,
-1.04550005020373));
#29364=CARTESIAN_POINT('Ctrl Pts',(0.119939351168713,0.227525266045112,
-1.03757959527795));
#29365=CARTESIAN_POINT('Ctrl Pts',(-0.125601956730251,0.224448986095295,
-1.02965914035216));
#29366=CARTESIAN_POINT('Ctrl Pts',(-0.256654504229033,0.0167828330074643,
-1.02173868542638));
#29367=CARTESIAN_POINT('Ctrl Pts',(-0.15376119589656,-0.206181211517413,
-1.01381823050059));
#29368=CARTESIAN_POINT('Ctrl Pts',(0.0892886006322762,-0.241206848519812,
-1.0058977755748));
#29369=CARTESIAN_POINT('Ctrl Pts',(0.250950003708668,-0.0563674856785394,
-0.997977320649019));
#29370=CARTESIAN_POINT('Ctrl Pts',(0.183865322083874,0.179851997660945,
-0.990056865723231));
#29371=CARTESIAN_POINT('Ctrl Pts',(-0.0508163781729916,0.252132690320144,
-0.982136410797448));
#29372=CARTESIAN_POINT('Ctrl Pts',(-0.239177905729943,0.0945892551935581,
-0.974215955871661));
#29373=CARTESIAN_POINT('Ctrl Pts',(-0.209523858011382,-0.14917422935663,
-0.966295500945875));
#29374=CARTESIAN_POINT('Ctrl Pts',(0.0111154911491714,-0.256962338971068,
-0.958375046020089));
#29375=CARTESIAN_POINT('Ctrl Pts',(0.221622841759585,-0.130523997019855,
-0.950454591094304));
#29376=CARTESIAN_POINT('Ctrl Pts',(0.230116418626786,0.114889649949471,
-0.942534136168517));
#29377=CARTESIAN_POINT('Ctrl Pts',(0.0288541519363172,0.255579020471033,
-0.934613681242733));
#29378=CARTESIAN_POINT('Ctrl Pts',(-0.198709267084557,0.163302862689978,
-0.926693226316945));
#29379=CARTESIAN_POINT('Ctrl Pts',(-0.245145106467147,-0.0778272096586138,
-0.918772771391161));
#29380=CARTESIAN_POINT('Ctrl Pts',(-0.0681261445426857,-0.248016181363272,
-0.910852316465374));
#29381=CARTESIAN_POINT('Ctrl Pts',(0.170991197855606,-0.192133308002639,
-0.902931861539589));
#29382=CARTESIAN_POINT('Ctrl Pts',(0.254246550215305,0.0388830231818767,
-0.895011406613802));
#29383=CARTESIAN_POINT('Ctrl Pts',(0.105750948292417,0.234456679843913,
-0.887090951688017));
#29384=CARTESIAN_POINT('Ctrl Pts',(-0.139138815762931,0.216318255670307,
-0.879170496762231));
#29385=CARTESIAN_POINT('Ctrl Pts',(-0.25720069049779,0.00100129696836331,
-0.871250041836445));
#29386=CARTESIAN_POINT('Ctrl Pts',(-0.140818851386615,-0.215228364492966,
-0.86332958691066));
#29387=CARTESIAN_POINT('Ctrl Pts',(0.103922264034112,-0.235272949626989,
-0.855409131984872));
#29388=CARTESIAN_POINT('Ctrl Pts',(0.25393610059609,-0.0408614072470928,
-0.847488677059087));
#29389=CARTESIAN_POINT('Ctrl Pts',(0.172481964081841,0.1907961473789,-0.839568222133301));
#29390=CARTESIAN_POINT('Ctrl Pts',(-0.0661930265154354,0.248539093562536,
-0.831647767207517));
#29391=CARTESIAN_POINT('Ctrl Pts',(-0.244531713438901,0.0797335494681849,
-0.823727312281729));
#29392=CARTESIAN_POINT('Ctrl Pts',(-0.19997471940289,-0.161750763175621,
-0.815806857355944));
#29393=CARTESIAN_POINT('Ctrl Pts',(0.026863340058709,-0.25579593184617,
-0.807886402430158));
#29394=CARTESIAN_POINT('Ctrl Pts',(0.229214913121365,-0.116677853043863,
-0.799965947504372));
#29395=CARTESIAN_POINT('Ctrl Pts',(0.222632383413667,0.128794486076502,
-0.792045492578587));
#29396=CARTESIAN_POINT('Ctrl Pts',(0.0131158620091436,0.256868004920654,
-0.7841250376528));
#29397=CARTESIAN_POINT('Ctrl Pts',(-0.208356037095823,0.150801059657697,
-0.776204582727015));
#29398=CARTESIAN_POINT('Ctrl Pts',(-0.239907127495152,-0.0927241498488127,
-0.768284127801228));
#29399=CARTESIAN_POINT('Ctrl Pts',(-0.0527779420396886,-0.251729391653449,
-0.760363672875443));
#29400=CARTESIAN_POINT('Ctrl Pts',(0.182459421962995,-0.181278120922218,
-0.752443217949657));
#29401=CARTESIAN_POINT('Ctrl Pts',(0.251381274026667,0.0544118815782901,
-0.744522763023871));
#29402=CARTESIAN_POINT('Ctrl Pts',(0.0911639299237252,0.240504336071146,
-0.736602308098085));
#29403=CARTESIAN_POINT('Ctrl Pts',(-0.152151209363023,0.207372146821915,
-0.7286818531723));
#29404=CARTESIAN_POINT('Ctrl Pts',(-0.256777395209575,-0.0147840149332312,
-0.720761398246514));
#29405=CARTESIAN_POINT('Ctrl Pts',(-0.127345709562336,-0.223464243323681,
-0.712840943320728));
#29406=CARTESIAN_POINT('Ctrl Pts',(0.118164206801822,-0.228452222617896,
-0.704920488394942));
#29407=CARTESIAN_POINT('Ctrl Pts',(0.255965020858851,-0.0252013072059438,
-0.697000033469156));
#29408=CARTESIAN_POINT('Ctrl Pts',(0.160448459333854,0.201021117511452,
-0.68907957854337));
#29409=CARTESIAN_POINT('Ctrl Pts',(-0.0813201694554329,0.244008663427961,
-0.681159123617584));
#29410=CARTESIAN_POINT('Ctrl Pts',(-0.248963792978122,0.0645772992165747,
-0.673238668691798));
#29411=CARTESIAN_POINT('Ctrl Pts',(-0.189671803979623,-0.173717600038902,
-0.665318213766012));
#29412=CARTESIAN_POINT('Ctrl Pts',(0.0425099313519794,-0.253665337649058,
-0.657397758840227));
#29413=CARTESIAN_POINT('Ctrl Pts',(0.235942990845232,-0.102391908172312,
-0.64947730391444));
#29414=CARTESIAN_POINT('Ctrl Pts',(0.21430916648743,0.142213849352388,-0.641556848988655));
#29415=CARTESIAN_POINT('Ctrl Pts',(-0.00267186632973278,0.257188761260045,
-0.633636394062868));
#29416=CARTESIAN_POINT('Ctrl Pts',(-0.217217438091055,0.137730833066962,
-0.625715939137084));
#29417=CARTESIAN_POINT('Ctrl Pts',(-0.233764852072829,-0.107271579290737,
-0.617795484211297));
#29418=CARTESIAN_POINT('Ctrl Pts',(-0.0372308004467332,-0.254493743118089,
-0.609875029285512));
#29419=CARTESIAN_POINT('Ctrl Pts',(0.193239890732311,-0.169739631253061,
-0.601954574359726));
#29420=CARTESIAN_POINT('Ctrl Pts',(0.247568451193101,0.0697356419774633,
-0.594034119433939));
#29421=CARTESIAN_POINT('Ctrl Pts',(0.0762332818385088,0.245645444753797,
-0.586113664508155));
#29422=CARTESIAN_POINT('Ctrl Pts',(-0.164590090204428,0.197644377594352,
-0.578193209582367));
#29423=CARTESIAN_POINT('Ctrl Pts',(-0.255386213350406,-0.0305136005528887,
-0.570272754656583));
#29424=CARTESIAN_POINT('Ctrl Pts',(-0.113392555850513,-0.230857804862319,
-0.562352299730795));
#29425=CARTESIAN_POINT('Ctrl Pts',(0.131960746075832,-0.220770376824587,
-0.554431844805011));
#29426=CARTESIAN_POINT('Ctrl Pts',(0.25702911668245,-0.00944621435284863,
-0.546511389879224));
#29427=CARTESIAN_POINT('Ctrl Pts',(0.14781016650087,0.21048836658387,-0.538590934953439));
#29428=CARTESIAN_POINT('Ctrl Pts',(-0.096140787360785,0.238558476675654,
-0.530670480027653));
#29429=CARTESIAN_POINT('Ctrl Pts',(-0.25245743823001,0.0491776338440616,
-0.522750025101866));
#29430=CARTESIAN_POINT('Ctrl Pts',(-0.178653947150355,-0.185029632642338,
-0.514829570176082));
#29431=CARTESIAN_POINT('Ctrl Pts',(0.0579962873891273,-0.250578587347838,
-0.506909115250295));
#29432=CARTESIAN_POINT('Ctrl Pts',(0.241781714379012,-0.087720011286514,
-0.49898866032451));
#29433=CARTESIAN_POINT('Ctrl Pts',(0.205178141054117,0.155097157361885,
-0.491068205398723));
#29434=CARTESIAN_POINT('Ctrl Pts',(-0.0184495234412028,0.256540080441542,
-0.483147750472938));
#29435=CARTESIAN_POINT('Ctrl Pts',(-0.225260068255102,0.12414144931435,
-0.475227295547152));
#29436=CARTESIAN_POINT('Ctrl Pts',(-0.226741432650673,-0.121414663478844,
-0.467306840621366));
#29437=CARTESIAN_POINT('Ctrl Pts',(-0.0215433225451699,-0.256298815919768,
-0.45938638569558));
#29438=CARTESIAN_POINT('Ctrl Pts',(0.203291968690357,-0.157561331722472,
-0.451465930769794));
#29439=CARTESIAN_POINT('Ctrl Pts',(0.242822453618414,0.0847965436022809,
-0.443545475844009));
#29440=CARTESIAN_POINT('Ctrl Pts',(0.0610152830318996,0.24986062719984,
-0.435625020918222));
#29441=CARTESIAN_POINT('Ctrl Pts',(-0.176408571661025,0.187171615456717,
-0.427704565992437));
#29442=CARTESIAN_POINT('Ctrl Pts',(-0.253032388786235,-0.0461281694118899,
-0.419784111066651));
#29443=CARTESIAN_POINT('Ctrl Pts',(-0.0990119847176032,-0.237381180110053,
-0.411863656140865));
#29444=CARTESIAN_POINT('Ctrl Pts',(0.145259877725951,-0.212256367893173,
-0.403943201215079));
#29445=CARTESIAN_POINT('Ctrl Pts',(0.25712437710612,0.00634448468750714,
-0.396022746289293));
#29446=CARTESIAN_POINT('Ctrl Pts',(0.134614723864691,0.219162209121448,
-0.388102291363507));
#29447=CARTESIAN_POINT('Ctrl Pts',(-0.11059901597976,0.232209077024282,
-0.380181836437722));
#29448=CARTESIAN_POINT('Ctrl Pts',(-0.254999480386151,0.033592600241025,
-0.372261381511935));
#29449=CARTESIAN_POINT('Ctrl Pts',(-0.166962679189424,-0.195644221857049,
-0.36434092658615));
#29450=CARTESIAN_POINT('Ctrl Pts',(0.0732640345114102,-0.246547316017172,
-0.356420471660364));
#29451=CARTESIAN_POINT('Ctrl Pts',(0.246709075468843,-0.0727174660550607,
-0.348500016734578));
#29452=CARTESIAN_POINT('Ctrl Pts',(0.195273725240327,0.167395848272668,
-0.340579561808792));
#29453=CARTESIAN_POINT('Ctrl Pts',(-0.0341576376477591,0.254924407577,-0.332659106883006));
#29454=CARTESIAN_POINT('Ctrl Pts',(-0.232453612015502,0.110084131686205,
-0.324738651957221));
#29455=CARTESIAN_POINT('Ctrl Pts',(-0.218863343028437,-0.135100092030241,
-0.316818197031434));
#29456=CARTESIAN_POINT('Ctrl Pts',(-0.00577464009454566,-0.257137806088364,
-0.308897742105649));
#29457=CARTESIAN_POINT('Ctrl Pts',(0.212577765931518,-0.144789126731672,
-0.300977287179862));
#29458=CARTESIAN_POINT('Ctrl Pts',(0.237161170678426,0.0995378164850663,
-0.293056832254077));
#29459=CARTESIAN_POINT('Ctrl Pts',(0.0455672956274394,0.253133994867042,
-0.285136377328291));
#29460=CARTESIAN_POINT('Ctrl Pts',(-0.187562105615528,0.175993336024981,
-0.277215922402505));
#29461=CARTESIAN_POINT('Ctrl Pts',(-0.249724793930603,-0.0615688645712112,
-0.269295467476719));
#29462=CARTESIAN_POINT('Ctrl Pts',(-0.084258201720026,-0.243009780113768,
-0.261375012550933));
#29463=CARTESIAN_POINT('Ctrl Pts',(0.158011472529912,-0.202942288192858,
-0.253454557625148));
#29464=CARTESIAN_POINT('Ctrl Pts',(0.256250443060382,0.0221112690783347,
-0.245534102699361));
#29465=CARTESIAN_POINT('Ctrl Pts',(0.120911869802921,0.227009950283883,
-0.237613647773576));
#29466=CARTESIAN_POINT('Ctrl Pts',(-0.124640357031449,0.224984397651718,
-0.22969319284779));
#29467=CARTESIAN_POINT('Ctrl Pts',(-0.256580337582835,0.0178809440144413,
-0.221772737922004));
#29468=CARTESIAN_POINT('Ctrl Pts',(-0.154642068682266,-0.205521357463858,
-0.213852282996218));
#29469=CARTESIAN_POINT('Ctrl Pts',(0.0882556230412838,-0.241586718983118,
-0.205931828070432));
#29470=CARTESIAN_POINT('Ctrl Pts',(0.250706501180205,-0.0574408224581984,
-0.198011373144647));
#29471=CARTESIAN_POINT('Ctrl Pts',(0.184633252234903,0.179063563844805,
-0.190090918218861));
#29472=CARTESIAN_POINT('Ctrl Pts',(-0.0497369991668516,0.252347832796275,
-0.182170463293075));
#29473=CARTESIAN_POINT('Ctrl Pts',(-0.23877095476344,0.0956118671352282,
-0.174250008367289));
#29474=CARTESIAN_POINT('Ctrl Pts',(-0.210160277709292,-0.148276279355404,
-0.166329553441503));
#29475=CARTESIAN_POINT('Ctrl Pts',(0.0100158074287402,-0.257007551691304,
-0.158409098515717));
#29476=CARTESIAN_POINT('Ctrl Pts',(0.221062284030839,-0.131471158330418,
-0.150488643589931));
#29477=CARTESIAN_POINT('Ctrl Pts',(0.230605935914093,0.113903893563196,
-0.142568188664146));
#29478=CARTESIAN_POINT('Ctrl Pts',(0.0299475598214531,0.255453212845186,
-0.13464773373836));
#29479=CARTESIAN_POINT('Ctrl Pts',(-0.198008671586209,0.164151667438431,
-0.126727278812574));
#29480=CARTESIAN_POINT('Ctrl Pts',(-0.245475856005881,-0.0767774715160755,
-0.118806823886788));
#29481=CARTESIAN_POINT('Ctrl Pts',(-0.0691868957427056,-0.24772241328998,
-0.110886368961002));
#29482=CARTESIAN_POINT('Ctrl Pts',(0.170167610585507,-0.192863199035107,
-0.102965914035216));
#29483=CARTESIAN_POINT('Ctrl Pts',(0.254410332361144,0.0377946191841849,
-0.0950454591094304));
#29484=CARTESIAN_POINT('Ctrl Pts',(0.106753780372761,0.234002178088288,
-0.0871250041836445));
#29485=CARTESIAN_POINT('Ctrl Pts',(-0.138212881221763,0.216911349922406,
-0.0792045492578586));
#29486=CARTESIAN_POINT('Ctrl Pts',(-0.257192155654031,0.00210249804848441,
-0.0712840943320729));
#29487=CARTESIAN_POINT('Ctrl Pts',(-0.141742157498023,-0.214624967918095,
-0.063363639406287));
#29488=CARTESIAN_POINT('Ctrl Pts',(0.102921386109171,-0.235713292600032,
-0.055443184480501));
#29489=CARTESIAN_POINT('Ctrl Pts',(0.253745924148315,-0.0419518472751756,
-0.0475227295547153));
#29490=CARTESIAN_POINT('Ctrl Pts',(0.173321533153074,0.190064273543398,
-0.0396022746289292));
#29491=CARTESIAN_POINT('Ctrl Pts',(-0.0651758599354944,0.248804958958394,
-0.0316818197031436));
#29492=CARTESIAN_POINT('Ctrl Pts',(-0.244098679855147,0.0808079646592843,
-0.0237613647773576));
#29493=CARTESIAN_POINT('Ctrl Pts',(-0.200838287407273,-0.160948635674951,
-0.0158409098515717));
#29494=CARTESIAN_POINT('Ctrl Pts',(0.0261231005236458,-0.255800095598605,
-0.00792045492578602));
#29495=CARTESIAN_POINT('Ctrl Pts',(0.160601584503721,-0.163869943260562,
-0.0026401516419286));
#29496=CARTESIAN_POINT('Ctrl Pts',(0.193653104151514,-0.0996214127458699,
0.));
#29497=CARTESIAN_POINT('Ctrl Pts',(-0.0986179012119374,0.204792088618073,
-1.17464852262806));
#29498=CARTESIAN_POINT('Ctrl Pts',(-0.16656202641662,0.172073505236353,
-1.17200837098613));
#29499=CARTESIAN_POINT('Ctrl Pts',(-0.266177295204196,0.0342896334034012,
-1.16672806770228));
#29500=CARTESIAN_POINT('Ctrl Pts',(-0.173452084178045,-0.205124351144866,
-1.15880761277649));
#29501=CARTESIAN_POINT('Ctrl Pts',(0.0776013675721355,-0.256908479144051,
-1.1508871578507));
#29502=CARTESIAN_POINT('Ctrl Pts',(0.257804953624139,-0.0748439916648578,
-1.14296670292492));
#29503=CARTESIAN_POINT('Ctrl Pts',(0.203074034265681,0.175613484186487,
-1.13504624799913));
#29504=CARTESIAN_POINT('Ctrl Pts',(-0.036794585207094,0.265905798100996,
-1.12712579307335));
#29505=CARTESIAN_POINT('Ctrl Pts',(-0.243107585293851,0.113866785733275,
-1.11920533814756));
#29506=CARTESIAN_POINT('Ctrl Pts',(-0.22783176255635,-0.141989019123882,
-1.11128488322178));
#29507=CARTESIAN_POINT('Ctrl Pts',(-0.00487800918614132,-0.268405822095947,
-1.10336442829599));
#29508=CARTESIAN_POINT('Ctrl Pts',(0.22251972969843,-0.150172095122027,
-1.09544397337021));
#29509=CARTESIAN_POINT('Ctrl Pts',(0.247087436830596,0.10495020925552,-1.08752351844442));
#29510=CARTESIAN_POINT('Ctrl Pts',(0.0464291981955566,0.264406332440427,
-1.07960306351863));
#29511=CARTESIAN_POINT('Ctrl Pts',(-0.196549855663804,0.182851655946659,
-1.07168260859285));
#29512=CARTESIAN_POINT('Ctrl Pts',(-0.260369863488897,-0.0653765907044025,
-1.06376215366706));
#29513=CARTESIAN_POINT('Ctrl Pts',(-0.0868572934190015,-0.254012453329219,
-1.05584169874127));
#29514=CARTESIAN_POINT('Ctrl Pts',(0.165827432725362,-0.211110892307444,
-1.04792124381549));
#29515=CARTESIAN_POINT('Ctrl Pts',(0.267357073922758,0.0242226616622236,
-1.0400007888897));
#29516=CARTESIAN_POINT('Ctrl Pts',(0.125185234855463,0.237476721258427,
-1.03208033396392));
#29517=CARTESIAN_POINT('Ctrl Pts',(-0.131095510342261,0.234265891582874,
-1.02415987903813));
#29518=CARTESIAN_POINT('Ctrl Pts',(-0.267880008317113,0.0175168772476024,
-1.01623942411235));
#29519=CARTESIAN_POINT('Ctrl Pts',(-0.160486372757608,-0.21519912468331,
-1.00831896918656));
#29520=CARTESIAN_POINT('Ctrl Pts',(0.0931938878370631,-0.251756706089098,
-1.00039851426077));
#29521=CARTESIAN_POINT('Ctrl Pts',(0.26192600547804,-0.0588328756502444,
-0.992478059334988));
#29522=CARTESIAN_POINT('Ctrl Pts',(0.19190718727891,0.187718328863886,-0.984557604409201));
#29523=CARTESIAN_POINT('Ctrl Pts',(-0.0530389748994192,0.263160420203277,
-0.976637149483416));
#29524=CARTESIAN_POINT('Ctrl Pts',(-0.249639021799637,0.098726381382141,
-0.96871669455763));
#29525=CARTESIAN_POINT('Ctrl Pts',(-0.218687971190389,-0.155698782379805,
-0.960796239631844));
#29526=CARTESIAN_POINT('Ctrl Pts',(0.0116016583088355,-0.268201307074383,
-0.952875784706058));
#29527=CARTESIAN_POINT('Ctrl Pts',(0.231316137903588,-0.136232829859319,
-0.944955329780272));
#29528=CARTESIAN_POINT('Ctrl Pts',(0.240181205160686,0.119914670800206,
-0.937034874854487));
#29529=CARTESIAN_POINT('Ctrl Pts',(0.0301161691430373,0.266757485262614,
-0.9291144199287));
#29530=CARTESIAN_POINT('Ctrl Pts',(-0.207400373818482,0.170445371091411,
-0.921193965002915));
#29531=CARTESIAN_POINT('Ctrl Pts',(-0.255867214785822,-0.0812312008054323,
-0.913273510077128));
#29532=CARTESIAN_POINT('Ctrl Pts',(-0.0711058324167257,-0.258863864189515,
-0.905353055151343));
#29533=CARTESIAN_POINT('Ctrl Pts',(0.178469977144206,-0.200536796735162,
-0.897432600225557));
#29534=CARTESIAN_POINT('Ctrl Pts',(0.265366735685634,0.040583681181222,
-0.889512145299772));
#29535=CARTESIAN_POINT('Ctrl Pts',(0.110376262412427,0.244711299866933,
-0.881591690373985));
#29536=CARTESIAN_POINT('Ctrl Pts',(-0.145224441845548,0.225779540874117,
-0.8736712354482));
#29537=CARTESIAN_POINT('Ctrl Pts',(-0.268450083573173,0.00104509149768783,
-0.865750780522413));
#29538=CARTESIAN_POINT('Ctrl Pts',(-0.146977958536001,-0.224641980251412,
-0.857830325596628));
#29539=CARTESIAN_POINT('Ctrl Pts',(0.108467595522689,-0.245563271496795,
-0.849909870670841));
#29540=CARTESIAN_POINT('Ctrl Pts',(0.265042707682201,-0.0426485954185014,
-0.841989415745057));
#29541=CARTESIAN_POINT('Ctrl Pts',(0.180025946209632,0.199141151643779,
-0.834068960819269));
#29542=CARTESIAN_POINT('Ctrl Pts',(-0.069088164054453,0.259409647419421,
-0.826148505893485));
#29543=CARTESIAN_POINT('Ctrl Pts',(-0.255226993294282,0.0832209197296219,
-0.818228050967699));
#29544=CARTESIAN_POINT('Ctrl Pts',(-0.208721174240739,-0.168825386154603,
-0.810307596041912));
#29545=CARTESIAN_POINT('Ctrl Pts',(0.0280382835281578,-0.266983883864697,
-0.802387141116127));
#29546=CARTESIAN_POINT('Ctrl Pts',(0.239240269785266,-0.121781085968867,
-0.79446668619034));
#29547=CARTESIAN_POINT('Ctrl Pts',(0.232369834691432,0.134427673907422,
-0.786546231264555));
#29548=CARTESIAN_POINT('Ctrl Pts',(0.0136895209949644,0.268102847059877,
-0.77862577633877));
#29549=CARTESIAN_POINT('Ctrl Pts',(-0.217469072353946,0.157396766663733,
-0.770705321412982));
#29550=CARTESIAN_POINT('Ctrl Pts',(-0.250400138122595,-0.0967797004276667,
-0.762784866487198));
#29551=CARTESIAN_POINT('Ctrl Pts',(-0.0550863332596542,-0.262739482139038,
-0.754864411561411));
#29552=CARTESIAN_POINT('Ctrl Pts',(0.190439796175818,-0.189206827623098,
-0.746943956635626));
#29553=CARTESIAN_POINT('Ctrl Pts',(0.262376138612152,0.0567917377235466,
-0.739023501709839));
#29554=CARTESIAN_POINT('Ctrl Pts',(0.0951512399112054,0.251023467289502,
-0.731103046784055));
#29555=CARTESIAN_POINT('Ctrl Pts',(-0.158805968950592,0.216442148881283,
-0.723182591858267));
#29556=CARTESIAN_POINT('Ctrl Pts',(-0.268008274279125,-0.0154306352626495,
-0.715262136932482));
#29557=CARTESIAN_POINT('Ctrl Pts',(-0.132915531091811,-0.233238078326128,
-0.707341682006696));
#29558=CARTESIAN_POINT('Ctrl Pts',(0.123332449574351,-0.238444220874975,
-0.699421227080911));
#29559=CARTESIAN_POINT('Ctrl Pts',(0.267160368459267,-0.0263035570102677,
-0.691500772155124));
#29560=CARTESIAN_POINT('Ctrl Pts',(0.167466122404248,0.2098133395034,-0.68358031722934));
#29561=CARTESIAN_POINT('Ctrl Pts',(-0.0848769349889562,0.25468106622512,
-0.675659862303552));
#29562=CARTESIAN_POINT('Ctrl Pts',(-0.259852922254286,0.0674017683936514,
-0.667739407377768));
#29563=CARTESIAN_POINT('Ctrl Pts',(-0.197967631934649,-0.181315626168488,
-0.659818952451982));
#29564=CARTESIAN_POINT('Ctrl Pts',(0.0443692223455626,-0.264760102158791,
-0.651898497526195));
#29565=CARTESIAN_POINT('Ctrl Pts',(0.246262618845695,-0.106870305258026,
-0.64397804260041));
#29566=CARTESIAN_POINT('Ctrl Pts',(0.223682578544795,0.148433970647676,
-0.636057587674623));
#29567=CARTESIAN_POINT('Ctrl Pts',(-0.00278872789231205,0.26843763257678,
-0.628137132748838));
#29568=CARTESIAN_POINT('Ctrl Pts',(-0.226718051558245,0.143754877080107,
-0.620216677823052));
#29569=CARTESIAN_POINT('Ctrl Pts',(-0.243989213069241,-0.111963402469451,
-0.612296222897266));
#29570=CARTESIAN_POINT('Ctrl Pts',(-0.0388591938539432,-0.265624740262848,
-0.60437576797148));
#29571=CARTESIAN_POINT('Ctrl Pts',(0.201691778962022,-0.177163669768434,
-0.596455313045694));
#29572=CARTESIAN_POINT('Ctrl Pts',(0.258396551285464,0.0727857257328775,
-0.588534858119908));
#29573=CARTESIAN_POINT('Ctrl Pts',(0.0795675580846886,0.256389436769777,
-0.580614403194122));
#29574=CARTESIAN_POINT('Ctrl Pts',(-0.171788899109018,0.206288908401773,
-0.572693948268337));
#29575=CARTESIAN_POINT('Ctrl Pts',(-0.266556245182171,-0.0318481983959204,
-0.564773493342551));
#29576=CARTESIAN_POINT('Ctrl Pts',(-0.118352097094806,-0.240955018001172,
-0.556853038416764));
#29577=CARTESIAN_POINT('Ctrl Pts',(0.137732419162147,-0.230426388025387,
-0.54893258349098));
#29578=CARTESIAN_POINT('Ctrl Pts',(0.268271005496135,-0.00985937101321311,
-0.541012128565193));
#29579=CARTESIAN_POINT('Ctrl Pts',(0.154275058411882,0.219694665248599,
-0.533091673639407));
#29580=CARTESIAN_POINT('Ctrl Pts',(-0.100345774157302,0.248992500279537,
-0.525171218713622));
#29581=CARTESIAN_POINT('Ctrl Pts',(-0.263499371873178,0.0513285554942264,
-0.517250763787835));
#29582=CARTESIAN_POINT('Ctrl Pts',(-0.186467878256346,-0.193122422222952,
-0.509330308862051));
#29583=CARTESIAN_POINT('Ctrl Pts',(0.0605329175688147,-0.261538344181672,
-0.501409853936263));
#29584=CARTESIAN_POINT('Ctrl Pts',(0.252356715317872,-0.0915566918398557,
-0.493489399010479));
#29585=CARTESIAN_POINT('Ctrl Pts',(0.214152182121918,0.161880766242023,
-0.485568944084692));
#29586=CARTESIAN_POINT('Ctrl Pts',(-0.0192564650588239,0.267760579884571,
-0.477648489158906));
#29587=CARTESIAN_POINT('Ctrl Pts',(-0.235112448694224,0.129571123541048,
-0.469728034233121));
#29588=CARTESIAN_POINT('Ctrl Pts',(-0.23665860471357,-0.126725074084451,
-0.461807579307334));
#29589=CARTESIAN_POINT('Ctrl Pts',(-0.0224855801378355,-0.267508762982727,
-0.453887124381549));
#29590=CARTESIAN_POINT('Ctrl Pts',(0.212183512723307,-0.164452718174804,
-0.445966669455763));
#29591=CARTESIAN_POINT('Ctrl Pts',(0.25344297420487,0.0885053581026219,
-0.438046214529977));
#29592=CARTESIAN_POINT('Ctrl Pts',(0.0636839574475984,0.260788982034319,
-0.430125759604191));
#29593=CARTESIAN_POINT('Ctrl Pts',(-0.184124294976701,0.195358090659221,
-0.422205304678405));
#29594=CARTESIAN_POINT('Ctrl Pts',(-0.264099469503438,-0.0481457141881418,
-0.41428484975262));
#29595=CARTESIAN_POINT('Ctrl Pts',(-0.103342551377849,-0.247763711348939,
-0.406364394826833));
#29596=CARTESIAN_POINT('Ctrl Pts',(0.151613225609499,-0.22153999505048,
-0.398443939901048));
#29597=CARTESIAN_POINT('Ctrl Pts',(0.268370432401429,0.00662197850749817,
-0.390523484975262));
#29598=CARTESIAN_POINT('Ctrl Pts',(0.140502476108113,0.228747882600414,
-0.382603030049476));
#29599=CARTESIAN_POINT('Ctrl Pts',(-0.115436373928134,0.242365391838454,
-0.37468257512369));
#29600=CARTESIAN_POINT('Ctrl Pts',(-0.266152597367798,0.0350618667651702,
-0.366762120197904));
#29601=CARTESIAN_POINT('Ctrl Pts',(-0.174265259923113,-0.204201270247307,
-0.358841665272119));
#29602=CARTESIAN_POINT('Ctrl Pts',(0.0764684424035977,-0.2573307539006,
-0.350921210346332));
#29603=CARTESIAN_POINT('Ctrl Pts',(0.257499588355266,-0.0758979682438996,
-0.343000755420547));
#29604=CARTESIAN_POINT('Ctrl Pts',(0.203814568922633,0.17471737487029,-0.335080300494761));
#29605=CARTESIAN_POINT('Ctrl Pts',(-0.0356516176665625,0.266074241038927,
-0.327159845568975));
#29606=CARTESIAN_POINT('Ctrl Pts',(-0.242620622252893,0.114898969726894,
-0.319239390643189));
#29607=CARTESIAN_POINT('Ctrl Pts',(-0.228435944761169,-0.141009073210762,
-0.311318935717403));
#29608=CARTESIAN_POINT('Ctrl Pts',(-0.0060272101641153,-0.268384448737849,
-0.303398480791617));
#29609=CARTESIAN_POINT('Ctrl Pts',(0.221875450332839,-0.151121885001074,
-0.295478025865832));
#29610=CARTESIAN_POINT('Ctrl Pts',(0.247534079188182,0.103891381871452,
-0.287557570940045));
#29611=CARTESIAN_POINT('Ctrl Pts',(0.0475603090167235,0.264205519610968,
-0.27963711601426));
#29612=CARTESIAN_POINT('Ctrl Pts',(-0.195765659999584,0.183690897846301,
-0.271716661088473));
#29613=CARTESIAN_POINT('Ctrl Pts',(-0.26064720771634,-0.0642617514270981,
-0.263796206162689));
#29614=CARTESIAN_POINT('Ctrl Pts',(-0.0879434703292936,-0.253638493949533,
-0.255875751236902));
#29615=CARTESIAN_POINT('Ctrl Pts',(0.164922547152102,-0.211818537969172,
-0.247955296311117));
#29616=CARTESIAN_POINT('Ctrl Pts',(0.267458274400757,0.0230783674044562,
-0.24003484138533));
#29617=CARTESIAN_POINT('Ctrl Pts',(0.126200289317892,0.236938866718065,
-0.232114386459545));
#29618=CARTESIAN_POINT('Ctrl Pts',(-0.130091852385482,0.234824720864357,
-0.224193931533758));
#29619=CARTESIAN_POINT('Ctrl Pts',(-0.267802597784771,0.0186630172172313,
-0.216273476607973));
#29620=CARTESIAN_POINT('Ctrl Pts',(-0.161405772983488,-0.214510410063299,
-0.208353021682187));
#29621=CARTESIAN_POINT('Ctrl Pts',(0.0921157300759217,-0.252153191251809,
-0.200432566756401));
#29622=CARTESIAN_POINT('Ctrl Pts',(0.261671852684011,-0.0599531578222869,
-0.192512111830615));
#29623=CARTESIAN_POINT('Ctrl Pts',(0.192708705007432,0.186895410684992,
-0.18459165690483));
#29624=CARTESIAN_POINT('Ctrl Pts',(-0.051912386227186,0.263384972538599,
-0.176671201979044));
#29625=CARTESIAN_POINT('Ctrl Pts',(-0.249214271692021,0.0997937201232344,
-0.168750747053258));
#29626=CARTESIAN_POINT('Ctrl Pts',(-0.219352226487531,-0.154761558018521,
-0.160830292127472));
#29627=CARTESIAN_POINT('Ctrl Pts',(0.0104538768387219,-0.268248497299659,
-0.152909837201686));
#29628=CARTESIAN_POINT('Ctrl Pts',(0.230731062611456,-0.137221417924482,
-0.1449893822759));
#29629=CARTESIAN_POINT('Ctrl Pts',(0.240692132858562,0.11888579959552,-0.137068927350114));
#29630=CARTESIAN_POINT('Ctrl Pts',(0.0312574002866088,0.26662617508764,
-0.129148472424328));
#29631=CARTESIAN_POINT('Ctrl Pts',(-0.2066691358124,0.171331300694549,-0.121228017498543));
#29632=CARTESIAN_POINT('Ctrl Pts',(-0.25621243058265,-0.0801355494230467,
-0.113307562572757));
#29633=CARTESIAN_POINT('Ctrl Pts',(-0.0722129785435288,-0.258557247346171,
-0.105387107646971));
#29634=CARTESIAN_POINT('Ctrl Pts',(0.177610367976516,-0.201298611597657,
-0.097466652721185));
#29635=CARTESIAN_POINT('Ctrl Pts',(0.265537681302665,0.0394476727841362,
-0.0895461977953991));
#29636=CARTESIAN_POINT('Ctrl Pts',(0.111422956164521,0.244236919203158,
-0.0816257428696134));
#29637=CARTESIAN_POINT('Ctrl Pts',(-0.144258008962033,0.226398575765643,
-0.0737052879438273));
#29638=CARTESIAN_POINT('Ctrl Pts',(-0.2684411754341,0.00219445669347009,
-0.0657848330180417));
#29639=CARTESIAN_POINT('Ctrl Pts',(-0.147941648028013,-0.224012192436151,
-0.0578643780922557));
#29640=CARTESIAN_POINT('Ctrl Pts',(0.107422941396463,-0.246022874103948,
-0.0499439231664699));
#29641=CARTESIAN_POINT('Ctrl Pts',(0.264844213334459,-0.0437867288974735,
-0.042023468240684));
#29642=CARTESIAN_POINT('Ctrl Pts',(0.180902236187321,0.198377267254801,
-0.034103013314898));
#29643=CARTESIAN_POINT('Ctrl Pts',(-0.068026508843246,0.259687141183529,
-0.0261825583891124));
#29644=CARTESIAN_POINT('Ctrl Pts',(-0.254775019773046,0.0843423274804512,
-0.0182621034633263));
#29645=CARTESIAN_POINT('Ctrl Pts',(-0.209622512812183,-0.167988175359505,
-0.0103416485375405));
#29646=CARTESIAN_POINT('Ctrl Pts',(0.0272656675423015,-0.266988229730515,
-0.00242119361175477));
#29647=CARTESIAN_POINT('Ctrl Pts',(0.167625944932595,-0.171037254520151,
0.00285910967210262));
#29648=CARTESIAN_POINT('Ctrl Pts',(0.202123065428259,-0.103978634449024,
0.00549926131403122));
#29649=CARTESIAN_POINT('Ctrl Pts',(-0.10275048154209,0.213373895235262,
-1.16914926131403));
#29650=CARTESIAN_POINT('Ctrl Pts',(-0.173541803370507,0.179284240552571,
-1.1665091096721));
#29651=CARTESIAN_POINT('Ctrl Pts',(-0.277331447147971,0.0357265395106049,
-1.16122880638825));
#29652=CARTESIAN_POINT('Ctrl Pts',(-0.180720588805392,-0.21372008121374,
-1.15330835146246));
#29653=CARTESIAN_POINT('Ctrl Pts',(0.0808532506611131,-0.267674221615882,
-1.14538789653667));
#29654=CARTESIAN_POINT('Ctrl Pts',(0.268608262833421,-0.0779803269952925,
-1.13746744161088));
#29655=CARTESIAN_POINT('Ctrl Pts',(0.211583845864364,0.182972562219379,
-1.1295469866851));
#29656=CARTESIAN_POINT('Ctrl Pts',(-0.0383364612479987,0.277048572966425,
-1.12162653175931));
#29657=CARTESIAN_POINT('Ctrl Pts',(-0.253295001703547,0.118638370133228,
-1.11370607683353));
#29658=CARTESIAN_POINT('Ctrl Pts',(-0.237379046051068,-0.14793906490987,
-1.10578562190774));
#29659=CARTESIAN_POINT('Ctrl Pts',(-0.0050824220215922,-0.279653360395392,
-1.09786516698196));
#29660=CARTESIAN_POINT('Ctrl Pts',(0.231844412608142,-0.156465052473709,
-1.08994471205617));
#29661=CARTESIAN_POINT('Ctrl Pts',(0.257441628805129,0.109348144773157,
-1.08202425713039));
#29662=CARTESIAN_POINT('Ctrl Pts',(0.0483748124182258,0.275486272240229,
-1.0741038022046));
#29663=CARTESIAN_POINT('Ctrl Pts',(-0.204786271744744,0.190514049360174,
-1.06618334727882));
#29664=CARTESIAN_POINT('Ctrl Pts',(-0.271280655172714,-0.0681161948683243,
-1.05826289235303));
#29665=CARTESIAN_POINT('Ctrl Pts',(-0.0904970458159042,-0.264656837922096,
-1.05034243742724));
#29666=CARTESIAN_POINT('Ctrl Pts',(0.172776426551623,-0.21995748821254,
-1.04242198250146));
#29667=CARTESIAN_POINT('Ctrl Pts',(0.278560664459996,0.0252377116064939,
-1.03450152757567));
#29668=CARTESIAN_POINT('Ctrl Pts',(0.130431118542213,0.247428176471743,
-1.02658107264989));
#29669=CARTESIAN_POINT('Ctrl Pts',(-0.136589063954272,0.244082797070454,
-1.0186606177241));
#29670=CARTESIAN_POINT('Ctrl Pts',(-0.279105512405193,0.0182509214877408,
-1.01074016279831));
#29671=CARTESIAN_POINT('Ctrl Pts',(-0.167211549618656,-0.224217037849208,
-1.00281970787253));
#29672=CARTESIAN_POINT('Ctrl Pts',(0.09709917504185,-0.262306563658383,
-0.994899252946742));
#29673=CARTESIAN_POINT('Ctrl Pts',(0.272902007247412,-0.0612982656219496,
-0.986978798020957));
#29674=CARTESIAN_POINT('Ctrl Pts',(0.199949052473945,0.195584660066828,
-0.97905834309517));
#29675=CARTESIAN_POINT('Ctrl Pts',(-0.0552615716258469,0.27418815008641,
-0.971137888169384));
#29676=CARTESIAN_POINT('Ctrl Pts',(-0.260100137869332,0.102863507570724,
-0.963217433243599));
#29677=CARTESIAN_POINT('Ctrl Pts',(-0.227852084369397,-0.16222333540298,
-0.955296978317811));
#29678=CARTESIAN_POINT('Ctrl Pts',(0.0120878254684999,-0.279440275177697,
-0.947376523392029));
#29679=CARTESIAN_POINT('Ctrl Pts',(0.241009434047589,-0.141941662698782,
-0.93945606846624));
#29680=CARTESIAN_POINT('Ctrl Pts',(0.250245991694586,0.12493969165094,-0.931535613540455));
#29681=CARTESIAN_POINT('Ctrl Pts',(0.0313781863497569,0.277935950054195,
-0.92361515861467));
#29682=CARTESIAN_POINT('Ctrl Pts',(-0.216091480552406,0.177587879492844,
-0.915694703688883));
#29683=CARTESIAN_POINT('Ctrl Pts',(-0.266589323104498,-0.0846351919522501,
-0.907774248763098));
#29684=CARTESIAN_POINT('Ctrl Pts',(-0.0740855202907657,-0.269711547015759,
-0.899853793837311));
#29685=CARTESIAN_POINT('Ctrl Pts',(0.185948756432805,-0.208940285467685,
-0.891933338911526));
#29686=CARTESIAN_POINT('Ctrl Pts',(0.276486921155962,0.0422843391805672,
-0.884012883985739));
#29687=CARTESIAN_POINT('Ctrl Pts',(0.115001576532437,0.254965919889953,
-0.876092429059954));
#29688=CARTESIAN_POINT('Ctrl Pts',(-0.151310067928165,0.235240826077927,
-0.868171974134168));
#29689=CARTESIAN_POINT('Ctrl Pts',(-0.279699476648555,0.00108888602701205,
-0.860251519208383));
#29690=CARTESIAN_POINT('Ctrl Pts',(-0.153137065685387,-0.234055596009857,
-0.852331064282597));
#29691=CARTESIAN_POINT('Ctrl Pts',(0.113012927011266,-0.255853593366601,
-0.84441060935681));
#29692=CARTESIAN_POINT('Ctrl Pts',(0.276149314768311,-0.0444357835899101,
-0.836490154431025));
#29693=CARTESIAN_POINT('Ctrl Pts',(0.187569928337422,0.207486155908658,
-0.828569699505239));
#29694=CARTESIAN_POINT('Ctrl Pts',(-0.0719833015934706,0.270280201276306,
-0.820649244579453));
#29695=CARTESIAN_POINT('Ctrl Pts',(-0.265922273149663,0.086708289991059,
-0.812728789653667));
#29696=CARTESIAN_POINT('Ctrl Pts',(-0.217467629078588,-0.175900009133585,
-0.804808334727882));
#29697=CARTESIAN_POINT('Ctrl Pts',(0.0292132269976068,-0.278171835883225,
-0.796887879802095));
#29698=CARTESIAN_POINT('Ctrl Pts',(0.249265626449167,-0.126884318893871,
-0.78896742487631));
#29699=CARTESIAN_POINT('Ctrl Pts',(0.242107285969196,0.140060861738342,
-0.781046969950524));
#29700=CARTESIAN_POINT('Ctrl Pts',(0.0142631799807849,0.279337689199099,
-0.773126515024737));
#29701=CARTESIAN_POINT('Ctrl Pts',(-0.226582107612069,0.16399247366977,
-0.765206060098952));
#29702=CARTESIAN_POINT('Ctrl Pts',(-0.260893148750037,-0.100835251006521,
-0.757285605173166));
#29703=CARTESIAN_POINT('Ctrl Pts',(-0.0573947244796198,-0.273749572624627,
-0.749365150247381));
#29704=CARTESIAN_POINT('Ctrl Pts',(0.198420170388641,-0.197135534323977,
-0.741444695321594));
#29705=CARTESIAN_POINT('Ctrl Pts',(0.273371003197638,0.0591715938688031,
-0.733524240395808));
#29706=CARTESIAN_POINT('Ctrl Pts',(0.0991385498986852,0.261542598507859,
-0.725603785470023));
#29707=CARTESIAN_POINT('Ctrl Pts',(-0.165460728538161,0.22551215094065,
-0.717683330544237));
#29708=CARTESIAN_POINT('Ctrl Pts',(-0.279239153348675,-0.0160772555920675,
-0.709762875618451));
#29709=CARTESIAN_POINT('Ctrl Pts',(-0.138485352621285,-0.243011913328576,
-0.701842420692666));
#29710=CARTESIAN_POINT('Ctrl Pts',(0.128500692346879,-0.248436219132054,
-0.693921965766879));
#29711=CARTESIAN_POINT('Ctrl Pts',(0.278355716059682,-0.0274058068145916,
-0.686001510841094));
#29712=CARTESIAN_POINT('Ctrl Pts',(0.174483785474641,0.218605561495349,
-0.678081055915307));
#29713=CARTESIAN_POINT('Ctrl Pts',(-0.0884337005224793,0.265353469022279,
-0.670160600989522));
#29714=CARTESIAN_POINT('Ctrl Pts',(-0.270742051530451,0.070226237570728,
-0.662240146063736));
#29715=CARTESIAN_POINT('Ctrl Pts',(-0.206263459889676,-0.188913652298074,
-0.65431969113795));
#29716=CARTESIAN_POINT('Ctrl Pts',(0.0462285133391461,-0.275854866668525,
-0.646399236212164));
#29717=CARTESIAN_POINT('Ctrl Pts',(0.256582246846158,-0.111348702343739,
-0.638478781286378));
#29718=CARTESIAN_POINT('Ctrl Pts',(0.23305599060216,0.154654091942965,-0.630558326360593));
#29719=CARTESIAN_POINT('Ctrl Pts',(-0.00290558945489154,0.279686503893515,
-0.622637871434806));
#29720=CARTESIAN_POINT('Ctrl Pts',(-0.236218665025435,0.149778921093253,
-0.614717416509021));
#29721=CARTESIAN_POINT('Ctrl Pts',(-0.254213574065653,-0.116655225648164,
-0.606796961583234));
#29722=CARTESIAN_POINT('Ctrl Pts',(-0.040487587261153,-0.276755737407606,
-0.59887650665745));
#29723=CARTESIAN_POINT('Ctrl Pts',(0.210143667191733,-0.184587708283807,
-0.590956051731662));
#29724=CARTESIAN_POINT('Ctrl Pts',(0.269224651377827,0.075835809488292,
-0.583035596805878));
#29725=CARTESIAN_POINT('Ctrl Pts',(0.0829018343308682,0.267133428785756,
-0.57511514188009));
#29726=CARTESIAN_POINT('Ctrl Pts',(-0.178987708013609,0.214933439209195,
-0.567194686954306));
#29727=CARTESIAN_POINT('Ctrl Pts',(-0.277726277013936,-0.0331827962389527,
-0.559274232028519));
#29728=CARTESIAN_POINT('Ctrl Pts',(-0.1233116383391,-0.251052231140024,
-0.551353777102734));
#29729=CARTESIAN_POINT('Ctrl Pts',(0.143504092248462,-0.240082399226187,
-0.543433322176948));
#29730=CARTESIAN_POINT('Ctrl Pts',(0.279512894309821,-0.0102725276735772,
-0.535512867251162));
#29731=CARTESIAN_POINT('Ctrl Pts',(0.160739950322895,0.228900963913328,
-0.527592412325376));
#29732=CARTESIAN_POINT('Ctrl Pts',(-0.104550760953819,0.25942652388342,
-0.51967195739959));
#29733=CARTESIAN_POINT('Ctrl Pts',(-0.274541305516346,0.0534794771443913,
-0.511751502473804));
#29734=CARTESIAN_POINT('Ctrl Pts',(-0.194281809362337,-0.201215211803566,
-0.503831047548019));
#29735=CARTESIAN_POINT('Ctrl Pts',(0.0630695477485025,-0.272498101015506,
-0.495910592622232));
#29736=CARTESIAN_POINT('Ctrl Pts',(0.262931716256731,-0.0953933723931974,
-0.487990137696447));
#29737=CARTESIAN_POINT('Ctrl Pts',(0.223126223189719,0.16866437512216,-0.480069682770661));
#29738=CARTESIAN_POINT('Ctrl Pts',(-0.0200634066764452,0.278981079327601,
-0.472149227844875));
#29739=CARTESIAN_POINT('Ctrl Pts',(-0.244964829133346,0.135000797767746,
-0.464228772919089));
#29740=CARTESIAN_POINT('Ctrl Pts',(-0.246575776776468,-0.132035484690058,
-0.456308317993303));
#29741=CARTESIAN_POINT('Ctrl Pts',(-0.0234278377305011,-0.278718710045685,
-0.448387863067518));
#29742=CARTESIAN_POINT('Ctrl Pts',(0.221075056756257,-0.171344104627135,
-0.440467408141731));
#29743=CARTESIAN_POINT('Ctrl Pts',(0.264063494791325,0.0922141726029629,
-0.432546953215946));
#29744=CARTESIAN_POINT('Ctrl Pts',(0.0663526318632972,0.271717336868797,
-0.42462649829016));
#29745=CARTESIAN_POINT('Ctrl Pts',(-0.191840018292377,0.203544565861725,
-0.416706043364374));
#29746=CARTESIAN_POINT('Ctrl Pts',(-0.275166550220641,-0.0501632589643939,
-0.408785588438588));
#29747=CARTESIAN_POINT('Ctrl Pts',(-0.107673118038096,-0.258146242587824,
-0.400865133512802));
#29748=CARTESIAN_POINT('Ctrl Pts',(0.157966573493047,-0.230823622207787,
-0.392944678587017));
#29749=CARTESIAN_POINT('Ctrl Pts',(0.279616487696737,0.00689947232748906,
-0.38502422366123));
#29750=CARTESIAN_POINT('Ctrl Pts',(0.146390228351534,0.23833355607938,-0.377103768735445));
#29751=CARTESIAN_POINT('Ctrl Pts',(-0.120273731876508,0.252521706652626,
-0.369183313809658));
#29752=CARTESIAN_POINT('Ctrl Pts',(-0.277305714349445,0.0365311332893155,
-0.361262858883874));
#29753=CARTESIAN_POINT('Ctrl Pts',(-0.181567840656802,-0.212758318637564,
-0.353342403958087));
#29754=CARTESIAN_POINT('Ctrl Pts',(0.0796728502957855,-0.268114191784028,
-0.345421949032302));
#29755=CARTESIAN_POINT('Ctrl Pts',(0.268290101241689,-0.0790784704327387,
-0.337501494106515));
#29756=CARTESIAN_POINT('Ctrl Pts',(0.212355412604938,0.182038901467912,
-0.32958103918073));
#29757=CARTESIAN_POINT('Ctrl Pts',(-0.0371455976853658,0.277224074500852,
-0.321660584254944));
#29758=CARTESIAN_POINT('Ctrl Pts',(-0.252787632490283,0.119713807767583,
-0.313740129329158));
#29759=CARTESIAN_POINT('Ctrl Pts',(-0.238008546493902,-0.146918054391284,
-0.305819674403372));
#29760=CARTESIAN_POINT('Ctrl Pts',(-0.0062797802336852,-0.279631091387335,
-0.297899219477586));
#29761=CARTESIAN_POINT('Ctrl Pts',(0.23117313473416,-0.157454643270477,
-0.2899787645518));
#29762=CARTESIAN_POINT('Ctrl Pts',(0.257906987697937,0.108244947257839,
-0.282058309626014));
#29763=CARTESIAN_POINT('Ctrl Pts',(0.0495533224060077,0.275277044354895,
-0.274137854700229));
#29764=CARTESIAN_POINT('Ctrl Pts',(-0.203969214383641,0.191388459667621,
-0.266217399774442));
#29765=CARTESIAN_POINT('Ctrl Pts',(-0.271569621502078,-0.0669546382829851,
-0.258296944848657));
#29766=CARTESIAN_POINT('Ctrl Pts',(-0.0916287389385613,-0.264267207785298,
-0.250376489922871));
#29767=CARTESIAN_POINT('Ctrl Pts',(0.171833621774292,-0.220694787745487,
-0.242456034997085));
#29768=CARTESIAN_POINT('Ctrl Pts',(0.278666105741132,0.0240454657305778,
-0.234535580071299));
#29769=CARTESIAN_POINT('Ctrl Pts',(0.131488708832863,0.246867783152248,
-0.226615125145514));
#29770=CARTESIAN_POINT('Ctrl Pts',(-0.135543347739516,0.244665044076997,
-0.218694670219728));
#29771=CARTESIAN_POINT('Ctrl Pts',(-0.279024857986706,0.0194450904200208,
-0.210774215293942));
#29772=CARTESIAN_POINT('Ctrl Pts',(-0.16816947728471,-0.22349946266274,
-0.202853760368156));
#29773=CARTESIAN_POINT('Ctrl Pts',(0.0959758371105592,-0.2627196635205,
-0.19493330544237));
#29774=CARTESIAN_POINT('Ctrl Pts',(0.272637204187818,-0.0624654931863752,
-0.187012850516584));
#29775=CARTESIAN_POINT('Ctrl Pts',(0.200784157779961,0.194727257525179,
-0.179092395590798));
#29776=CARTESIAN_POINT('Ctrl Pts',(-0.0540877732875199,0.274422112280922,
-0.171171940665012));
#29777=CARTESIAN_POINT('Ctrl Pts',(-0.259657588620603,0.103975573111241,
-0.163251485739227));
#29778=CARTESIAN_POINT('Ctrl Pts',(-0.22854417526577,-0.161246836681637,
-0.155331030813441));
#29779=CARTESIAN_POINT('Ctrl Pts',(0.0108919462487035,-0.279489442908015,
-0.147410575887655));
#29780=CARTESIAN_POINT('Ctrl Pts',(0.240399841192072,-0.142971677518545,
-0.139490120961869));
#29781=CARTESIAN_POINT('Ctrl Pts',(0.250778329803031,0.123867705627845,
-0.131569666036083));
#29782=CARTESIAN_POINT('Ctrl Pts',(0.0325672407517647,0.277799137330094,
-0.123649211110297));
#29783=CARTESIAN_POINT('Ctrl Pts',(-0.21532960003859,0.178510933950667,
-0.115728756184511));
#29784=CARTESIAN_POINT('Ctrl Pts',(-0.26694900515942,-0.0834936273300177,
-0.107808301258725));
#29785=CARTESIAN_POINT('Ctrl Pts',(-0.0752390613443519,-0.269392081402363,
-0.0998878463329399));
#29786=CARTESIAN_POINT('Ctrl Pts',(0.185053125367525,-0.209734024160208,
-0.0919673914071537));
#29787=CARTESIAN_POINT('Ctrl Pts',(0.276665030244187,0.0411007263840873,
-0.0840469364813679));
#29788=CARTESIAN_POINT('Ctrl Pts',(0.116092131956281,0.254471660318029,
-0.0761264815555821));
#29789=CARTESIAN_POINT('Ctrl Pts',(-0.150303136702303,0.235885801608879,
-0.0682060266297961));
#29790=CARTESIAN_POINT('Ctrl Pts',(-0.27969019521417,0.00228641533845606,
-0.0602855717040106));
#29791=CARTESIAN_POINT('Ctrl Pts',(-0.154141138558003,-0.233399416954208,
-0.0523651167782244));
#29792=CARTESIAN_POINT('Ctrl Pts',(0.111924496683754,-0.256332455607864,
-0.0444446618524387));
#29793=CARTESIAN_POINT('Ctrl Pts',(0.275942502520604,-0.045621610519772,
-0.0365242069266528));
#29794=CARTESIAN_POINT('Ctrl Pts',(0.188482939221567,0.206690260966205,
-0.0286037520008668));
#29795=CARTESIAN_POINT('Ctrl Pts',(-0.0708771577509975,0.270569323408663,
-0.0206832970750811));
#29796=CARTESIAN_POINT('Ctrl Pts',(-0.265451359690944,0.0878766903016184,
-0.0127628421492951));
#29797=CARTESIAN_POINT('Ctrl Pts',(-0.218406738217093,-0.17502771504406,
-0.00484238722350926));
#29798=CARTESIAN_POINT('Ctrl Pts',(0.0284082345609573,-0.278176363862425,
0.00307806770227645));
#29799=CARTESIAN_POINT('Ctrl Pts',(0.174650305361468,-0.178204565779739,
0.00835837098613384));
#29800=CARTESIAN_POINT('Ctrl Pts',(0.210593026705004,-0.108335856152178,
0.0109985226280624));
#29801=CARTESIAN_POINT('Ctrl Pts',(-0.106883061872243,0.221955701852451,
-1.16365));
#29802=CARTESIAN_POINT('Ctrl Pts',(-0.180521580324393,0.186494975868788,
-1.16100984835807));
#29803=CARTESIAN_POINT('Ctrl Pts',(-0.288485599091745,0.0371634456178085,
-1.15572954507421));
#29804=CARTESIAN_POINT('Ctrl Pts',(-0.187989093432738,-0.222315811282613,
-1.14780909014843));
#29805=CARTESIAN_POINT('Ctrl Pts',(0.0841051337500907,-0.278439964087712,
-1.13988863522264));
#29806=CARTESIAN_POINT('Ctrl Pts',(0.279411572042703,-0.0811166623257269,
-1.13196818029685));
#29807=CARTESIAN_POINT('Ctrl Pts',(0.220093657463047,0.190331640252271,
-1.12404772537107));
#29808=CARTESIAN_POINT('Ctrl Pts',(-0.0398783372889031,0.288191347831854,
-1.11612727044528));
#29809=CARTESIAN_POINT('Ctrl Pts',(-0.263482418113243,0.123409954533181,
-1.1082068155195));
#29810=CARTESIAN_POINT('Ctrl Pts',(-0.246926329545785,-0.153889110695858,
-1.10028636059371));
#29811=CARTESIAN_POINT('Ctrl Pts',(-0.005286834857043,-0.290900898694837,
-1.09236590566793));
#29812=CARTESIAN_POINT('Ctrl Pts',(0.241169095517854,-0.162758009825391,
-1.08444545074214));
#29813=CARTESIAN_POINT('Ctrl Pts',(0.267795820779662,0.113746080290794,
-1.07652499581635));
#29814=CARTESIAN_POINT('Ctrl Pts',(0.0503204266408948,0.286566212040031,
-1.06860454089057));
#29815=CARTESIAN_POINT('Ctrl Pts',(-0.213022687825685,0.198176442773689,
-1.06068408596478));
#29816=CARTESIAN_POINT('Ctrl Pts',(-0.282191446856532,-0.0708557990322463,
-1.052763631039));
#29817=CARTESIAN_POINT('Ctrl Pts',(-0.0941367982128068,-0.275301222514972,
-1.04484317611321));
#29818=CARTESIAN_POINT('Ctrl Pts',(0.179725420377883,-0.228804084117637,
-1.03692272118743));
#29819=CARTESIAN_POINT('Ctrl Pts',(0.289764254997235,0.0262527615507647,
-1.02900226626164));
#29820=CARTESIAN_POINT('Ctrl Pts',(0.135677002228963,0.257379631685058,
-1.02108181133585));
#29821=CARTESIAN_POINT('Ctrl Pts',(-0.142082617566283,0.253899702558034,
-1.01316135641007));
#29822=CARTESIAN_POINT('Ctrl Pts',(-0.290331016493273,0.0189849657278787,
-1.00524090148428));
#29823=CARTESIAN_POINT('Ctrl Pts',(-0.173936726479704,-0.233234951015106,
-0.997320446558496));
#29824=CARTESIAN_POINT('Ctrl Pts',(0.101004462246637,-0.272856421227669,
-0.989399991632712));
#29825=CARTESIAN_POINT('Ctrl Pts',(0.283878009016785,-0.0637636555936547,
-0.981479536706925));
#29826=CARTESIAN_POINT('Ctrl Pts',(0.207990917668981,0.203450991269769,
-0.973559081781138));
#29827=CARTESIAN_POINT('Ctrl Pts',(-0.0574841683522745,0.285215879969544,
-0.965638626855354));
#29828=CARTESIAN_POINT('Ctrl Pts',(-0.270561253939026,0.107000633759307,
-0.957718171929567));
#29829=CARTESIAN_POINT('Ctrl Pts',(-0.237016197548405,-0.168747888426155,
-0.949797717003782));
#29830=CARTESIAN_POINT('Ctrl Pts',(0.0125739926281641,-0.290679243281013,
-0.941877262077995));
#29831=CARTESIAN_POINT('Ctrl Pts',(0.250702730191592,-0.147650495538245,
-0.933956807152211));
#29832=CARTESIAN_POINT('Ctrl Pts',(0.260310778228486,0.129964712501675,
-0.926036352226424));
#29833=CARTESIAN_POINT('Ctrl Pts',(0.0326402035564766,0.289114414845776,
-0.918115897300638));
#29834=CARTESIAN_POINT('Ctrl Pts',(-0.224782587286331,0.184730387894277,
-0.910195442374853));
#29835=CARTESIAN_POINT('Ctrl Pts',(-0.277311431423173,-0.0880391830990681,
-0.902274987449066));
#29836=CARTESIAN_POINT('Ctrl Pts',(-0.0770652081648057,-0.280559229842002,
-0.894354532523281));
#29837=CARTESIAN_POINT('Ctrl Pts',(0.193427535721404,-0.217343774200207,
-0.886434077597494));
#29838=CARTESIAN_POINT('Ctrl Pts',(0.287607106626291,0.0439849971799122,
-0.878513622671709));
#29839=CARTESIAN_POINT('Ctrl Pts',(0.119626890652448,0.265220539912974,
-0.870593167745923));
#29840=CARTESIAN_POINT('Ctrl Pts',(-0.157395694010782,0.244702111281736,
-0.862672712820137));
#29841=CARTESIAN_POINT('Ctrl Pts',(-0.290948869723938,0.00113268055633667,
-0.854752257894351));
#29842=CARTESIAN_POINT('Ctrl Pts',(-0.159296172834772,-0.243469211768303,
-0.846831802968566));
#29843=CARTESIAN_POINT('Ctrl Pts',(0.117558258499843,-0.266143915236407,
-0.838911348042778));
#29844=CARTESIAN_POINT('Ctrl Pts',(0.287255921854422,-0.046222971761319,
-0.830990893116994));
#29845=CARTESIAN_POINT('Ctrl Pts',(0.195113910465212,0.215831160173538,
-0.823070438191208));
#29846=CARTESIAN_POINT('Ctrl Pts',(-0.0748784391324881,0.281150755133191,
-0.815149983265422));
#29847=CARTESIAN_POINT('Ctrl Pts',(-0.276617553005043,0.0901956602524961,
-0.807229528339636));
#29848=CARTESIAN_POINT('Ctrl Pts',(-0.226214083916436,-0.182974632112567,
-0.799309073413849));
#29849=CARTESIAN_POINT('Ctrl Pts',(0.0303881704670555,-0.289359787901752,
-0.791388618488065));
#29850=CARTESIAN_POINT('Ctrl Pts',(0.259290983113068,-0.131987551818876,
-0.783468163562277));
#29851=CARTESIAN_POINT('Ctrl Pts',(0.251844737246961,0.145694049569263,
-0.775547708636494));
#29852=CARTESIAN_POINT('Ctrl Pts',(0.0148368389666054,0.290572531338322,
-0.767627253710706));
#29853=CARTESIAN_POINT('Ctrl Pts',(-0.235695142870192,0.170588180675806,
-0.759706798784921));
#29854=CARTESIAN_POINT('Ctrl Pts',(-0.27138615937748,-0.104890801585375,
-0.751786343859135));
#29855=CARTESIAN_POINT('Ctrl Pts',(-0.0597031156995855,-0.284759663110216,
-0.743865888933349));
#29856=CARTESIAN_POINT('Ctrl Pts',(0.206400544601464,-0.205064241024857,
-0.735945434007563));
#29857=CARTESIAN_POINT('Ctrl Pts',(0.284365867783122,0.0615514500140597,
-0.728024979081777));
#29858=CARTESIAN_POINT('Ctrl Pts',(0.103125859886165,0.272061729726216,
-0.720104524155992));
#29859=CARTESIAN_POINT('Ctrl Pts',(-0.17211548812573,0.234582153000017,
-0.712184069230205));
#29860=CARTESIAN_POINT('Ctrl Pts',(-0.290470032418224,-0.0167238759214858,
-0.70426361430442));
#29861=CARTESIAN_POINT('Ctrl Pts',(-0.144055174150759,-0.252785748331024,
-0.696343159378634));
#29862=CARTESIAN_POINT('Ctrl Pts',(0.133668935119408,-0.258428217389133,
-0.688422704452848));
#29863=CARTESIAN_POINT('Ctrl Pts',(0.289551063660099,-0.0285080566189151,
-0.680502249527062));
#29864=CARTESIAN_POINT('Ctrl Pts',(0.181501448545034,0.227397783487298,
-0.672581794601277));
#29865=CARTESIAN_POINT('Ctrl Pts',(-0.0919904660560023,0.276025871819438,
-0.66466133967549));
#29866=CARTESIAN_POINT('Ctrl Pts',(-0.281631180806615,0.0730507067478044,
-0.656740884749705));
#29867=CARTESIAN_POINT('Ctrl Pts',(-0.214559287844702,-0.196511678427659,
-0.648820429823918));
#29868=CARTESIAN_POINT('Ctrl Pts',(0.0480878043327292,-0.286949631178259,
-0.640899974898133));
#29869=CARTESIAN_POINT('Ctrl Pts',(0.266901874846621,-0.115827099429452,
-0.632979519972346));
#29870=CARTESIAN_POINT('Ctrl Pts',(0.242429402659526,0.160874213238254,
-0.625059065046561));
#29871=CARTESIAN_POINT('Ctrl Pts',(-0.00302245101747099,0.29093537521025,
-0.617138610120775));
#29872=CARTESIAN_POINT('Ctrl Pts',(-0.245719278492625,0.155802965106398,
-0.609218155194989));
#29873=CARTESIAN_POINT('Ctrl Pts',(-0.264437935062065,-0.121347048826877,
-0.601297700269203));
#29874=CARTESIAN_POINT('Ctrl Pts',(-0.0421159806683627,-0.287886734552365,
-0.593377245343418));
#29875=CARTESIAN_POINT('Ctrl Pts',(0.218595555421444,-0.19201174679918,
-0.585456790417632));
#29876=CARTESIAN_POINT('Ctrl Pts',(0.280052751470189,0.0788858932437061,
-0.577536335491846));
#29877=CARTESIAN_POINT('Ctrl Pts',(0.086236110577048,0.277877420801736,
-0.56961588056606));
#29878=CARTESIAN_POINT('Ctrl Pts',(-0.186186516918199,0.223577970016616,
-0.561695425640274));
#29879=CARTESIAN_POINT('Ctrl Pts',(-0.288896308845701,-0.0345173940819846,
-0.553774970714489));
#29880=CARTESIAN_POINT('Ctrl Pts',(-0.128271179583394,-0.261149444278877,
-0.545854515788702));
#29881=CARTESIAN_POINT('Ctrl Pts',(0.149275765334778,-0.249738410426987,
-0.537934060862917));
#29882=CARTESIAN_POINT('Ctrl Pts',(0.290754783123506,-0.0106856843339418,
-0.530013605937131));
#29883=CARTESIAN_POINT('Ctrl Pts',(0.167204842233907,0.238107262578057,
-0.522093151011345));
#29884=CARTESIAN_POINT('Ctrl Pts',(-0.108755747750336,0.269860547487303,
-0.514172696085559));
#29885=CARTESIAN_POINT('Ctrl Pts',(-0.285583239159514,0.0556303987945563,
-0.506252241159773));
#29886=CARTESIAN_POINT('Ctrl Pts',(-0.202095740468328,-0.20930800138418,
-0.498331786233988));
#29887=CARTESIAN_POINT('Ctrl Pts',(0.06560617792819,-0.283457857849339,
-0.490411331308201));
#29888=CARTESIAN_POINT('Ctrl Pts',(0.27350671719559,-0.0992300529465394,
-0.482490876382416));
#29889=CARTESIAN_POINT('Ctrl Pts',(0.232100264257521,0.175447984002298,
-0.47457042145663));
#29890=CARTESIAN_POINT('Ctrl Pts',(-0.0208703482940667,0.29020157877063,
-0.466649966530844));
#29891=CARTESIAN_POINT('Ctrl Pts',(-0.254817209572468,0.140430471994444,
-0.458729511605058));
#29892=CARTESIAN_POINT('Ctrl Pts',(-0.256492948839367,-0.137345895295664,
-0.450809056679272));
#29893=CARTESIAN_POINT('Ctrl Pts',(-0.0243700953231664,-0.289928657108644,
-0.442888601753487));
#29894=CARTESIAN_POINT('Ctrl Pts',(0.229966600789207,-0.178235491079467,
-0.4349681468277));
#29895=CARTESIAN_POINT('Ctrl Pts',(0.274684015377781,0.0959229871033038,
-0.427047691901915));
#29896=CARTESIAN_POINT('Ctrl Pts',(0.069021306278996,0.282645691703275,
-0.419127236976129));
#29897=CARTESIAN_POINT('Ctrl Pts',(-0.199555741608052,0.211731041064228,
-0.411206782050343));
#29898=CARTESIAN_POINT('Ctrl Pts',(-0.286233630937844,-0.0521808037406457,
-0.403286327124557));
#29899=CARTESIAN_POINT('Ctrl Pts',(-0.112003684698342,-0.268528773826709,
-0.395365872198771));
#29900=CARTESIAN_POINT('Ctrl Pts',(0.164319921376595,-0.240107249365093,
-0.387445417272986));
#29901=CARTESIAN_POINT('Ctrl Pts',(0.290862542992046,0.0071769661474798,
-0.379524962347199));
#29902=CARTESIAN_POINT('Ctrl Pts',(0.152277980594956,0.247919229558346,
-0.371604507421414));
#29903=CARTESIAN_POINT('Ctrl Pts',(-0.125111089824882,0.262678021466798,
-0.363684052495627));
#29904=CARTESIAN_POINT('Ctrl Pts',(-0.288458831331091,0.0380003998134609,
-0.355763597569842));
#29905=CARTESIAN_POINT('Ctrl Pts',(-0.188870421390492,-0.221315367027822,
-0.347843142644056));
#29906=CARTESIAN_POINT('Ctrl Pts',(0.0828772581879734,-0.278897629667457,
-0.33992268771827));
#29907=CARTESIAN_POINT('Ctrl Pts',(0.279080614128112,-0.0822589726215777,
-0.332002232792485));
#29908=CARTESIAN_POINT('Ctrl Pts',(0.220896256287244,0.189360428065534,
-0.324081777866698));
#29909=CARTESIAN_POINT('Ctrl Pts',(-0.0386395777041695,0.288373907962778,
-0.316161322940913));
#29910=CARTESIAN_POINT('Ctrl Pts',(-0.262954642727673,0.124528645808272,
-0.308240868015126));
#29911=CARTESIAN_POINT('Ctrl Pts',(-0.247581148226634,-0.152827035571806,
-0.300320413089341));
#29912=CARTESIAN_POINT('Ctrl Pts',(-0.00653235030325454,-0.29087773403682,
-0.292399958163555));
#29913=CARTESIAN_POINT('Ctrl Pts',(0.240470819135481,-0.16378740153988,
-0.284479503237769));
#29914=CARTESIAN_POINT('Ctrl Pts',(0.268279896207693,0.112598512644225,
-0.276559048311983));
#29915=CARTESIAN_POINT('Ctrl Pts',(0.0515463357952915,0.286348569098821,
-0.268638593386197));
#29916=CARTESIAN_POINT('Ctrl Pts',(-0.212172768767697,0.199086021488941,
-0.260718138460411));
#29917=CARTESIAN_POINT('Ctrl Pts',(-0.282492035287816,-0.0696475251388723,
-0.252797683534626));
#29918=CARTESIAN_POINT('Ctrl Pts',(-0.0953140075478283,-0.274895921621062,
-0.24487722860884));
#29919=CARTESIAN_POINT('Ctrl Pts',(0.178744696396482,-0.229571037521802,
-0.236956773683054));
#29920=CARTESIAN_POINT('Ctrl Pts',(0.289873937081507,0.0250125640566995,
-0.229036318757268));
#29921=CARTESIAN_POINT('Ctrl Pts',(0.136777128347834,0.25679669958643,-0.221115863831482));
#29922=CARTESIAN_POINT('Ctrl Pts',(-0.140994843093548,0.254505367289637,
-0.213195408905696));
#29923=CARTESIAN_POINT('Ctrl Pts',(-0.290247118188642,0.0202271636228108,
-0.20527495397991));
#29924=CARTESIAN_POINT('Ctrl Pts',(-0.174933181585931,-0.232488515262181,
-0.197354499054125));
#29925=CARTESIAN_POINT('Ctrl Pts',(0.0998359441451969,-0.273286135789191,
-0.189434044128339));
#29926=CARTESIAN_POINT('Ctrl Pts',(0.283602555691625,-0.0649778285504636,
-0.181513589202553));
#29927=CARTESIAN_POINT('Ctrl Pts',(0.208859610552489,0.202559104365367,
-0.173593134276767));
#29928=CARTESIAN_POINT('Ctrl Pts',(-0.0562631603478542,0.285459252023246,
-0.165672679350981));
#29929=CARTESIAN_POINT('Ctrl Pts',(-0.270100905549183,0.108157426099247,
-0.157752224425195));
#29930=CARTESIAN_POINT('Ctrl Pts',(-0.23773612404401,-0.167732115344754,
-0.149831769499409));
#29931=CARTESIAN_POINT('Ctrl Pts',(0.0113300156586853,-0.290730388516371,
-0.141911314573624));
#29932=CARTESIAN_POINT('Ctrl Pts',(0.250068619772689,-0.148721937112609,
-0.133990859647838));
#29933=CARTESIAN_POINT('Ctrl Pts',(0.2608645267475,0.128849611660169,-0.126070404722052));
#29934=CARTESIAN_POINT('Ctrl Pts',(0.0338770812169207,0.288972099572548,
-0.118149949796266));
#29935=CARTESIAN_POINT('Ctrl Pts',(-0.223990064264781,0.185690567206784,
-0.11022949487048));
#29936=CARTESIAN_POINT('Ctrl Pts',(-0.277685579736189,-0.0868517052369887,
-0.102309039944694));
#29937=CARTESIAN_POINT('Ctrl Pts',(-0.078265144145175,-0.280226915458554,
-0.0943885850189086));
#29938=CARTESIAN_POINT('Ctrl Pts',(0.192495882758534,-0.218169436722758,
-0.0864681300931225));
#29939=CARTESIAN_POINT('Ctrl Pts',(0.287792379185709,0.0427537799840384,
-0.0785476751673367));
#29940=CARTESIAN_POINT('Ctrl Pts',(0.120761307748041,0.2647064014329,-0.0706272202415509));
#29941=CARTESIAN_POINT('Ctrl Pts',(-0.156348264442573,0.245373027452116,
-0.0627067653157649));
#29942=CARTESIAN_POINT('Ctrl Pts',(-0.290939214994239,0.00237837398344197,
-0.0547863103899793));
#29943=CARTESIAN_POINT('Ctrl Pts',(-0.160340629087994,-0.242786641472266,
-0.0468658554641933));
#29944=CARTESIAN_POINT('Ctrl Pts',(0.116426051971046,-0.26664203711178,
-0.0389454005384074));
#29945=CARTESIAN_POINT('Ctrl Pts',(0.287040791706749,-0.0474564921420706,
-0.0310249456126217));
#29946=CARTESIAN_POINT('Ctrl Pts',(0.196063642255814,0.215003254677608,
-0.0231044906868355));
#29947=CARTESIAN_POINT('Ctrl Pts',(-0.0737278066587491,0.281451505633798,
-0.01518403576105));
#29948=CARTESIAN_POINT('Ctrl Pts',(-0.276127699608842,0.0914110531227855,
-0.00726358083526385));
#29949=CARTESIAN_POINT('Ctrl Pts',(-0.227190963622003,-0.182067254728615,
0.00065687409052195));
#29950=CARTESIAN_POINT('Ctrl Pts',(0.029550801579613,-0.289364497994335,
0.00857732901630768));
#29951=CARTESIAN_POINT('Ctrl Pts',(0.181674665790342,-0.185371877039327,
0.0138576323001651));
#29952=CARTESIAN_POINT('Ctrl Pts',(0.219062987981749,-0.112693077855332,
0.0164977839420937));
#29953=CARTESIAN_POINT('',(-0.204509257318296,-0.138028148648276,-2.52416797836347E-16));
#29954=CARTESIAN_POINT('Ctrl Pts',(-0.204513561691918,-0.138033045165328,
7.97972798949331E-17));
#29955=CARTESIAN_POINT('Ctrl Pts',(-0.200458969367413,-0.14343453541669,
1.13314958597239E-16));
#29956=CARTESIAN_POINT('Ctrl Pts',(-0.196176350401663,-0.14864871991259,
5.9397114527851E-16));
#29957=CARTESIAN_POINT('Ctrl Pts',(-0.191667490565443,-0.153657468545478,
4.5102810375397E-16));
#29958=CARTESIAN_POINT('Ctrl Pts',(-0.183969917901797,-0.162208456590365,
2.03524801489296E-16));
#29959=CARTESIAN_POINT('Ctrl Pts',(-0.175613388124977,-0.170161490060188,
-1.5271922467326E-16));
#29960=CARTESIAN_POINT('Ctrl Pts',(-0.166688955232968,-0.177488068326711,
-2.51534904016637E-16));
#29961=CARTESIAN_POINT('Ctrl Pts',(-0.161662997196323,-0.181614165230046,
-3.07184765890441E-16));
#29962=CARTESIAN_POINT('Ctrl Pts',(-0.156453755055607,-0.18554289472659,
-4.44006003611873E-16));
#29963=CARTESIAN_POINT('Ctrl Pts',(-0.151098143157478,-0.1892536575405,
-3.72965547335014E-16));
#29964=CARTESIAN_POINT('Ctrl Pts',(-0.143555040089887,-0.194480075529169,
-2.72908729578602E-16));
#29965=CARTESIAN_POINT('Ctrl Pts',(-0.135714281411093,-0.199281170935203,
-2.35696859612518E-16));
#29966=CARTESIAN_POINT('Ctrl Pts',(-0.127621690156068,-0.203642056189206,
-3.22658566531686E-16));
#29967=CARTESIAN_POINT('Ctrl Pts',(-0.122072656842052,-0.206632284756358,
-3.82287601723413E-16));
#29968=CARTESIAN_POINT('Ctrl Pts',(-0.1164051378392,-0.209415418232596,
-3.70654868758527E-16));
#29969=CARTESIAN_POINT('Ctrl Pts',(-0.110633357581212,-0.211984946769715,
-3.81639164714898E-16));
#29970=CARTESIAN_POINT('Ctrl Pts',(-0.106100414669248,-0.214002959522939,
-3.90265824821965E-16));
#29971=CARTESIAN_POINT('Ctrl Pts',(-0.101501721030156,-0.21588944006491,
-4.94020418234288E-16));
#29972=CARTESIAN_POINT('Ctrl Pts',(-0.0968614704712326,-0.217634943816702,
-4.9960036108132E-16));
#29973=CARTESIAN_POINT('Ctrl Pts',(-0.0826821613338624,-0.222968715556572,
-5.16651107283974E-16));
#29974=CARTESIAN_POINT('Ctrl Pts',(-0.0680806317286739,-0.227006644225286,
-3.92788537165852E-16));
#29975=CARTESIAN_POINT('Ctrl Pts',(-0.0532579471984103,-0.229671072551787,
-4.04190569902596E-16));
#29976=CARTESIAN_POINT('Ctrl Pts',(-0.0416423014901125,-0.231759024662797,
-4.13125656684887E-16));
#29977=CARTESIAN_POINT('Ctrl Pts',(-0.0298901490078552,-0.233002671776119,
-2.53258607599116E-16));
#29978=CARTESIAN_POINT('Ctrl Pts',(-0.0180992304553012,-0.233341545130159,
-2.41126563160776E-16));
#29979=CARTESIAN_POINT('Ctrl Pts',(-0.014418495701006,-0.2334473301821,
-2.37339340188637E-16));
#29980=CARTESIAN_POINT('Ctrl Pts',(-0.0107362607675731,-0.233464579565444,
-5.5259238222526E-16));
#29981=CARTESIAN_POINT('Ctrl Pts',(-0.00706437366680782,-0.233391940295786,
-5.25621213220973E-16));
#29982=CARTESIAN_POINT('Ctrl Pts',(0.00313705648947054,-0.233190130050622,
-4.50688490814264E-16));
#29983=CARTESIAN_POINT('Ctrl Pts',(0.0132783977524309,-0.232296137191171,
-2.4101113858591E-16));
#29984=CARTESIAN_POINT('Ctrl Pts',(0.0232964001888359,-0.230679356207016,
-1.64798730217797E-16));
#29985=CARTESIAN_POINT('Ctrl Pts',(0.0344038527887266,-0.228886751517617,
-8.36100771269679E-17));
#29986=CARTESIAN_POINT('Ctrl Pts',(0.0453601005161749,-0.226205689418119,
-9.88173003853937E-17));
#29987=CARTESIAN_POINT('Ctrl Pts',(0.0560899933785598,-0.222695008049497,
-1.50053580671994E-16));
#29988=CARTESIAN_POINT('Ctrl Pts',(0.0605383051258949,-0.221239578310032,
-1.71294701194979E-16));
#29989=CARTESIAN_POINT('Ctrl Pts',(0.0649476163018993,-0.219641368744839,
-2.82468155353174E-16));
#29990=CARTESIAN_POINT('Ctrl Pts',(0.0693120640699186,-0.217903830273792,
-3.35668992601512E-16));
#29991=CARTESIAN_POINT('Ctrl Pts',(0.0726902936253035,-0.216558916981549,
-3.76848232293759E-16));
#29992=CARTESIAN_POINT('Ctrl Pts',(0.0760395849689661,-0.215131185718671,
-1.66001976769033E-16));
#29993=CARTESIAN_POINT('Ctrl Pts',(0.0793492735533264,-0.21362643030463,
-1.39645239816133E-16));
#29994=CARTESIAN_POINT('Ctrl Pts',(0.0918661238439923,-0.2079356235228,
-3.99671818414834E-17));
#29995=CARTESIAN_POINT('Ctrl Pts',(0.103852408746883,-0.201132648912409,
1.2723644335876E-17));
#29996=CARTESIAN_POINT('Ctrl Pts',(0.115173520844875,-0.193329455672931,
-1.16226472890446E-16));
#29997=CARTESIAN_POINT('Ctrl Pts',(0.125337633549786,-0.186323736194337,
-2.31998096159875E-16));
#29998=CARTESIAN_POINT('Ctrl Pts',(0.134965897482742,-0.178510810996301,
1.26912968512929E-16));
#29999=CARTESIAN_POINT('Ctrl Pts',(0.14394042956759,-0.169952142766193,
2.51101223147643E-16));
#30000=CARTESIAN_POINT('Ctrl Pts',(0.146996369828429,-0.167037809341757,
2.93388874879624E-16));
#30001=CARTESIAN_POINT('Ctrl Pts',(0.149970279662056,-0.164042501082029,
3.04623096677509E-16));
#30002=CARTESIAN_POINT('Ctrl Pts',(0.15285458649515,-0.160973061898707,
2.53269627492614E-16));
#30003=CARTESIAN_POINT('Ctrl Pts',(0.162422461331181,-0.150791062679389,
8.2918969955242E-17));
#30004=CARTESIAN_POINT('Ctrl Pts',(0.171020780523213,-0.139782655946406,
-2.2682857248612E-16));
#30005=CARTESIAN_POINT('Ctrl Pts',(0.178487646579902,-0.128046791389447,
-3.42174205636425E-16));
#30006=CARTESIAN_POINT('Ctrl Pts',(0.184248186336547,-0.118992803565679,
-4.31161084532231E-16));
#30007=CARTESIAN_POINT('Ctrl Pts',(0.189334785443673,-0.1095050565137,2.58952566004617E-17));
#30008=CARTESIAN_POINT('Ctrl Pts',(0.193653104151514,-0.0996214127458699,
0.));
#30009=CARTESIAN_POINT('Ctrl Pts',(-0.246160120813712,0.000192360259597545,
-0.00472127808698222));
#30010=CARTESIAN_POINT('Ctrl Pts',(-0.24582237483402,-0.0486236404045207,
-0.00314751872465485));
#30011=CARTESIAN_POINT('Ctrl Pts',(-0.231427963796332,-0.0976359744578188,
-0.0015737593623275));
#30012=CARTESIAN_POINT('Ctrl Pts',(-0.204513561691922,-0.138033045165322,
-1.45716771982052E-16));
#30013=CARTESIAN_POINT('',(-0.126471106027292,-0.177287929553124,-1.16365));
#30014=CARTESIAN_POINT('Ctrl Pts',(-0.126742452678739,-0.177514072314448,
-1.16365));
#30015=CARTESIAN_POINT('Ctrl Pts',(-0.131861338221367,-0.174371803129766,
-1.16365));
#30016=CARTESIAN_POINT('Ctrl Pts',(-0.136831729034579,-0.171012070470409,
-1.16365));
#30017=CARTESIAN_POINT('Ctrl Pts',(-0.141637451548538,-0.167437627045634,
-1.16365));
#30018=CARTESIAN_POINT('Ctrl Pts',(-0.150897109985627,-0.160550395184039,
-1.16365));
#30019=CARTESIAN_POINT('Ctrl Pts',(-0.159546413429048,-0.152867380212311,
-1.16365));
#30020=CARTESIAN_POINT('Ctrl Pts',(-0.16755538633808,-0.144504071864687,
-1.16365));
#30021=CARTESIAN_POINT('Ctrl Pts',(-0.17090995218102,-0.141001092289706,
-1.16365));
#30022=CARTESIAN_POINT('Ctrl Pts',(-0.174151378696826,-0.137378738244585,
-1.16365));
#30023=CARTESIAN_POINT('Ctrl Pts',(-0.177268691376915,-0.133655610415481,
-1.16365));
#30024=CARTESIAN_POINT('Ctrl Pts',(-0.186038283781417,-0.12318174498015,
-1.16365));
#30025=CARTESIAN_POINT('Ctrl Pts',(-0.193847100730409,-0.111893260660668,
-1.16365));
#30026=CARTESIAN_POINT('Ctrl Pts',(-0.200640170312477,-0.0999687378212474,
-1.16365));
#30027=CARTESIAN_POINT('Ctrl Pts',(-0.203365214294673,-0.0951852082531265,
-1.16365));
#30028=CARTESIAN_POINT('Ctrl Pts',(-0.205927329765095,-0.0902963247364379,
-1.16365));
#30029=CARTESIAN_POINT('Ctrl Pts',(-0.208311993322315,-0.0853347291837548,
-1.16365));
#30030=CARTESIAN_POINT('Ctrl Pts',(-0.214711771281109,-0.072019177913485,
-1.16365));
#30031=CARTESIAN_POINT('Ctrl Pts',(-0.219855302751287,-0.0581522607815734,
-1.16365));
#30032=CARTESIAN_POINT('Ctrl Pts',(-0.223672726060924,-0.0439462398011037,
-1.16365));
#30033=CARTESIAN_POINT('Ctrl Pts',(-0.226338842024177,-0.0340246523222635,
-1.16365));
#30034=CARTESIAN_POINT('Ctrl Pts',(-0.228357386302339,-0.0239367220668382,
-1.16365));
#30035=CARTESIAN_POINT('Ctrl Pts',(-0.229690730670339,-0.013748733749612,
-1.16365));
#30036=CARTESIAN_POINT('Ctrl Pts',(-0.230229670333924,-0.00963073458295048,
-1.16365));
#30037=CARTESIAN_POINT('Ctrl Pts',(-0.230656273552338,-0.00549607418239393,
-1.16365));
#30038=CARTESIAN_POINT('Ctrl Pts',(-0.230967088650693,-0.00136420452645389,
-1.16365));
#30039=CARTESIAN_POINT('Ctrl Pts',(-0.231742593736289,0.00894509495149809,
-1.16365));
#30040=CARTESIAN_POINT('Ctrl Pts',(-0.231801493177623,0.0192593571944351,
-1.16365));
#30041=CARTESIAN_POINT('Ctrl Pts',(-0.231115915127983,0.0295095610734199,
-1.16365));
#30042=CARTESIAN_POINT('Ctrl Pts',(-0.230457433078469,0.0393546476565208,
-1.16365));
#30043=CARTESIAN_POINT('Ctrl Pts',(-0.229112221005407,0.0491408939728083,
-1.16365));
#30044=CARTESIAN_POINT('Ctrl Pts',(-0.227122783666268,0.0588215211318158,
-1.16365));
#30045=CARTESIAN_POINT('Ctrl Pts',(-0.22602341141252,0.0641710803705567,
-1.16365));
#30046=CARTESIAN_POINT('Ctrl Pts',(-0.224727103207668,0.0694883890758916,
-1.16365));
#30047=CARTESIAN_POINT('Ctrl Pts',(-0.223239600591205,0.074765365573958,
-1.16365));
#30048=CARTESIAN_POINT('Ctrl Pts',(-0.222045632550997,0.0790010161320732,
-1.16365));
#30049=CARTESIAN_POINT('Ctrl Pts',(-0.220727846656266,0.083211665253357,
-1.16365));
#30050=CARTESIAN_POINT('Ctrl Pts',(-0.219295202918089,0.0873767379509316,
-1.16365));
#30051=CARTESIAN_POINT('Ctrl Pts',(-0.21444725735436,0.101470992627617,
-1.16365));
#30052=CARTESIAN_POINT('Ctrl Pts',(-0.208276894357113,0.115087695452192,
-1.16365));
#30053=CARTESIAN_POINT('Ctrl Pts',(-0.200926527149074,0.128072014981204,
-1.16365));
#30054=CARTESIAN_POINT('Ctrl Pts',(-0.197308721049431,0.134462818197185,
-1.16365));
#30055=CARTESIAN_POINT('Ctrl Pts',(-0.193404247750143,0.140700343051493,
-1.16365));
#30056=CARTESIAN_POINT('Ctrl Pts',(-0.189225861417297,0.146764841991167,
-1.16365));
#30057=CARTESIAN_POINT('Ctrl Pts',(-0.18619672096879,0.151161328475361,
-1.16365));
#30058=CARTESIAN_POINT('Ctrl Pts',(-0.183023566145792,0.155466860400186,
-1.16365));
#30059=CARTESIAN_POINT('Ctrl Pts',(-0.179710475436982,0.159673387333553,
-1.16365));
#30060=CARTESIAN_POINT('Ctrl Pts',(-0.176874734026243,0.163273838896385,
-1.16365));
#30061=CARTESIAN_POINT('Ctrl Pts',(-0.17394079312019,0.166796008550431,
-1.16365));
#30062=CARTESIAN_POINT('Ctrl Pts',(-0.170917645960835,0.170229306991485,
-1.16365));
#30063=CARTESIAN_POINT('Ctrl Pts',(-0.160759806788243,0.181765263250785,
-1.16365));
#30064=CARTESIAN_POINT('Ctrl Pts',(-0.149580565015023,0.192322357430371,
-1.16365));
#30065=CARTESIAN_POINT('Ctrl Pts',(-0.137500883169785,0.201728680603211,
-1.16365));
#30066=CARTESIAN_POINT('Ctrl Pts',(-0.127855257975516,0.209239629065579,
-1.16365));
#30067=CARTESIAN_POINT('Ctrl Pts',(-0.117634401071449,0.216016836489331,
-1.16365));
#30068=CARTESIAN_POINT('Ctrl Pts',(-0.106883061872243,0.221955701852451,
-1.16365));
#30069=CARTESIAN_POINT('Ctrl Pts',(-0.126742452678738,-0.177514072314449,
-1.16365));
#30070=CARTESIAN_POINT('Ctrl Pts',(-0.0727848118484482,-0.215552950999294,
-1.16122880638825));
#30071=CARTESIAN_POINT('Ctrl Pts',(0.0791223892213512,-0.241320543762611,
-1.15616746113456));
#30072=CARTESIAN_POINT('Ctrl Pts',(0.247001644414856,-0.0717076563344237,
-1.14846596423895));
#30073=CARTESIAN_POINT('Ctrl Pts',(0.194564222666998,0.168254406153596,
-1.14054550931316));
#30074=CARTESIAN_POINT('Ctrl Pts',(-0.0352527091661894,0.254763023235567,
-1.13262505438738));
#30075=CARTESIAN_POINT('Ctrl Pts',(-0.196026712503706,0.136283234411974,
-1.12618290529268));
#30076=CARTESIAN_POINT('Ctrl Pts',(-0.21753268144054,0.0319805760390736,
-1.12238090783991));
#30077=CARTESIAN_POINT('Ctrl Pts',(-0.217441534898734,7.07751596318099E-5,
-1.12121906202908));
#30078=CARTESIAN_POINT('Origin',(-2.26018097944867E-17,0.,-1.16365));
#30079=CARTESIAN_POINT('',(-0.24635,-3.01691738969951E-17,-1.16365));
#30080=CARTESIAN_POINT('Origin',(0.,0.,-1.16365));
#30081=CARTESIAN_POINT('Origin',(0.,0.,-1.16365));
#30082=CARTESIAN_POINT('',(0.126471106027295,-0.177287929553122,-1.16365));
#30083=CARTESIAN_POINT('Ctrl Pts',(0.10714206075237,0.222259968661296,-1.16365));
#30084=CARTESIAN_POINT('Ctrl Pts',(0.113071151342837,0.219025513962988,
-1.16365));
#30085=CARTESIAN_POINT('Ctrl Pts',(0.118847726774383,0.21553843574513,-1.16365));
#30086=CARTESIAN_POINT('Ctrl Pts',(0.12445358873384,0.211797890271589,-1.16365));
#30087=CARTESIAN_POINT('Ctrl Pts',(0.134023975740716,0.205411991357647,
-1.16365));
#30088=CARTESIAN_POINT('Ctrl Pts',(0.143097537518038,0.198287893018338,
-1.16365));
#30089=CARTESIAN_POINT('Ctrl Pts',(0.151632957908753,0.190511595485141,
-1.16365));
#30090=CARTESIAN_POINT('Ctrl Pts',(0.156439835694909,0.18613223159212,-1.16365));
#30091=CARTESIAN_POINT('Ctrl Pts',(0.161077798201613,0.181543071307519,
-1.16365));
#30092=CARTESIAN_POINT('Ctrl Pts',(0.165521144850447,0.176777677610949,
-1.16365));
#30093=CARTESIAN_POINT('Ctrl Pts',(0.171779371002945,0.170065864687989,
-1.16365));
#30094=CARTESIAN_POINT('Ctrl Pts',(0.177659573392144,0.162998247969616,
-1.16365));
#30095=CARTESIAN_POINT('Ctrl Pts',(0.183140420688034,0.155618028761713,
-1.16365));
#30096=CARTESIAN_POINT('Ctrl Pts',(0.186898597060763,0.15055746714499,-1.16365));
#30097=CARTESIAN_POINT('Ctrl Pts',(0.190468900412591,0.14534983118815,-1.16365));
#30098=CARTESIAN_POINT('Ctrl Pts',(0.193842840317149,0.140008259503939,
-1.16365));
#30099=CARTESIAN_POINT('Ctrl Pts',(0.196492609601869,0.135813184019093,
-1.16365));
#30100=CARTESIAN_POINT('Ctrl Pts',(0.199021686516466,0.131534101113879,
-1.16365));
#30101=CARTESIAN_POINT('Ctrl Pts',(0.201417240773586,0.127193592262789,
-1.16365));
#30102=CARTESIAN_POINT('Ctrl Pts',(0.208737384344553,0.113930211620668,
-1.16365));
#30103=CARTESIAN_POINT('Ctrl Pts',(0.214835996804749,0.100062396156116,
-1.16365));
#30104=CARTESIAN_POINT('Ctrl Pts',(0.219607275101183,0.0857779314832026,
-1.16365));
#30105=CARTESIAN_POINT('Ctrl Pts',(0.223346238611081,0.0745840566236364,
-1.16365));
#30106=CARTESIAN_POINT('Ctrl Pts',(0.22626935672672,0.0631335084732036,
-1.16365));
#30107=CARTESIAN_POINT('Ctrl Pts',(0.228302715464478,0.0515143004487872,
-1.16365));
#30108=CARTESIAN_POINT('Ctrl Pts',(0.228937463003728,0.0478871668965153,
-1.16365));
#30109=CARTESIAN_POINT('Ctrl Pts',(0.229484813783808,0.0442457986424989,
-1.16365));
#30110=CARTESIAN_POINT('Ctrl Pts',(0.229941722688576,0.0406017253371934,
-1.16365));
#30111=CARTESIAN_POINT('Ctrl Pts',(0.231211130326128,0.030477574905268,
-1.16365));
#30112=CARTESIAN_POINT('Ctrl Pts',(0.231786917854907,0.0203132046570649,
-1.16365));
#30113=CARTESIAN_POINT('Ctrl Pts',(0.231629690263984,0.010166797456069,
-1.16365));
#30114=CARTESIAN_POINT('Ctrl Pts',(0.231455364231173,-0.00108302774480546,
-1.16365));
#30115=CARTESIAN_POINT('Ctrl Pts',(0.230380067272138,-0.0123111726630605,
-1.16365));
#30116=CARTESIAN_POINT('Ctrl Pts',(0.228451201638814,-0.0234347970229404,
-1.16365));
#30117=CARTESIAN_POINT('Ctrl Pts',(0.227651547930891,-0.0280463403628394,
-1.16365));
#30118=CARTESIAN_POINT('Ctrl Pts',(0.226704986161851,-0.0326398516094958,
-1.16365));
#30119=CARTESIAN_POINT('Ctrl Pts',(0.225614086959102,-0.0372090320414421,
-1.16365));
#30120=CARTESIAN_POINT('Ctrl Pts',(0.224769694305267,-0.0407457312901538,
-1.16365));
#30121=CARTESIAN_POINT('Ctrl Pts',(0.223839179533421,-0.0442657206832852,
-1.16365));
#30122=CARTESIAN_POINT('Ctrl Pts',(0.222826740250488,-0.0477576124712794,
-1.16365));
#30123=CARTESIAN_POINT('Ctrl Pts',(0.218997816432901,-0.0609635279872651,
-1.16365));
#30124=CARTESIAN_POINT('Ctrl Pts',(0.213991911411158,-0.0738045735508588,
-1.16365));
#30125=CARTESIAN_POINT('Ctrl Pts',(0.207900422173151,-0.086131422481015,
-1.16365));
#30126=CARTESIAN_POINT('Ctrl Pts',(0.202431471973834,-0.0971984900369931,
-1.16365));
#30127=CARTESIAN_POINT('Ctrl Pts',(0.196086562094324,-0.107851540751618,
-1.16365));
#30128=CARTESIAN_POINT('Ctrl Pts',(0.188909537892742,-0.117965068595534,
-1.16365));
#30129=CARTESIAN_POINT('Ctrl Pts',(0.186465674632955,-0.121408846745137,
-1.16365));
#30130=CARTESIAN_POINT('Ctrl Pts',(0.183929867562409,-0.124783110870494,
-1.16365));
#30131=CARTESIAN_POINT('Ctrl Pts',(0.181307798655181,-0.128079381800206,
-1.16365));
#30132=CARTESIAN_POINT('Ctrl Pts',(0.172609817251073,-0.139013840147387,
-1.16365));
#30133=CARTESIAN_POINT('Ctrl Pts',(0.162954416545594,-0.149107860965651,
-1.16365));
#30134=CARTESIAN_POINT('Ctrl Pts',(0.152416199398516,-0.158186984131325,
-1.16365));
#30135=CARTESIAN_POINT('Ctrl Pts',(0.144286167596249,-0.165191352995949,
-1.16365));
#30136=CARTESIAN_POINT('Ctrl Pts',(0.135629842554803,-0.17159127125675,
-1.16365));
#30137=CARTESIAN_POINT('Ctrl Pts',(0.126471106027295,-0.177287929553122,
-1.16365));
#30138=CARTESIAN_POINT('Origin',(0.,0.,-1.16365));
#30139=CARTESIAN_POINT('Origin',(0.,0.,-1.25608093797092));
#30140=CARTESIAN_POINT('Ctrl Pts',(0.126471106027295,-0.177287929553122,
-1.16365));
#30141=CARTESIAN_POINT('Ctrl Pts',(0.185290142270931,-0.135328453868889,
-1.16100984835807));
#30142=CARTESIAN_POINT('Ctrl Pts',(0.25689562471139,0.0109872606886212,
-1.15572954507421));
#30143=CARTESIAN_POINT('Ctrl Pts',(0.130348081000917,0.221923062878552,
-1.14780909014843));
#30144=CARTESIAN_POINT('Ctrl Pts',(-0.115118491958846,0.229917045457789,
-1.13988863522264));
#30145=CARTESIAN_POINT('Ctrl Pts',(-0.214016587705737,0.0882349264091937,
-1.13431258449681));
#30146=CARTESIAN_POINT('Ctrl Pts',(-0.218077155627143,0.00821599845413173,
-1.1313766854129));
#30147=CARTESIAN_POINT('Ctrl Pts',(-0.21801873929181,0.000148950382043584,
-1.13108093797092));
#30148=CARTESIAN_POINT('Ctrl Pts',(0.143065810904944,-0.200550483046316,
-1.18014778394209));
#30149=CARTESIAN_POINT('Ctrl Pts',(0.209602693369046,-0.153085361545635,
-1.17750763230016));
#30150=CARTESIAN_POINT('Ctrl Pts',(0.290603775215938,0.0124289366118328,
-1.17222732901631));
#30151=CARTESIAN_POINT('Ctrl Pts',(0.147451496978881,0.251042344346831,
-1.16430687409052));
#30152=CARTESIAN_POINT('Ctrl Pts',(-0.13022358165107,0.260085244626455,
-1.15638641916474));
#30153=CARTESIAN_POINT('Ctrl Pts',(-0.28913528563414,0.0324272013455538,
-1.14846596423895));
#30154=CARTESIAN_POINT('Ctrl Pts',(-0.184526815942454,-0.22498267491905,
-1.14054550931316));
#30155=CARTESIAN_POINT('Ctrl Pts',(0.0882987842694294,-0.277214481409077,
-1.13262505438738));
#30156=CARTESIAN_POINT('Ctrl Pts',(0.28062920438186,-0.0768131084218392,
-1.12470459946159));
#30157=CARTESIAN_POINT('Ctrl Pts',(0.217165088152307,0.193633152740157,
-1.11678414453581));
#30158=CARTESIAN_POINT('Ctrl Pts',(-0.0442519673101072,0.287563995963539,
-1.10886368961002));
#30159=CARTESIAN_POINT('Ctrl Pts',(-0.265331129903845,0.119382148576781,
-1.10094323468424));
#30160=CARTESIAN_POINT('Ctrl Pts',(-0.244556208400208,-0.157623085138064,
-1.09302277975845));
#30161=CARTESIAN_POINT('Ctrl Pts',(-0.000862913917304123,-0.290949477759334,
-1.08510232483266));
#30162=CARTESIAN_POINT('Ctrl Pts',(0.243616752571797,-0.15907058057088,
-1.07718186990688));
#30163=CARTESIAN_POINT('Ctrl Pts',(0.266034844651534,0.117805017487398,
-1.06926141498109));
#30164=CARTESIAN_POINT('Ctrl Pts',(0.0459566567534106,0.287298606742041,
-1.0613409600553));
#30165=CARTESIAN_POINT('Ctrl Pts',(-0.216011940049781,0.19491377884898,
-1.05342050512952));
#30166=CARTESIAN_POINT('Ctrl Pts',(-0.281081230017808,-0.0751390504041708,
-1.04550005020373));
#30167=CARTESIAN_POINT('Ctrl Pts',(-0.0899391959740744,-0.276701045494272,
-1.03757959527795));
#30168=CARTESIAN_POINT('Ctrl Pts',(0.183184259020086,-0.22604437666544,
-1.02965914035216));
#30169=CARTESIAN_POINT('Ctrl Pts',(0.289331500349707,0.0306563985282065,
-1.02173868542638));
#30170=CARTESIAN_POINT('Ctrl Pts',(0.131747133363499,0.259413229903282,
-1.01381823050059));
#30171=CARTESIAN_POINT('Ctrl Pts',(-0.145927451972247,0.25170957582738,
-1.0058977755748));
#30172=CARTESIAN_POINT('Ctrl Pts',(-0.290586166915714,0.014567469894556,
-0.997977320649018));
#30173=CARTESIAN_POINT('Ctrl Pts',(-0.170369620154127,-0.235853183175507,
-0.990056865723232));
#30174=CARTESIAN_POINT('Ctrl Pts',(0.105142335713471,-0.27128881444409,
-0.982136410797447));
#30175=CARTESIAN_POINT('Ctrl Pts',(0.284814892364508,-0.0594391171641165,
-0.97421595587166));
#30176=CARTESIAN_POINT('Ctrl Pts',(0.204872822781333,0.206590556507594,
-0.966295500945875));
#30177=CARTESIAN_POINT('Ctrl Pts',(-0.0618150340809172,0.284308693378328,
-0.958375046020089));
#30178=CARTESIAN_POINT('Ctrl Pts',(-0.272157217330499,0.102873614775734,
-0.950454591094303));
#30179=CARTESIAN_POINT('Ctrl Pts',(-0.234422505225032,-0.172332877320268,
-0.942534136168517));
#30180=CARTESIAN_POINT('Ctrl Pts',(0.0169931368468682,-0.290454410990472,
-0.934613681242732));
#30181=CARTESIAN_POINT('Ctrl Pts',(0.25291918554204,-0.143820781347327,
-0.926693226316945));
#30182=CARTESIAN_POINT('Ctrl Pts',(0.258304200125824,0.133908445439324,
-0.918772771391161));
#30183=CARTESIAN_POINT('Ctrl Pts',(0.0282396291651197,0.289577372920495,
-0.910852316465373));
#30184=CARTESIAN_POINT('Ctrl Pts',(-0.227565943992463,0.181290575313672,
-0.902931861539589));
#30185=CARTESIAN_POINT('Ctrl Pts',(-0.275940483620407,-0.0922463064956857,
-0.895011406613801));
#30186=CARTESIAN_POINT('Ctrl Pts',(-0.0727896029424237,-0.281698784637569,
-0.887090951688017));
#30187=CARTESIAN_POINT('Ctrl Pts',(0.196710496356156,-0.2143770327859,-0.87917049676223));
#30188=CARTESIAN_POINT('Ctrl Pts',(0.286904936603112,0.0483537890505052,
-0.871250041836445));
#30189=CARTESIAN_POINT('Ctrl Pts',(0.115579632374212,0.267009138688217,
-0.863329586910658));
#30190=CARTESIAN_POINT('Ctrl Pts',(-0.16109888146827,0.242280172429462,
-0.855409131984874));
#30191=CARTESIAN_POINT('Ctrl Pts',(-0.290932454907336,-0.00329214889838965,
-0.847488677059086));
#30192=CARTESIAN_POINT('Ctrl Pts',(-0.155575118186665,-0.245863608864721,
-0.839568222133302));
#30193=CARTESIAN_POINT('Ctrl Pts',(0.121592135214742,-0.264325337825753,
-0.831647767207515));
#30194=CARTESIAN_POINT('Ctrl Pts',(0.287925659130265,-0.0418490905179701,
-0.823727312281731));
#30195=CARTESIAN_POINT('Ctrl Pts',(0.191809029014613,0.218773462630297,
-0.815806857355942));
#30196=CARTESIAN_POINT('Ctrl Pts',(-0.0791454719650589,0.279979509661344,
-0.807886402430158));
#30197=CARTESIAN_POINT('Ctrl Pts',(-0.277957249122045,0.0859784811640934,
-0.799965947504372));
#30198=CARTESIAN_POINT('Ctrl Pts',(-0.223405282781762,-0.186393699432088,
-0.792045492578585));
#30199=CARTESIAN_POINT('Ctrl Pts',(0.0347851889093908,-0.288864193342333,
-0.784125037652801));
#30200=CARTESIAN_POINT('Ctrl Pts',(0.26126824621153,-0.128029040003937,
-0.776204582727013));
#30201=CARTESIAN_POINT('Ctrl Pts',(0.249599929062365,0.149507213788637,
-0.76828412780123));
#30202=CARTESIAN_POINT('Ctrl Pts',(0.0104161482811412,0.290764570430725,
-0.760363672875442));
#30203=CARTESIAN_POINT('Ctrl Pts',(-0.238262165669008,0.166984047062865,
-0.752443217949657));
#30204=CARTESIAN_POINT('Ctrl Pts',(-0.269759620266356,-0.109005866064766,
-0.744522763023871));
#30205=CARTESIAN_POINT('Ctrl Pts',(-0.0553656384972611,-0.285634692634787,
-0.736602308098084));
#30206=CARTESIAN_POINT('Ctrl Pts',(0.209495260307064,-0.201901628204565,
-0.7286818531723));
#30207=CARTESIAN_POINT('Ctrl Pts',(0.28339692504217,0.0658689186143308,
-0.720761398246513));
#30208=CARTESIAN_POINT('Ctrl Pts',(0.0989764699149806,0.273598592770407,
-0.712840943320728));
#30209=CARTESIAN_POINT('Ctrl Pts',(-0.17566307111485,0.231937528246891,
-0.704920488394942));
#30210=CARTESIAN_POINT('Ctrl Pts',(-0.290182113641896,-0.0211393586728707,
-0.697000033469155));
#30211=CARTESIAN_POINT('Ctrl Pts',(-0.140194197489197,-0.25494728583207,
-0.689079578543371));
#30212=CARTESIAN_POINT('Ctrl Pts',(0.137583610111387,-0.256365523796583,
-0.681159123617583));
#30213=CARTESIAN_POINT('Ctrl Pts',(0.289951130296208,-0.0241013195225775,
-0.673238668691798));
#30214=CARTESIAN_POINT('Ctrl Pts',(0.178022237866677,0.230131732683084,
-0.665318213766013));
#30215=CARTESIAN_POINT('Ctrl Pts',(-0.0961775820314826,0.274594982250872,
-0.657397758840226));
#30216=CARTESIAN_POINT('Ctrl Pts',(-0.282709559838887,0.0687592636557534,
-0.649477303914441));
#30217=CARTESIAN_POINT('Ctrl Pts',(-0.211545965289424,-0.199751936492601,
-0.641556848988655));
#30218=CARTESIAN_POINT('Ctrl Pts',(0.052446123054555,-0.286185142415403,
-0.633636394062869));
#30219=CARTESIAN_POINT('Ctrl Pts',(0.268632492673834,-0.111754711053366,
-0.625715939137084));
#30220=CARTESIAN_POINT('Ctrl Pts',(0.239954825885267,0.16454243555129,-0.617795484211296));
#30221=CARTESIAN_POINT('Ctrl Pts',(-0.00744659482069732,0.290855771454435,
-0.609875029285512));
#30222=CARTESIAN_POINT('Ctrl Pts',(-0.248060291349511,0.152048095740703,
-0.601954574359725));
#30223=CARTESIAN_POINT('Ctrl Pts',(-0.262561935655004,-0.125354543227901,
-0.594034119433939));
#30224=CARTESIAN_POINT('Ctrl Pts',(-0.0377329810012622,-0.288493940504021,
-0.586113664508154));
#30225=CARTESIAN_POINT('Ctrl Pts',(0.221490361098709,-0.18866518360085,
-0.578193209582367));
#30226=CARTESIAN_POINT('Ctrl Pts',(0.278820688305979,0.0831357644781028,
-0.570272754656583));
#30227=CARTESIAN_POINT('Ctrl Pts',(0.0820002294595659,0.279156755123992,
-0.562352299730795));
#30228=CARTESIAN_POINT('Ctrl Pts',(-0.189565123319758,0.220720627906736,
-0.554431844805011));
#30229=CARTESIAN_POINT('Ctrl Pts',(-0.288337971379312,-0.038906886583765,
-0.546511389879224));
#30230=CARTESIAN_POINT('Ctrl Pts',(-0.124284834321296,-0.263069974570467,
-0.538590934953439));
#30231=CARTESIAN_POINT('Ctrl Pts',(0.153056482782545,-0.247439375688298,
-0.530670480027653));
#30232=CARTESIAN_POINT('Ctrl Pts',(0.290883671124509,-0.00626270196536656,
-0.522750025101867));
#30233=CARTESIAN_POINT('Ctrl Pts',(0.163564416727095,0.240622553272764,
-0.514829570176081));
#30234=CARTESIAN_POINT('Ctrl Pts',(-0.112847164119155,0.268175407360637,
-0.506909115250295));
#30235=CARTESIAN_POINT('Ctrl Pts',(-0.286396236307729,0.0512808676949378,
-0.498988660324509));
#30236=CARTESIAN_POINT('Ctrl Pts',(-0.198889254791463,-0.212357236493779,
-0.491068205398723));
#30237=CARTESIAN_POINT('Ctrl Pts',(0.0699093688550693,-0.282427356516795,
-0.483147750472938));
#30238=CARTESIAN_POINT('Ctrl Pts',(0.274984166429074,-0.0950591383091926,
-0.475227295547151));
#30239=CARTESIAN_POINT('Ctrl Pts',(0.229405246465546,0.178957437556701,
-0.467306840621366));
#30240=CARTESIAN_POINT('Ctrl Pts',(-0.0252812690221513,0.289850632221853,
-0.459386385695579));
#30241=CARTESIAN_POINT('Ctrl Pts',(-0.256923388366033,0.136539020332266,
-0.451465930769795));
#30242=CARTESIAN_POINT('Ctrl Pts',(-0.254374560454433,-0.141230713927224,
-0.443545475844008));
#30243=CARTESIAN_POINT('Ctrl Pts',(-0.0199580942971045,-0.290265750709254,
-0.435625020918223));
#30244=CARTESIAN_POINT('Ctrl Pts',(0.232650584871963,-0.17471759190623,
-0.427704565992436));
#30245=CARTESIAN_POINT('Ctrl Pts',(0.273193475880536,0.100089241675063,
-0.419784111066651));
#30246=CARTESIAN_POINT('Ctrl Pts',(0.0647149005781834,0.283662675031338,
-0.411863656140865));
#30247=CARTESIAN_POINT('Ctrl Pts',(-0.202752636236533,0.208671751950079,
-0.403943201215079));
#30248=CARTESIAN_POINT('Ctrl Pts',(-0.285406979356585,-0.0565277604131661,
-0.396022746289293));
#30249=CARTESIAN_POINT('Ctrl Pts',(-0.107906996808085,-0.270201057737822,
-0.388102291363507));
#30250=CARTESIAN_POINT('Ctrl Pts',(0.16795243039314,-0.237580539371001,
-0.380181836437721));
#30251=CARTESIAN_POINT('Ctrl Pts',(0.290719766532602,0.0115995219732621,
-0.372261381511936));
#30252=CARTESIAN_POINT('Ctrl Pts',(0.148490062335797,0.250206380714582,
-0.364340926586149));
#30253=CARTESIAN_POINT('Ctrl Pts',(-0.129091384563791,0.260744982682662,
-0.356420471660364));
#30254=CARTESIAN_POINT('Ctrl Pts',(-0.28900338211591,0.033609175656999,
-0.348500016734578));
#30255=CARTESIAN_POINT('Ctrl Pts',(-0.185482858992497,-0.224162085515702,
-0.340579561808792));
#30256=CARTESIAN_POINT('Ctrl Pts',(0.0871091010420014,-0.27760500009624,
-0.332659106883006));
#30257=CARTESIAN_POINT('Ctrl Pts',(0.280299325729081,-0.0780052534038562,
-0.32473865195722));
#30258=CARTESIAN_POINT('Ctrl Pts',(0.217990955971174,0.192697884465696,
-0.316818197031434));
#30259=CARTESIAN_POINT('Ctrl Pts',(-0.0430206490067566,0.287752941465094,
-0.308897742105649));
#30260=CARTESIAN_POINT('Ctrl Pts',(-0.264818048510752,0.120515280133804,
-0.300977287179863));
#30261=CARTESIAN_POINT('Ctrl Pts',(-0.245228355833355,-0.156574535152013,
-0.293056832254077));
#30262=CARTESIAN_POINT('Ctrl Pts',(-0.00210797834057768,-0.290943444659053,
-0.285136377328291));
#30263=CARTESIAN_POINT('Ctrl Pts',(0.242933864720045,-0.160111426621978,
-0.277215922402505));
#30264=CARTESIAN_POINT('Ctrl Pts',(0.266536498758302,0.116665446438031,
-0.26929546747672));
#30265=CARTESIAN_POINT('Ctrl Pts',(0.0471856379063532,0.287099368055711,
-0.261375012550933));
#30266=CARTESIAN_POINT('Ctrl Pts',(-0.215175901374109,0.195836316934433,
-0.253454557625148));
#30267=CARTESIAN_POINT('Ctrl Pts',(-0.281400185540743,-0.0739355607360446,
-0.245534102699361));
#30268=CARTESIAN_POINT('Ctrl Pts',(-0.0911224189205789,-0.276313655709459,
-0.237613647773576));
#30269=CARTESIAN_POINT('Ctrl Pts',(0.182215304741336,-0.22682617635566,
-0.229693192847789));
#30270=CARTESIAN_POINT('Ctrl Pts',(0.289460034346049,0.0294180231372127,
-0.221772737922004));
#30271=CARTESIAN_POINT('Ctrl Pts',(0.132855995349668,0.258847090097914,
-0.213852282996218));
#30272=CARTESIAN_POINT('Ctrl Pts',(-0.144849013006134,0.252331716185271,
-0.205931828070432));
#30273=CARTESIAN_POINT('Ctrl Pts',(-0.29052117006007,0.0158107984837069,
-0.198011373144647));
#30274=CARTESIAN_POINT('Ctrl Pts',(-0.171377311300073,-0.23512198675802,
-0.19009091821886));
#30275=CARTESIAN_POINT('Ctrl Pts',(0.103980487374873,-0.271736250484141,
-0.182170463293075));
#30276=CARTESIAN_POINT('Ctrl Pts',(0.284557936296122,-0.0606573383293682,
-0.174250008367289));
#30277=CARTESIAN_POINT('Ctrl Pts',(0.205754978077643,0.205711983108962,
-0.166329553441503));
#30278=CARTESIAN_POINT('Ctrl Pts',(-0.0605978669457687,0.284570607032695,
-0.158409098515717));
#30279=CARTESIAN_POINT('Ctrl Pts',(-0.271714517213715,0.104037272696485,
-0.150488643589931));
#30280=CARTESIAN_POINT('Ctrl Pts',(-0.235157790958593,-0.17132816727427,
-0.142568188664145));
#30281=CARTESIAN_POINT('Ctrl Pts',(0.0157500716120863,-0.290524474026164,
-0.13464773373836));
#30282=CARTESIAN_POINT('Ctrl Pts',(0.252301461550156,-0.14490173197348,
-0.126727278812573));
#30283=CARTESIAN_POINT('Ctrl Pts',(0.258874807121329,0.132801874887983,
-0.118806823886788));
#30284=CARTESIAN_POINT('Ctrl Pts',(0.0294785960508995,0.289453922220514,
-0.110886368961002));
#30285=CARTESIAN_POINT('Ctrl Pts',(-0.226788243918246,0.182262624136886,
-0.102965914035216));
#30286=CARTESIAN_POINT('Ctrl Pts',(-0.276332402362021,-0.09106451907133,
-0.09504545910943));
#30287=CARTESIAN_POINT('Ctrl Pts',(-0.0739949199882418,-0.281385017105497,
-0.0871250041836446));
#30288=CARTESIAN_POINT('Ctrl Pts',(0.195792393150789,-0.215216274196785,
-0.0792045492578584));
#30289=CARTESIAN_POINT('Ctrl Pts',(0.287107229299654,0.0471245930402426,
-0.0712840943320728));
#30290=CARTESIAN_POINT('Ctrl Pts',(0.116724934327384,0.266514095421913,
-0.0633636394062869));
#30291=CARTESIAN_POINT('Ctrl Pts',(-0.160067851115533,0.242963550798627,
-0.0554431844805008));
#30292=CARTESIAN_POINT('Ctrl Pts',(-0.290930201862917,-0.00204001234416272,
-0.0475227295547152));
#30293=CARTESIAN_POINT('Ctrl Pts',(-0.156651773764553,-0.245209240429496,
-0.0396022746289292));
#30294=CARTESIAN_POINT('Ctrl Pts',(0.120509367727107,-0.264817350405622,
-0.0316818197031433));
#30295=CARTESIAN_POINT('Ctrl Pts',(0.287649633879381,-0.0431300802166473,
-0.0237613647773576));
#30296=CARTESIAN_POINT('Ctrl Pts',(0.192925896622358,0.218045410474343,
-0.0158409098515715));
#30297=CARTESIAN_POINT('Ctrl Pts',(-0.0783209863033229,0.280126499531071,
-0.00792045492578587));
#30298=CARTESIAN_POINT('Ctrl Pts',(-0.21054802840921,0.151782557364509,
-0.0026401516419286));
#30299=CARTESIAN_POINT('Ctrl Pts',(-0.235034375322676,0.0738049111962042,
0.));
#30300=CARTESIAN_POINT('Ctrl Pts',(0.137534242612394,-0.192796298548585,
-1.17464852262806));
#30301=CARTESIAN_POINT('Ctrl Pts',(0.201498509669674,-0.147166392320053,
-1.17200837098613));
#30302=CARTESIAN_POINT('Ctrl Pts',(0.279367725047756,0.0119483779707621,
-1.16672806770228));
#30303=CARTESIAN_POINT('Ctrl Pts',(0.14175035831956,0.241335917190738,-1.15880761277649));
#30304=CARTESIAN_POINT('Ctrl Pts',(-0.125188551753662,0.250029178236899,
-1.15088715785071));
#30305=CARTESIAN_POINT('Ctrl Pts',(-0.277956013883926,0.0311734197631856,
-1.14296670292492));
#30306=CARTESIAN_POINT('Ctrl Pts',(-0.177392178549103,-0.216283831896505,
-1.13504624799913));
#30307=CARTESIAN_POINT('Ctrl Pts',(0.0848847557727121,-0.266496121614389,
-1.12712579307335));
#30308=CARTESIAN_POINT('Ctrl Pts',(0.269778816024899,-0.0738431678587459,
-1.11920533814756));
#30309=CARTESIAN_POINT('Ctrl Pts',(0.208768508226792,0.186146423371982,
-1.11128488322178));
#30310=CARTESIAN_POINT('Ctrl Pts',(-0.0425409870437026,0.276445477345505,
-1.10336442829599));
#30311=CARTESIAN_POINT('Ctrl Pts',(-0.255072233973931,0.114766297287177,
-1.09544397337021));
#30312=CARTESIAN_POINT('Ctrl Pts',(-0.235100564458613,-0.151528667090814,
-1.08752351844442));
#30313=CARTESIAN_POINT('Ctrl Pts',(-0.000829549780659682,-0.279700061174566,
-1.07960306351863));
#30314=CARTESIAN_POINT('Ctrl Pts',(0.2341974322217,-0.152920195833971,-1.07168260859285));
#30315=CARTESIAN_POINT('Ctrl Pts',(0.255748739941544,0.11325014518552,-1.06376215366706));
#30316=CARTESIAN_POINT('Ctrl Pts',(0.0441797655190845,0.27619034926602,
-1.05584169874127));
#30317=CARTESIAN_POINT('Ctrl Pts',(-0.207659946021065,0.187377534710411,
-1.04792124381549));
#30318=CARTESIAN_POINT('Ctrl Pts',(-0.270213364314866,-0.0722338364601898,
-1.0400007888897));
#30319=CARTESIAN_POINT('Ctrl Pts',(-0.0864617417761726,-0.266002537443397,
-1.03208033396392));
#30320=CARTESIAN_POINT('Ctrl Pts',(0.176101530921177,-0.217304483473891,
-1.02415987903813));
#30321=CARTESIAN_POINT('Ctrl Pts',(0.278144642055285,0.0294710841544246,
-1.01623942411235));
#30322=CARTESIAN_POINT('Ctrl Pts',(0.126653196098277,0.24938314662815,-1.00831896918656));
#30323=CARTESIAN_POINT('Ctrl Pts',(-0.140285239753713,0.241977350498556,
-1.00039851426077));
#30324=CARTESIAN_POINT('Ctrl Pts',(-0.279350797563686,0.0140042259296867,
-0.992478059334987));
#30325=CARTESIAN_POINT('Ctrl Pts',(-0.163782363681758,-0.226734037367727,
-0.984557604409201));
#30326=CARTESIAN_POINT('Ctrl Pts',(0.101077059692887,-0.260799567609992,
-0.976637149483415));
#30327=CARTESIAN_POINT('Ctrl Pts',(0.273802666467321,-0.0571409333159812,
-0.968716694557631));
#30328=CARTESIAN_POINT('Ctrl Pts',(0.19695151717146,0.198602835579099,-0.960796239631843));
#30329=CARTESIAN_POINT('Ctrl Pts',(-0.059424986589053,0.273316039412716,
-0.952875784706058));
#30330=CARTESIAN_POINT('Ctrl Pts',(-0.261634394131502,0.0988960577197611,
-0.944955329780273));
#30331=CARTESIAN_POINT('Ctrl Pts',(-0.225358675867337,-0.165669712487812,
-0.937034874854486));
#30332=CARTESIAN_POINT('Ctrl Pts',(0.0163361056779362,-0.279224135915642,
-0.9291144199287));
#30333=CARTESIAN_POINT('Ctrl Pts',(0.243140191256317,-0.138260022498806,
-0.921193965002915));
#30334=CARTESIAN_POINT('Ctrl Pts',(0.248316996934436,0.128730942119617,
-0.913273510077128));
#30335=CARTESIAN_POINT('Ctrl Pts',(0.027147757974546,0.278381008085635,
-0.905353055151344));
#30336=CARTESIAN_POINT('Ctrl Pts',(-0.218767220158372,0.174281065551697,
-0.897432600225556));
#30337=CARTESIAN_POINT('Ctrl Pts',(-0.265271382315417,-0.0886796490190409,
-0.889512145299772));
#30338=CARTESIAN_POINT('Ctrl Pts',(-0.0699752292138806,-0.270807041492966,
-0.881591690373984));
#30339=CARTESIAN_POINT('Ctrl Pts',(0.189104783030431,-0.206088251631909,
-0.8736712354482));
#30340=CARTESIAN_POINT('Ctrl Pts',(0.275811900186857,0.0464842138903423,
-0.865750780522412));
#30341=CARTESIAN_POINT('Ctrl Pts',(0.111110803478883,0.256685363384765,
-0.857830325596628));
#30342=CARTESIAN_POINT('Ctrl Pts',(-0.154870073487814,0.232912530284584,
-0.849909870670842));
#30343=CARTESIAN_POINT('Ctrl Pts',(-0.279683696502658,-0.00316485960162851,
-0.841989415745056));
#30344=CARTESIAN_POINT('Ctrl Pts',(-0.14955988376114,-0.23635741493561,
-0.834068960819269));
#30345=CARTESIAN_POINT('Ctrl Pts',(0.116890835892962,-0.254105330345378,
-0.826148505893485));
#30346=CARTESIAN_POINT('Ctrl Pts',(0.276793156986097,-0.0402310162854403,
-0.818228050967698));
#30347=CARTESIAN_POINT('Ctrl Pts',(0.184392828481371,0.210314695707002,
-0.810307596041912));
#30348=CARTESIAN_POINT('Ctrl Pts',(-0.0760853517277248,0.269154241427026,
-0.802387141116127));
#30349=CARTESIAN_POINT('Ctrl Pts',(-0.267210170583837,0.0826541660307953,
-0.794466686190341));
#30350=CARTESIAN_POINT('Ctrl Pts',(-0.21476742884023,-0.179186879918832,
-0.786546231264554));
#30351=CARTESIAN_POINT('Ctrl Pts',(0.0334402369127925,-0.277695403240503,
-0.77862577633877));
#30352=CARTESIAN_POINT('Ctrl Pts',(0.251166439655148,-0.123078860965831,
-0.770705321412982));
#30353=CARTESIAN_POINT('Ctrl Pts',(0.239949272174526,0.143726591863178,
-0.762784866487197));
#30354=CARTESIAN_POINT('Ctrl Pts',(0.010013413097955,0.279522303195683,
-0.754864411561412));
#30355=CARTESIAN_POINT('Ctrl Pts',(-0.229049877753451,0.160527692087124,
-0.746943956635625));
#30356=CARTESIAN_POINT('Ctrl Pts',(-0.259329498963182,-0.10479120856825,
-0.73902350170984));
#30357=CARTESIAN_POINT('Ctrl Pts',(-0.0532249536720674,-0.274590769568636,
-0.731103046784054));
#30358=CARTESIAN_POINT('Ctrl Pts',(0.201395230453503,-0.194095202352532,
-0.723182591858267));
#30359=CARTESIAN_POINT('Ctrl Pts',(0.272439524144964,0.0633221296969308,
-0.715262136932483));
#30360=CARTESIAN_POINT('Ctrl Pts',(0.0951495940231997,0.263020039508227,
-0.707341682006696));
#30361=CARTESIAN_POINT('Ctrl Pts',(-0.168871145998678,0.222969779285854,
-0.69942122708091));
#30362=CARTESIAN_POINT('Ctrl Pts',(-0.278962366808371,-0.0203220159029941,
-0.691500772155125));
#30363=CARTESIAN_POINT('Ctrl Pts',(-0.134773658698514,-0.245089876059184,
-0.683580317229338));
#30364=CARTESIAN_POINT('Ctrl Pts',(0.132264008380877,-0.246453278559472,
-0.675659862303554));
#30365=CARTESIAN_POINT('Ctrl Pts',(0.278740314318651,-0.0231694540123176,
-0.667739407377766));
#30366=CARTESIAN_POINT('Ctrl Pts',(0.171139096743559,0.221233803907739,
-0.659818952451982));
#30367=CARTESIAN_POINT('Ctrl Pts',(-0.0924589237451018,0.263977904085905,
-0.651898497526195));
#30368=CARTESIAN_POINT('Ctrl Pts',(-0.27177873557477,0.0661007209875132,
-0.643978042600409));
#30369=CARTESIAN_POINT('Ctrl Pts',(-0.203366645949535,-0.192028627399474,
-0.636057587674623));
#30370=CARTESIAN_POINT('Ctrl Pts',(0.0504183198392325,-0.27511993648276,
-0.628137132748838));
#30371=CARTESIAN_POINT('Ctrl Pts',(0.258245951197406,-0.107433770835046,
-0.620216677823051));
#30372=CARTESIAN_POINT('Ctrl Pts',(0.230677092105858,0.158180484268051,
-0.612296222897266));
#30373=CARTESIAN_POINT('Ctrl Pts',(-0.00715867594240549,0.279609977977254,
-0.604375767971481));
#30374=CARTESIAN_POINT('Ctrl Pts',(-0.238469163786677,0.146169231880625,
-0.596455313045694));
#30375=CARTESIAN_POINT('Ctrl Pts',(-0.252410109240903,-0.120507772275005,
-0.588534858119908));
#30376=CARTESIAN_POINT('Ctrl Pts',(-0.0362740540922425,-0.277339466043697,
-0.580614403194122));
#30377=CARTESIAN_POINT('Ctrl Pts',(0.212926546649896,-0.181370538284032,
-0.572693948268336));
#30378=CARTESIAN_POINT('Ctrl Pts',(0.268040225321954,0.0799213615690144,
-0.564773493342551));
#30379=CARTESIAN_POINT('Ctrl Pts',(0.0788297314461609,0.268363298283903,
-0.556853038416765));
#30380=CARTESIAN_POINT('Ctrl Pts',(-0.182235682282126,0.212186574808252,
-0.548932583490979));
#30381=CARTESIAN_POINT('Ctrl Pts',(-0.277189527387479,-0.0374025712003252,
-0.541012128565193));
#30382=CARTESIAN_POINT('Ctrl Pts',(-0.119479423130266,-0.252898505084842,
-0.533091673639407));
#30383=CARTESIAN_POINT('Ctrl Pts',(0.147138630139948,-0.237872255520119,
-0.525171218713621));
#30384=CARTESIAN_POINT('Ctrl Pts',(0.279636798920486,-0.00602055771442263,
-0.517250763787836));
#30385=CARTESIAN_POINT('Ctrl Pts',(0.157240280054371,0.23131900214663,-0.509330308862049));
#30386=CARTESIAN_POINT('Ctrl Pts',(-0.108483984747388,0.257806538860088,
-0.501409853936264));
#30387=CARTESIAN_POINT('Ctrl Pts',(-0.275322868534921,0.0492981184974779,
-0.493489399010478));
#30388=CARTESIAN_POINT('Ctrl Pts',(-0.191199300856458,-0.204146549757009,
-0.485568944084692));
#30389=CARTESIAN_POINT('Ctrl Pts',(0.0672063579423657,-0.271507443503511,
-0.477648489158906));
#30390=CARTESIAN_POINT('Ctrl Pts',(0.264352040651778,-0.0913837240920417,
-0.46972803423312));
#30391=CARTESIAN_POINT('Ctrl Pts',(0.220535406917812,0.172038137403554,
-0.461807579307335));
#30392=CARTESIAN_POINT('Ctrl Pts',(-0.0243037813524294,0.278643701952265,
-0.453887124381548));
#30393=CARTESIAN_POINT('Ctrl Pts',(-0.246989573573313,0.131259807145073,
-0.445966669455763));
#30394=CARTESIAN_POINT('Ctrl Pts',(-0.244539294822899,-0.135770098744935,
-0.438046214529977));
#30395=CARTESIAN_POINT('Ctrl Pts',(-0.0191864245257226,-0.279042770090194,
-0.430125759604191));
#30396=CARTESIAN_POINT('Ctrl Pts',(0.223655265931815,-0.16796222327255,
-0.422205304678406));
#30397=CARTESIAN_POINT('Ctrl Pts',(0.262630586261044,0.0962193410176438,
-0.414284849752619));
#30398=CARTESIAN_POINT('Ctrl Pts',(0.0622127311931329,0.272694999043218,
-0.406364394826833));
#30399=CARTESIAN_POINT('Ctrl Pts',(-0.194913306582979,0.200603562636807,
-0.398443939901048));
#30400=CARTESIAN_POINT('Ctrl Pts',(-0.274371860710872,-0.0543421427231499,
-0.390523484975262));
#30401=CARTESIAN_POINT('Ctrl Pts',(-0.103734826543839,-0.259753868474771,
-0.382603030049476));
#30402=CARTESIAN_POINT('Ctrl Pts',(0.161458633358455,-0.228394606196619,
-0.37468257512369));
#30403=CARTESIAN_POINT('Ctrl Pts',(0.279479231617956,0.0111510322359151,
-0.366762120197904));
#30404=CARTESIAN_POINT('Ctrl Pts',(0.142748768064441,0.24053227567579,-0.358841665272119));
#30405=CARTESIAN_POINT('Ctrl Pts',(-0.124100130502618,0.250663407849894,
-0.350921210346332));
#30406=CARTESIAN_POINT('Ctrl Pts',(-0.277829210349505,0.0323096936268268,
-0.343000755420547));
#30407=CARTESIAN_POINT('Ctrl Pts',(-0.178311256670989,-0.215494970173559,
-0.33508030049476));
#30408=CARTESIAN_POINT('Ctrl Pts',(0.0837410710544831,-0.266871541091098,
-0.327159845568975));
#30409=CARTESIAN_POINT('Ctrl Pts',(0.26946169196586,-0.074989219149049,
-0.319239390643189));
#30410=CARTESIAN_POINT('Ctrl Pts',(0.209562444277951,0.185247316779332,
-0.311318935717403));
#30411=CARTESIAN_POINT('Ctrl Pts',(-0.0413572770490159,0.276627117363389,
-0.303398480791617));
#30412=CARTESIAN_POINT('Ctrl Pts',(-0.254578990617248,0.115855616877159,
-0.295478025865831));
#30413=CARTESIAN_POINT('Ctrl Pts',(-0.235746723646171,-0.150520658767508,
-0.287557570940046));
#30414=CARTESIAN_POINT('Ctrl Pts',(-0.00202647440839203,-0.279694261341101,
-0.27963711601426));
#30415=CARTESIAN_POINT('Ctrl Pts',(0.233540947888471,-0.15392079809113,
-0.271716661088474));
#30416=CARTESIAN_POINT('Ctrl Pts',(0.256230997842236,0.112154635082958,
-0.263796206162688));
#30417=CARTESIAN_POINT('Ctrl Pts',(0.045361228728119,0.275998814044221,
-0.255875751236902));
#30418=CARTESIAN_POINT('Ctrl Pts',(-0.206856232364211,0.188264403320467,
-0.247955296311116));
#30419=CARTESIAN_POINT('Ctrl Pts',(-0.270519987581435,-0.0710768791204128,
-0.240034841385331));
#30420=CARTESIAN_POINT('Ctrl Pts',(-0.087599215997021,-0.265630125891588,
-0.232114386459544));
#30421=CARTESIAN_POINT('Ctrl Pts',(0.175170040776809,-0.218056055268639,
-0.224193931533759));
#30422=CARTESIAN_POINT('Ctrl Pts',(0.278268206348704,0.0282805899308719,
-0.216273476607973));
#30423=CARTESIAN_POINT('Ctrl Pts',(0.127719184488269,0.248838896336264,
-0.208353021682187));
#30424=CARTESIAN_POINT('Ctrl Pts',(-0.139248498092866,0.242575436109506,
-0.200432566756401));
#30425=CARTESIAN_POINT('Ctrl Pts',(-0.279288313779079,0.0151994818384572,
-0.192512111830616));
#30426=CARTESIAN_POINT('Ctrl Pts',(-0.164751092951653,-0.226031112295385,
-0.184591656904829));
#30427=CARTESIAN_POINT('Ctrl Pts',(0.099960133641381,-0.261229703758501,
-0.176671201979044));
#30428=CARTESIAN_POINT('Ctrl Pts',(0.273555645477285,-0.0583120525668871,
-0.168750747053258));
#30429=CARTESIAN_POINT('Ctrl Pts',(0.197799564372794,0.197758231783153,
-0.160830292127472));
#30430=CARTESIAN_POINT('Ctrl Pts',(-0.0582548806147009,0.273567826306141,
-0.152909837201686));
#30431=CARTESIAN_POINT('Ctrl Pts',(-0.261208810794147,0.100014723386828,
-0.1449893822759));
#30432=CARTESIAN_POINT('Ctrl Pts',(-0.226065532144383,-0.164703849055121,
-0.137068927350114));
#30433=CARTESIAN_POINT('Ctrl Pts',(0.0151411029410687,-0.27929148999897,
-0.129148472424328));
#30434=CARTESIAN_POINT('Ctrl Pts',(0.242546351254783,-0.139299178707609,
-0.121228017498542));
#30435=CARTESIAN_POINT('Ctrl Pts',(0.248865541694779,0.127667156567268,
-0.113307562572757));
#30436=CARTESIAN_POINT('Ctrl Pts',(0.0283388208230337,0.278262330545457,
-0.105387107646971));
#30437=CARTESIAN_POINT('Ctrl Pts',(-0.218019589470017,0.175215530591508,
-0.097466652721185));
#30438=CARTESIAN_POINT('Ctrl Pts',(-0.265648147714169,-0.0875435548165934,
-0.0895461977953989));
#30439=CARTESIAN_POINT('Ctrl Pts',(-0.0711339432767014,-0.270505405626179,
-0.0816257428696132));
#30440=CARTESIAN_POINT('Ctrl Pts',(0.188222177828032,-0.206895044191815,
-0.0737052879438272));
#30441=CARTESIAN_POINT('Ctrl Pts',(0.276006371337084,0.0453025441313394,
-0.0657848330180416));
#30442=CARTESIAN_POINT('Ctrl Pts',(0.112211822902711,0.256209460719685,
-0.0578643780922556));
#30443=CARTESIAN_POINT('Ctrl Pts',(-0.153878907409929,0.233569486169616,
-0.0499439231664696));
#30444=CARTESIAN_POINT('Ctrl Pts',(-0.279681530571079,-0.00196113628336259,
-0.042023468240684));
#30445=CARTESIAN_POINT('Ctrl Pts',(-0.15059491098758,-0.235728347329877,
-0.0341030133148979));
#30446=CARTESIAN_POINT('Ctrl Pts',(0.115849933070721,-0.254578319504005,
-0.0261825583891122));
#30447=CARTESIAN_POINT('Ctrl Pts',(0.276527804114002,-0.0414624771557032,
-0.0182621034633263));
#30448=CARTESIAN_POINT('Ctrl Pts',(0.18546651295957,0.209614793324889,-0.0103416485375403));
#30449=CARTESIAN_POINT('Ctrl Pts',(-0.0752927443932796,0.269295548006681,
-0.00242119361175462));
#30450=CARTESIAN_POINT('Ctrl Pts',(-0.202407293801547,0.145913960413436,
0.00285910967210262));
#30451=CARTESIAN_POINT('Ctrl Pts',(-0.225946888312534,0.0709512810799313,
0.00549926131403122));
#30452=CARTESIAN_POINT('Ctrl Pts',(0.132002674319845,-0.185042114050853,
-1.16914926131403));
#30453=CARTESIAN_POINT('Ctrl Pts',(0.193394325970303,-0.141247423094471,
-1.1665091096721));
#30454=CARTESIAN_POINT('Ctrl Pts',(0.268131674879573,0.0114678193296916,
-1.16122880638824));
#30455=CARTESIAN_POINT('Ctrl Pts',(0.136049219660238,0.231629490034645,
-1.15330835146246));
#30456=CARTESIAN_POINT('Ctrl Pts',(-0.120153521856254,0.239973111847344,
-1.14538789653667));
#30457=CARTESIAN_POINT('Ctrl Pts',(-0.266776742133712,0.0299196381808178,
-1.13746744161089));
#30458=CARTESIAN_POINT('Ctrl Pts',(-0.170257541155753,-0.207584988873961,
-1.1295469866851));
#30459=CARTESIAN_POINT('Ctrl Pts',(0.0814707272759947,-0.2557777618197,
-1.12162653175932));
#30460=CARTESIAN_POINT('Ctrl Pts',(0.258928427667939,-0.070873227295653,
-1.11370607683353));
#30461=CARTESIAN_POINT('Ctrl Pts',(0.200371928301276,0.178659694003806,
-1.10578562190774));
#30462=CARTESIAN_POINT('Ctrl Pts',(-0.0408300067772977,0.265326958727471,
-1.09786516698196));
#30463=CARTESIAN_POINT('Ctrl Pts',(-0.244813338044019,0.110150445997574,
-1.08994471205617));
#30464=CARTESIAN_POINT('Ctrl Pts',(-0.225644920517017,-0.145434249043564,
-1.08202425713039));
#30465=CARTESIAN_POINT('Ctrl Pts',(-0.000796185644015697,-0.268450644589798,
-1.0741038022046));
#30466=CARTESIAN_POINT('Ctrl Pts',(0.224778111871604,-0.146769811097062,
-1.06618334727881));
#30467=CARTESIAN_POINT('Ctrl Pts',(0.245462635231555,0.108695272883643,
-1.05826289235303));
#30468=CARTESIAN_POINT('Ctrl Pts',(0.0424028742847586,0.265082091789998,
-1.05034243742724));
#30469=CARTESIAN_POINT('Ctrl Pts',(-0.199307951992349,0.179841290571841,
-1.04242198250146));
#30470=CARTESIAN_POINT('Ctrl Pts',(-0.259345498611925,-0.0693286225162085,
-1.03450152757567));
#30471=CARTESIAN_POINT('Ctrl Pts',(-0.0829842875782713,-0.255304029392523,
-1.02658107264989));
#30472=CARTESIAN_POINT('Ctrl Pts',(0.169018802822267,-0.208564590282341,
-1.0186606177241));
#30473=CARTESIAN_POINT('Ctrl Pts',(0.266957783760862,0.0282857697806424,
-1.01074016279831));
#30474=CARTESIAN_POINT('Ctrl Pts',(0.121559258833056,0.239353063353018,
-1.00281970787253));
#30475=CARTESIAN_POINT('Ctrl Pts',(-0.13464302753518,0.232245125169732,
-0.994899252946743));
#30476=CARTESIAN_POINT('Ctrl Pts',(-0.268115428211658,0.0134409819648169,
-0.986978798020956));
#30477=CARTESIAN_POINT('Ctrl Pts',(-0.157195107209389,-0.217614891559946,
-0.97905834309517));
#30478=CARTESIAN_POINT('Ctrl Pts',(0.0970117836723027,-0.250310320775895,
-0.971137888169384));
#30479=CARTESIAN_POINT('Ctrl Pts',(0.262790440570134,-0.0548427494678456,
-0.963217433243599));
#30480=CARTESIAN_POINT('Ctrl Pts',(0.189030211561587,0.190615114650604,
-0.955296978317811));
#30481=CARTESIAN_POINT('Ctrl Pts',(-0.0570349390971887,0.262323385447104,
-0.947376523392028));
#30482=CARTESIAN_POINT('Ctrl Pts',(-0.251111570932505,0.0949185006637886,
-0.93945606846624));
#30483=CARTESIAN_POINT('Ctrl Pts',(-0.21629484650964,-0.159006547655356,
-0.931535613540455));
#30484=CARTESIAN_POINT('Ctrl Pts',(0.0156790745090038,-0.267993860840813,
-0.923615158614669));
#30485=CARTESIAN_POINT('Ctrl Pts',(0.233361196970594,-0.132699263650284,
-0.915694703688884));
#30486=CARTESIAN_POINT('Ctrl Pts',(0.238329793743047,0.123553438799912,
-0.907774248763097));
#30487=CARTESIAN_POINT('Ctrl Pts',(0.026055886783973,0.267184643250775,
-0.899853793837312));
#30488=CARTESIAN_POINT('Ctrl Pts',(-0.209968496324281,0.167271555789721,
-0.891933338911526));
#30489=CARTESIAN_POINT('Ctrl Pts',(-0.254602281010427,-0.0851129915423963,
-0.884012883985739));
#30490=CARTESIAN_POINT('Ctrl Pts',(-0.0671608554853375,-0.259915298348364,
-0.876092429059954));
#30491=CARTESIAN_POINT('Ctrl Pts',(0.181499069704705,-0.197799470477918,
-0.868171974134168));
#30492=CARTESIAN_POINT('Ctrl Pts',(0.264718863770601,0.0446146387301797,
-0.860251519208382));
#30493=CARTESIAN_POINT('Ctrl Pts',(0.106641974583553,0.246361588081314,
-0.852331064282595));
#30494=CARTESIAN_POINT('Ctrl Pts',(-0.148641265507358,0.223544888139707,
-0.844410609356812));
#30495=CARTESIAN_POINT('Ctrl Pts',(-0.268434938097981,-0.00303757030486697,
-0.836490154431023));
#30496=CARTESIAN_POINT('Ctrl Pts',(-0.143544649335616,-0.226851221006499,
-0.828569699505241));
#30497=CARTESIAN_POINT('Ctrl Pts',(0.112189536571183,-0.243885322865004,
-0.82064924457945));
#30498=CARTESIAN_POINT('Ctrl Pts',(0.265660654841929,-0.0386129420529108,
-0.812728789653669));
#30499=CARTESIAN_POINT('Ctrl Pts',(0.176976627948129,0.201855928783708,
-0.804808334727879));
#30500=CARTESIAN_POINT('Ctrl Pts',(-0.0730252314903912,0.258328973192708,
-0.796887879802097));
#30501=CARTESIAN_POINT('Ctrl Pts',(-0.256463092045629,0.0793298508974973,
-0.788967424876308));
#30502=CARTESIAN_POINT('Ctrl Pts',(-0.206129574898699,-0.171980060405576,
-0.781046969950524));
#30503=CARTESIAN_POINT('Ctrl Pts',(0.0320952849161942,-0.266526613138673,
-0.773126515024738));
#30504=CARTESIAN_POINT('Ctrl Pts',(0.241064633098765,-0.118128681927724,
-0.765206060098951));
#30505=CARTESIAN_POINT('Ctrl Pts',(0.230298615286688,0.137945969937719,
-0.757285605173167));
#30506=CARTESIAN_POINT('Ctrl Pts',(0.00961067791476936,0.26828003596064,
-0.749365150247379));
#30507=CARTESIAN_POINT('Ctrl Pts',(-0.219837589837895,0.154071337111383,
-0.741444695321596));
#30508=CARTESIAN_POINT('Ctrl Pts',(-0.248899377660007,-0.100576551071733,
-0.733524240395808));
#30509=CARTESIAN_POINT('Ctrl Pts',(-0.051084268846874,-0.263546846502485,
-0.725603785470023));
#30510=CARTESIAN_POINT('Ctrl Pts',(0.193295200599941,-0.186288776500498,
-0.717683330544237));
#30511=CARTESIAN_POINT('Ctrl Pts',(0.261482123247759,0.0607753407795304,
-0.709762875618451));
#30512=CARTESIAN_POINT('Ctrl Pts',(0.0913227181314191,0.252441486246047,
-0.701842420692664));
#30513=CARTESIAN_POINT('Ctrl Pts',(-0.162079220882506,0.214002030324816,
-0.69392196576688));
#30514=CARTESIAN_POINT('Ctrl Pts',(-0.267742619974845,-0.0195046731331173,
-0.686001510841093));
#30515=CARTESIAN_POINT('Ctrl Pts',(-0.129353119907832,-0.235232466286298,
-0.678081055915308));
#30516=CARTESIAN_POINT('Ctrl Pts',(0.126944406650368,-0.23654103332236,
-0.670160600989521));
#30517=CARTESIAN_POINT('Ctrl Pts',(0.267529498341093,-0.0222375885020577,
-0.662240146063737));
#30518=CARTESIAN_POINT('Ctrl Pts',(0.164255955620441,0.212335875132393,
-0.654319691137949));
#30519=CARTESIAN_POINT('Ctrl Pts',(-0.0887402654587212,0.253360825920938,
-0.646399236212163));
#30520=CARTESIAN_POINT('Ctrl Pts',(-0.260847911310652,0.0634421783192726,
-0.638478781286379));
#30521=CARTESIAN_POINT('Ctrl Pts',(-0.195187326609645,-0.184305318306346,
-0.630558326360592));
#30522=CARTESIAN_POINT('Ctrl Pts',(0.0483905166239101,-0.264054730550116,
-0.622637871434807));
#30523=CARTESIAN_POINT('Ctrl Pts',(0.247859409720977,-0.103112830616725,
-0.614717416509021));
#30524=CARTESIAN_POINT('Ctrl Pts',(0.221399358326451,0.151818532984811,
-0.606796961583234));
#30525=CARTESIAN_POINT('Ctrl Pts',(-0.00687075706411388,0.268364184500074,
-0.598876506657451));
#30526=CARTESIAN_POINT('Ctrl Pts',(-0.228878036223844,0.140290368020547,
-0.590956051731662));
#30527=CARTESIAN_POINT('Ctrl Pts',(-0.242258282826801,-0.11566100132211,
-0.583035596805878));
#30528=CARTESIAN_POINT('Ctrl Pts',(-0.0348151271832227,-0.266184991583373,
-0.575115141880091));
#30529=CARTESIAN_POINT('Ctrl Pts',(0.204362732201082,-0.174075892967214,
-0.567194686954306));
#30530=CARTESIAN_POINT('Ctrl Pts',(0.25725976233793,0.0767069586599257,
-0.55927423202852));
#30531=CARTESIAN_POINT('Ctrl Pts',(0.0756592334327556,0.257569841443814,
-0.551353777102734));
#30532=CARTESIAN_POINT('Ctrl Pts',(-0.174906241244494,0.203652521709767,
-0.543433322176948));
#30533=CARTESIAN_POINT('Ctrl Pts',(-0.266041083395647,-0.0358982558168854,
-0.535512867251162));
#30534=CARTESIAN_POINT('Ctrl Pts',(-0.114674011939236,-0.242727035599217,
-0.527592412325376));
#30535=CARTESIAN_POINT('Ctrl Pts',(0.141220777497351,-0.228305135351939,
-0.519671957399591));
#30536=CARTESIAN_POINT('Ctrl Pts',(0.268389926716464,-0.0057784134634781,
-0.511751502473804));
#30537=CARTESIAN_POINT('Ctrl Pts',(0.150916143381647,0.222015451020496,
-0.503831047548019));
#30538=CARTESIAN_POINT('Ctrl Pts',(-0.10412080537562,0.24743767035954,-0.495910592622232));
#30539=CARTESIAN_POINT('Ctrl Pts',(-0.264249500762114,0.0473153693000177,
-0.487990137696447));
#30540=CARTESIAN_POINT('Ctrl Pts',(-0.183509346921452,-0.195935863020239,
-0.480069682770661));
#30541=CARTESIAN_POINT('Ctrl Pts',(0.064503347029662,-0.260587530490228,
-0.472149227844876));
#30542=CARTESIAN_POINT('Ctrl Pts',(0.253719914874482,-0.0877083098748911,
-0.464228772919089));
#30543=CARTESIAN_POINT('Ctrl Pts',(0.211665567370078,0.165118837250408,
-0.456308317993303));
#30544=CARTESIAN_POINT('Ctrl Pts',(-0.0233262936827075,0.267436771682676,
-0.448387863067517));
#30545=CARTESIAN_POINT('Ctrl Pts',(-0.237055758780593,0.125980593957881,
-0.440467408141732));
#30546=CARTESIAN_POINT('Ctrl Pts',(-0.234704029191364,-0.130309483562646,
-0.432546953215946));
#30547=CARTESIAN_POINT('Ctrl Pts',(-0.0184147547543408,-0.267819789471133,
-0.42462649829016));
#30548=CARTESIAN_POINT('Ctrl Pts',(0.214659946991667,-0.161206854638871,
-0.416706043364374));
#30549=CARTESIAN_POINT('Ctrl Pts',(0.25206769664155,0.0923494403602257,
-0.408785588438588));
#30550=CARTESIAN_POINT('Ctrl Pts',(0.0597105618080826,0.261727323055098,
-0.400865133512803));
#30551=CARTESIAN_POINT('Ctrl Pts',(-0.187073976929425,0.192535373323535,
-0.392944678587016));
#30552=CARTESIAN_POINT('Ctrl Pts',(-0.263336742065158,-0.0521565250331341,
-0.385024223661231));
#30553=CARTESIAN_POINT('Ctrl Pts',(-0.0995626562795935,-0.249306679211719,
-0.377103768735445));
#30554=CARTESIAN_POINT('Ctrl Pts',(0.15496483632377,-0.219208673022239,
-0.369183313809659));
#30555=CARTESIAN_POINT('Ctrl Pts',(0.26823869670331,0.0107025424985688,
-0.361262858883874));
#30556=CARTESIAN_POINT('Ctrl Pts',(0.137007473793086,0.230858170636998,
-0.353342403958087));
#30557=CARTESIAN_POINT('Ctrl Pts',(-0.119108876441444,0.240581833017126,
-0.345421949032302));
#30558=CARTESIAN_POINT('Ctrl Pts',(-0.266655038583099,0.0310102115966547,
-0.337501494106515));
#30559=CARTESIAN_POINT('Ctrl Pts',(-0.171139654349481,-0.206827854831415,
-0.32958103918073));
#30560=CARTESIAN_POINT('Ctrl Pts',(0.080373041066965,-0.256138082085956,
-0.321660584254943));
#30561=CARTESIAN_POINT('Ctrl Pts',(0.258624058202639,-0.0719731848942422,
-0.313740129329159));
#30562=CARTESIAN_POINT('Ctrl Pts',(0.201133932584729,0.177796749092968,
-0.305819674403371));
#30563=CARTESIAN_POINT('Ctrl Pts',(-0.0396939050912753,0.265501293261684,
-0.297899219477587));
#30564=CARTESIAN_POINT('Ctrl Pts',(-0.244339932723743,0.111195953620514,
-0.2899787645518));
#30565=CARTESIAN_POINT('Ctrl Pts',(-0.226265091458987,-0.144466782383002,
-0.282058309626015));
#30566=CARTESIAN_POINT('Ctrl Pts',(-0.00194497047620613,-0.268445078023149,
-0.274137854700228));
#30567=CARTESIAN_POINT('Ctrl Pts',(0.224148031056896,-0.147730169560283,
-0.266217399774443));
#30568=CARTESIAN_POINT('Ctrl Pts',(0.24592549692617,0.107643823727885,-0.258296944848656));
#30569=CARTESIAN_POINT('Ctrl Pts',(0.0435368195498848,0.264898260032731,
-0.250376489922871));
#30570=CARTESIAN_POINT('Ctrl Pts',(-0.198536563354313,0.180692489706502,
-0.242456034997085));
#30571=CARTESIAN_POINT('Ctrl Pts',(-0.259639789622127,-0.0682181975047813,
-0.234535580071299));
#30572=CARTESIAN_POINT('Ctrl Pts',(-0.0840760130734629,-0.254946596073716,
-0.226615125145513));
#30573=CARTESIAN_POINT('Ctrl Pts',(0.168124776812282,-0.209285934181618,
-0.218694670219728));
#30574=CARTESIAN_POINT('Ctrl Pts',(0.267076378351358,0.0271431567245319,
-0.210774215293941));
#30575=CARTESIAN_POINT('Ctrl Pts',(0.12258237362687,0.238830702574613,-0.202853760368156));
#30576=CARTESIAN_POINT('Ctrl Pts',(-0.133647983179599,0.232819156033741,
-0.19493330544237));
#30577=CARTESIAN_POINT('Ctrl Pts',(-0.268055457498088,0.0145881651932073,
-0.187012850516584));
#30578=CARTESIAN_POINT('Ctrl Pts',(-0.158124874603234,-0.216940237832751,
-0.179092395590798));
#30579=CARTESIAN_POINT('Ctrl Pts',(0.0959397799078894,-0.250723157032861,
-0.171171940665013));
#30580=CARTESIAN_POINT('Ctrl Pts',(0.262553354658447,-0.0559667668044061,
-0.163251485739226));
#30581=CARTESIAN_POINT('Ctrl Pts',(0.189844150667945,0.189804480457345,
-0.155331030813441));
#30582=CARTESIAN_POINT('Ctrl Pts',(-0.055911894283634,0.262565045579588,
-0.147410575887655));
#30583=CARTESIAN_POINT('Ctrl Pts',(-0.250703104374578,0.0959921740771708,
-0.139490120961869));
#30584=CARTESIAN_POINT('Ctrl Pts',(-0.216973273330174,-0.158079530835972,
-0.131569666036083));
#30585=CARTESIAN_POINT('Ctrl Pts',(0.0145321342700516,-0.268058505971775,
-0.123649211110297));
#30586=CARTESIAN_POINT('Ctrl Pts',(0.23279124095941,-0.133696625441738,
-0.115728756184511));
#30587=CARTESIAN_POINT('Ctrl Pts',(0.238856276268229,0.122532438246554,
-0.107808301258725));
#30588=CARTESIAN_POINT('Ctrl Pts',(0.0271990455951673,0.267070738870399,
-0.0998878463329397));
#30589=CARTESIAN_POINT('Ctrl Pts',(-0.209250935021787,0.16816843704613,
-0.0919673914071536));
#30590=CARTESIAN_POINT('Ctrl Pts',(-0.254963893066318,-0.0840225905618564,
-0.0840469364813679));
#30591=CARTESIAN_POINT('Ctrl Pts',(-0.068272966565161,-0.259625794146862,
-0.0761264815555819));
#30592=CARTESIAN_POINT('Ctrl Pts',(0.180651962505275,-0.198573814186845,
-0.0682060266297962));
#30593=CARTESIAN_POINT('Ctrl Pts',(0.264905513374514,0.0434804952224359,
-0.0602855717040101));
#30594=CARTESIAN_POINT('Ctrl Pts',(0.107698711478037,0.245904826017458,
-0.0523651167782246));
#30595=CARTESIAN_POINT('Ctrl Pts',(-0.147689963704326,0.224175421540604,
-0.0444446618524383));
#30596=CARTESIAN_POINT('Ctrl Pts',(-0.268432859279241,-0.00188226022256202,
-0.0365242069266527));
#30597=CARTESIAN_POINT('Ctrl Pts',(-0.144538048210606,-0.226247454230259,
-0.0286037520008667));
#30598=CARTESIAN_POINT('Ctrl Pts',(0.111190498414335,-0.244339288602387,
-0.0206832970750809));
#30599=CARTESIAN_POINT('Ctrl Pts',(0.265405974348622,-0.0397948740947594,
-0.0127628421492951));
#30600=CARTESIAN_POINT('Ctrl Pts',(0.178007129296782,0.201184176175435,
-0.00484238722350905));
#30601=CARTESIAN_POINT('Ctrl Pts',(-0.0722645024832365,0.258464596482291,
0.0030780677022766));
#30602=CARTESIAN_POINT('Ctrl Pts',(-0.194266559193884,0.140045363462362,
0.00835837098613384));
#30603=CARTESIAN_POINT('Ctrl Pts',(-0.216859401302392,0.0680976509636584,
0.0109985226280624));
#30604=CARTESIAN_POINT('Ctrl Pts',(0.126471106027295,-0.177287929553122,
-1.16365));
#30605=CARTESIAN_POINT('Ctrl Pts',(0.185290142270931,-0.135328453868889,
-1.16100984835807));
#30606=CARTESIAN_POINT('Ctrl Pts',(0.25689562471139,0.0109872606886212,
-1.15572954507421));
#30607=CARTESIAN_POINT('Ctrl Pts',(0.130348081000917,0.221923062878552,
-1.14780909014843));
#30608=CARTESIAN_POINT('Ctrl Pts',(-0.115118491958846,0.229917045457789,
-1.13988863522264));
#30609=CARTESIAN_POINT('Ctrl Pts',(-0.255597470383498,0.0286658565984495,
-1.13196818029686));
#30610=CARTESIAN_POINT('Ctrl Pts',(-0.163122903762403,-0.198886145851415,
-1.12404772537107));
#30611=CARTESIAN_POINT('Ctrl Pts',(0.0780566987792774,-0.245059402025012,
-1.11612727044528));
#30612=CARTESIAN_POINT('Ctrl Pts',(0.248078039310978,-0.0679032867325597,
-1.1082068155195));
#30613=CARTESIAN_POINT('Ctrl Pts',(0.191975348375761,0.171172964635631,
-1.10028636059371));
#30614=CARTESIAN_POINT('Ctrl Pts',(-0.0391190265108933,0.254208440109437,
-1.09236590566793));
#30615=CARTESIAN_POINT('Ctrl Pts',(-0.234554442114105,0.10553459470797,
-1.08444545074214));
#30616=CARTESIAN_POINT('Ctrl Pts',(-0.216189276575422,-0.139339830996314,
-1.07652499581635));
#30617=CARTESIAN_POINT('Ctrl Pts',(-0.000762821507371324,-0.25720122800503,
-1.06860454089057));
#30618=CARTESIAN_POINT('Ctrl Pts',(0.215358791521507,-0.140619426360152,
-1.06068408596478));
#30619=CARTESIAN_POINT('Ctrl Pts',(0.235176530521566,0.104140400581766,
-1.052763631039));
#30620=CARTESIAN_POINT('Ctrl Pts',(0.0406259830504325,0.253973834313976,
-1.04484317611321));
#30621=CARTESIAN_POINT('Ctrl Pts',(-0.190955957963633,0.172305046433272,
-1.03692272118743));
#30622=CARTESIAN_POINT('Ctrl Pts',(-0.248477632908984,-0.0664234085722272,
-1.02900226626164));
#30623=CARTESIAN_POINT('Ctrl Pts',(-0.0795068333803697,-0.244605521341649,
-1.02108181133586));
#30624=CARTESIAN_POINT('Ctrl Pts',(0.161936074723358,-0.199824697090791,
-1.01316135641007));
#30625=CARTESIAN_POINT('Ctrl Pts',(0.25577092546644,0.0271004554068604,
-1.00524090148428));
#30626=CARTESIAN_POINT('Ctrl Pts',(0.116465321567834,0.229322980077886,
-0.997320446558497));
#30627=CARTESIAN_POINT('Ctrl Pts',(-0.129000815316647,0.222512899840908,
-0.98939999163271));
#30628=CARTESIAN_POINT('Ctrl Pts',(-0.25688005885963,0.0128777379999474,
-0.981479536706925));
#30629=CARTESIAN_POINT('Ctrl Pts',(-0.15060785073702,-0.208495745752166,
-0.973559081781138));
#30630=CARTESIAN_POINT('Ctrl Pts',(0.092946507651719,-0.239821073941797,
-0.965638626855354));
#30631=CARTESIAN_POINT('Ctrl Pts',(0.251778214672948,-0.05254456561971,
-0.957718171929568));
#30632=CARTESIAN_POINT('Ctrl Pts',(0.181108905951714,0.182627393722108,
-0.949797717003781));
#30633=CARTESIAN_POINT('Ctrl Pts',(-0.0546448916053246,0.251330731481492,
-0.941877262077996));
#30634=CARTESIAN_POINT('Ctrl Pts',(-0.240588747733507,0.090940943607816,
-0.93395680715221));
#30635=CARTESIAN_POINT('Ctrl Pts',(-0.207231017151944,-0.1523433828229,
-0.926036352226423));
#30636=CARTESIAN_POINT('Ctrl Pts',(0.0150220433400717,-0.256763585765983,
-0.918115897300639));
#30637=CARTESIAN_POINT('Ctrl Pts',(0.22358220268487,-0.127138504801763,
-0.910195442374852));
#30638=CARTESIAN_POINT('Ctrl Pts',(0.228342590551659,0.118375935480206,
-0.902274987449066));
#30639=CARTESIAN_POINT('Ctrl Pts',(0.0249640155933997,0.255988278415915,
-0.894354532523281));
#30640=CARTESIAN_POINT('Ctrl Pts',(-0.201169772490191,0.160262046027745,
-0.886434077597493));
#30641=CARTESIAN_POINT('Ctrl Pts',(-0.243933179705436,-0.0815463340657517,
-0.87851362267171));
#30642=CARTESIAN_POINT('Ctrl Pts',(-0.0643464817567947,-0.249023555203761,
-0.870593167745921));
#30643=CARTESIAN_POINT('Ctrl Pts',(0.173893356378981,-0.189510689323927,
-0.862672712820138));
#30644=CARTESIAN_POINT('Ctrl Pts',(0.253625827354345,0.042745063570017,
-0.85475225789435));
#30645=CARTESIAN_POINT('Ctrl Pts',(0.102173145688224,0.236037812777863,
-0.846831802968565));
#30646=CARTESIAN_POINT('Ctrl Pts',(-0.142412457526902,0.214177245994829,
-0.838911348042779));
#30647=CARTESIAN_POINT('Ctrl Pts',(-0.257186179693303,-0.00291028100810552,
-0.830990893116994));
#30648=CARTESIAN_POINT('Ctrl Pts',(-0.137529414910091,-0.217345027077388,
-0.823070438191206));
#30649=CARTESIAN_POINT('Ctrl Pts',(0.107488237249403,-0.233665315384629,
-0.815149983265423));
#30650=CARTESIAN_POINT('Ctrl Pts',(0.254528152697761,-0.0369948678203813,
-0.807229528339635));
#30651=CARTESIAN_POINT('Ctrl Pts',(0.169560427414887,0.193397161860414,
-0.79930907341385));
#30652=CARTESIAN_POINT('Ctrl Pts',(-0.0699651112530573,0.247503704958389,
-0.791388618488063));
#30653=CARTESIAN_POINT('Ctrl Pts',(-0.245716013507421,0.0760055357641992,
-0.783468163562279));
#30654=CARTESIAN_POINT('Ctrl Pts',(-0.197491720957168,-0.164773240892319,
-0.775547708636491));
#30655=CARTESIAN_POINT('Ctrl Pts',(0.0307503329195962,-0.255357823036844,
-0.767627253710707));
#30656=CARTESIAN_POINT('Ctrl Pts',(0.230962826542383,-0.113178502889618,
-0.759706798784921));
#30657=CARTESIAN_POINT('Ctrl Pts',(0.220647958398849,0.132165348012261,
-0.751786343859134));
#30658=CARTESIAN_POINT('Ctrl Pts',(0.00920794273158324,0.257037768725599,
-0.743865888933349));
#30659=CARTESIAN_POINT('Ctrl Pts',(-0.210625301922338,0.147614982135642,
-0.735945434007564));
#30660=CARTESIAN_POINT('Ctrl Pts',(-0.238469256356832,-0.096361893575216,
-0.728024979081776));
#30661=CARTESIAN_POINT('Ctrl Pts',(-0.0489435840216807,-0.252502923436333,
-0.720104524155992));
#30662=CARTESIAN_POINT('Ctrl Pts',(0.18519517074638,-0.178482350648465,
-0.712184069230205));
#30663=CARTESIAN_POINT('Ctrl Pts',(0.250524722350552,0.0582285518621306,
-0.70426361430442));
#30664=CARTESIAN_POINT('Ctrl Pts',(0.0874958422396386,0.241862932983866,
-0.696343159378634));
#30665=CARTESIAN_POINT('Ctrl Pts',(-0.155287295766334,0.205034281363778,
-0.688422704452848));
#30666=CARTESIAN_POINT('Ctrl Pts',(-0.256522873141319,-0.0186873303632409,
-0.680502249527062));
#30667=CARTESIAN_POINT('Ctrl Pts',(-0.12393258111715,-0.225375056513412,
-0.672581794601276));
#30668=CARTESIAN_POINT('Ctrl Pts',(0.121624804919859,-0.226628788085249,
-0.664661339675491));
#30669=CARTESIAN_POINT('Ctrl Pts',(0.256318682363535,-0.0213057229917977,
-0.656740884749704));
#30670=CARTESIAN_POINT('Ctrl Pts',(0.157372814497323,0.203437946357048,
-0.648820429823919));
#30671=CARTESIAN_POINT('Ctrl Pts',(-0.0850216071723404,0.242743747755972,
-0.640899974898132));
#30672=CARTESIAN_POINT('Ctrl Pts',(-0.249917087046534,0.0607836356510322,
-0.632979519972347));
#30673=CARTESIAN_POINT('Ctrl Pts',(-0.187008007269756,-0.176582009213218,
-0.625059065046561));
#30674=CARTESIAN_POINT('Ctrl Pts',(0.046362713408588,-0.252989524617473,
-0.617138610120775));
#30675=CARTESIAN_POINT('Ctrl Pts',(0.237472868244547,-0.0987918903984044,
-0.609218155194989));
#30676=CARTESIAN_POINT('Ctrl Pts',(0.212121624547043,0.145456581701572,
-0.601297700269203));
#30677=CARTESIAN_POINT('Ctrl Pts',(-0.00658283818582227,0.257118391022893,
-0.593377245343417));
#30678=CARTESIAN_POINT('Ctrl Pts',(-0.21928690866101,0.134411504160469,
-0.585456790417632));
#30679=CARTESIAN_POINT('Ctrl Pts',(-0.2321064564127,-0.110814230369215,
-0.577536335491846));
#30680=CARTESIAN_POINT('Ctrl Pts',(-0.033356200274203,-0.255030517123049,
-0.569615880566061));
#30681=CARTESIAN_POINT('Ctrl Pts',(0.195798917752269,-0.166781247650396,
-0.561695425640274));
#30682=CARTESIAN_POINT('Ctrl Pts',(0.246479299353905,0.0734925557508373,
-0.553774970714489));
#30683=CARTESIAN_POINT('Ctrl Pts',(0.0724887354193506,0.246776384603724,
-0.545854515788701));
#30684=CARTESIAN_POINT('Ctrl Pts',(-0.167576800206862,0.195118468611283,
-0.537934060862918));
#30685=CARTESIAN_POINT('Ctrl Pts',(-0.254892639403815,-0.0343939404334457,
-0.53001360593713));
#30686=CARTESIAN_POINT('Ctrl Pts',(-0.109868600748205,-0.232555566113592,
-0.522093151011346));
#30687=CARTESIAN_POINT('Ctrl Pts',(0.135302924854754,-0.21873801518376,
-0.514172696085558));
#30688=CARTESIAN_POINT('Ctrl Pts',(0.257143054512441,-0.0055362692125341,
-0.506252241159774));
#30689=CARTESIAN_POINT('Ctrl Pts',(0.144592006708923,0.212711899894362,
-0.498331786233987));
#30690=CARTESIAN_POINT('Ctrl Pts',(-0.0997576260038526,0.237068801858992,
-0.490411331308202));
#30691=CARTESIAN_POINT('Ctrl Pts',(-0.253176132989307,0.0453326201025579,
-0.482490876382416));
#30692=CARTESIAN_POINT('Ctrl Pts',(-0.175819392986446,-0.187725176283469,
-0.474570421456629));
#30693=CARTESIAN_POINT('Ctrl Pts',(0.0618003361169582,-0.249667617476944,
-0.466649966530844));
#30694=CARTESIAN_POINT('Ctrl Pts',(0.243087789097186,-0.0840328956577408,
-0.458729511605058));
#30695=CARTESIAN_POINT('Ctrl Pts',(0.202795727822344,0.158199537097262,
-0.450809056679272));
#30696=CARTESIAN_POINT('Ctrl Pts',(-0.0223488060129853,0.256229841413087,
-0.442888601753486));
#30697=CARTESIAN_POINT('Ctrl Pts',(-0.227121943987874,0.120701380770689,
-0.4349681468277));
#30698=CARTESIAN_POINT('Ctrl Pts',(-0.22486876355983,-0.124848868380357,
-0.427047691901915));
#30699=CARTESIAN_POINT('Ctrl Pts',(-0.0176430849829593,-0.256596808852072,
-0.419127236976129));
#30700=CARTESIAN_POINT('Ctrl Pts',(0.205664628051519,-0.154451486005192,
-0.411206782050343));
#30701=CARTESIAN_POINT('Ctrl Pts',(0.241504807022057,0.0884795397028073,
-0.403286327124557));
#30702=CARTESIAN_POINT('Ctrl Pts',(0.0572083924230321,0.250759647066977,
-0.395365872198771));
#30703=CARTESIAN_POINT('Ctrl Pts',(-0.179234647275871,0.184467184010264,
-0.387445417272985));
#30704=CARTESIAN_POINT('Ctrl Pts',(-0.252301623419445,-0.0499709073431182,
-0.379524962347199));
#30705=CARTESIAN_POINT('Ctrl Pts',(-0.0953904860153474,-0.238859489948667,
-0.371604507421413));
#30706=CARTESIAN_POINT('Ctrl Pts',(0.148471039289085,-0.210022739847858,
-0.363684052495628));
#30707=CARTESIAN_POINT('Ctrl Pts',(0.256998161788665,0.0102540527612222,
-0.355763597569842));
#30708=CARTESIAN_POINT('Ctrl Pts',(0.13126617952173,0.221184065598206,-0.347843142644056));
#30709=CARTESIAN_POINT('Ctrl Pts',(-0.11411762238027,0.230500258184359,
-0.33992268771827));
#30710=CARTESIAN_POINT('Ctrl Pts',(-0.255480866816693,0.0297107295664827,
-0.332002232792484));
#30711=CARTESIAN_POINT('Ctrl Pts',(-0.163968052027973,-0.198160739489272,
-0.324081777866699));
#30712=CARTESIAN_POINT('Ctrl Pts',(0.0770050110794473,-0.245404623080814,
-0.316161322940912));
#30713=CARTESIAN_POINT('Ctrl Pts',(0.247786424439417,-0.0689571506394352,
-0.308240868015127));
#30714=CARTESIAN_POINT('Ctrl Pts',(0.192705420891506,0.170346181406604,
-0.300320413089341));
#30715=CARTESIAN_POINT('Ctrl Pts',(-0.038030533133535,0.254375469159979,
-0.292399958163555));
#30716=CARTESIAN_POINT('Ctrl Pts',(-0.234100874830238,0.106536290363869,
-0.284479503237769));
#30717=CARTESIAN_POINT('Ctrl Pts',(-0.216783459271804,-0.138412905998497,
-0.276559048311983));
#30718=CARTESIAN_POINT('Ctrl Pts',(-0.00186346654402013,-0.257195894705197,
-0.268638593386197));
#30719=CARTESIAN_POINT('Ctrl Pts',(0.214755114225321,-0.141539541029435,
-0.260718138460412));
#30720=CARTESIAN_POINT('Ctrl Pts',(0.235619996010104,0.103133012372812,
-0.252797683534625));
#30721=CARTESIAN_POINT('Ctrl Pts',(0.0417124103716506,0.25379770602124,
-0.24487722860884));
#30722=CARTESIAN_POINT('Ctrl Pts',(-0.190216894344415,0.173120576092536,
-0.236956773683054));
#30723=CARTESIAN_POINT('Ctrl Pts',(-0.248759591662818,-0.0653595158891499,
-0.229036318757268));
#30724=CARTESIAN_POINT('Ctrl Pts',(-0.0805528101499051,-0.244263066255845,
-0.221115863831482));
#30725=CARTESIAN_POINT('Ctrl Pts',(0.161079512847755,-0.200515813094597,
-0.213195408905696));
#30726=CARTESIAN_POINT('Ctrl Pts',(0.255884550354012,0.0260057235181914,
-0.20527495397991));
#30727=CARTESIAN_POINT('Ctrl Pts',(0.117445562765472,0.228822508812962,
-0.197354499054125));
#30728=CARTESIAN_POINT('Ctrl Pts',(-0.128047468266331,0.223062875957976,
-0.189434044128339));
#30729=CARTESIAN_POINT('Ctrl Pts',(-0.256822601217097,0.0139768485479575,
-0.181513589202553));
#30730=CARTESIAN_POINT('Ctrl Pts',(-0.151498656254814,-0.207849363370115,
-0.173593134276767));
#30731=CARTESIAN_POINT('Ctrl Pts',(0.0919194261743976,-0.240216610307221,
-0.165672679350981));
#30732=CARTESIAN_POINT('Ctrl Pts',(0.25155106383961,-0.0536214810419249,
-0.157752224425195));
#30733=CARTESIAN_POINT('Ctrl Pts',(0.181888736963096,0.181850729131537,
-0.149831769499409));
#30734=CARTESIAN_POINT('Ctrl Pts',(-0.0535689079525661,0.251562264853035,
-0.141911314573623));
#30735=CARTESIAN_POINT('Ctrl Pts',(-0.240197397955011,0.0919696247675137,
-0.133990859647838));
#30736=CARTESIAN_POINT('Ctrl Pts',(-0.207881014515963,-0.151455212616823,
-0.126070404722052));
#30737=CARTESIAN_POINT('Ctrl Pts',(0.0139231655990339,-0.256825521944582,
-0.118149949796266));
#30738=CARTESIAN_POINT('Ctrl Pts',(0.223036130664036,-0.128094072175867,
-0.11022949487048));
#30739=CARTESIAN_POINT('Ctrl Pts',(0.228847010841678,0.117397719925839,
-0.102309039944694));
#30740=CARTESIAN_POINT('Ctrl Pts',(0.0260592703673014,0.255879147195341,
-0.0943885850189083));
#30741=CARTESIAN_POINT('Ctrl Pts',(-0.200482280573558,0.161121343500753,
-0.0864681300931226));
#30742=CARTESIAN_POINT('Ctrl Pts',(-0.244279638418466,-0.0805016263071196,
-0.0785476751673364));
#30743=CARTESIAN_POINT('Ctrl Pts',(-0.0654119898536204,-0.248746182667544,
-0.0706272202415509));
#30744=CARTESIAN_POINT('Ctrl Pts',(0.173081747182517,-0.190252584181875,
-0.0627067653157647));
#30745=CARTESIAN_POINT('Ctrl Pts',(0.253804655411944,0.0416584463135328,
-0.0547863103899791));
#30746=CARTESIAN_POINT('Ctrl Pts',(0.103185600053364,0.235600191315231,
-0.0468658554641932));
#30747=CARTESIAN_POINT('Ctrl Pts',(-0.141501019998722,0.214781356911593,
-0.0389454005384072));
#30748=CARTESIAN_POINT('Ctrl Pts',(-0.257184187987403,-0.00180338416176167,
-0.0310249456126215));
#30749=CARTESIAN_POINT('Ctrl Pts',(-0.138481185433633,-0.216766561130641,
-0.0231044906868355));
#30750=CARTESIAN_POINT('Ctrl Pts',(0.106531063757949,-0.234100257700769,
-0.0151840357610497));
#30751=CARTESIAN_POINT('Ctrl Pts',(0.254284144583244,-0.0381272710338155,
-0.00726358083526386));
#30752=CARTESIAN_POINT('Ctrl Pts',(0.170547745633993,0.19275355902598,0.000656874090522184));
#30753=CARTESIAN_POINT('Ctrl Pts',(-0.0692362605731931,0.247633644957901,
0.00857732901630782));
#30754=CARTESIAN_POINT('Ctrl Pts',(-0.186125824586221,0.134176766511289,
0.0138576323001651));
#30755=CARTESIAN_POINT('Ctrl Pts',(-0.20777191429225,0.0652440208473855,
0.0164977839420937));
#30756=CARTESIAN_POINT('Ctrl Pts',(0.157411390703589,0.150985252349406,
2.77555756156289E-17));
#30757=CARTESIAN_POINT('Ctrl Pts',(0.153564701611678,0.155598258518773,
1.79071970638144E-17));
#30758=CARTESIAN_POINT('Ctrl Pts',(0.149524200953796,0.160033000704482,
-1.97347420389862E-16));
#30759=CARTESIAN_POINT('Ctrl Pts',(0.145294941952413,0.164273870340422,
-1.45716771982052E-16));
#30760=CARTESIAN_POINT('Ctrl Pts',(0.13714601219612,0.172445171449571,-4.59119247969748E-17));
#30761=CARTESIAN_POINT('Ctrl Pts',(0.128297493209746,0.179897878181489,
-8.12010810131507E-18));
#30762=CARTESIAN_POINT('Ctrl Pts',(0.118867987330782,0.186618959304511,
-4.5102810375397E-17));
#30763=CARTESIAN_POINT('Ctrl Pts',(0.114918429711642,0.189434090606089,
-6.05930508416384E-17));
#30764=CARTESIAN_POINT('Ctrl Pts',(0.110867035362717,0.192120070666577,
6.04783058210693E-17));
#30765=CARTESIAN_POINT('Ctrl Pts',(0.106733791498232,0.194668718081002,
6.93889390390723E-18));
#30766=CARTESIAN_POINT('Ctrl Pts',(0.0951061479421179,0.201838574169047,
-1.4367820452717E-16));
#30767=CARTESIAN_POINT('Ctrl Pts',(0.0828107346625941,0.20794034750507,
1.36988496431349E-16));
#30768=CARTESIAN_POINT('Ctrl Pts',(0.0700321885925319,0.212945356424772,
2.89698820488127E-16));
#30769=CARTESIAN_POINT('Ctrl Pts',(0.0649061281753037,0.214953094861562,
3.50957929557155E-16));
#30770=CARTESIAN_POINT('Ctrl Pts',(0.0596992770508872,0.216784433784475,
1.31329437058139E-16));
#30771=CARTESIAN_POINT('Ctrl Pts',(0.0544460276382488,0.218429702201119,
1.26634813746307E-16));
#30772=CARTESIAN_POINT('Ctrl Pts',(0.0403476443297082,0.222845183546339,
1.14035640598315E-16));
#30773=CARTESIAN_POINT('Ctrl Pts',(0.0258845556478006,0.225938110725585,
4.51833798814228E-17));
#30774=CARTESIAN_POINT('Ctrl Pts',(0.011276871154686,0.227669918440373,
-8.32667268468867E-17));
#30775=CARTESIAN_POINT('Ctrl Pts',(0.00107476123702629,0.228879425167524,
-1.7297718769337E-16));
#30776=CARTESIAN_POINT('Ctrl Pts',(-0.00919870048170219,0.229424155614405,
-2.66449797732721E-16));
#30777=CARTESIAN_POINT('Ctrl Pts',(-0.0194725016422591,0.229276419562986,
-2.68882138776405E-16));
#30778=CARTESIAN_POINT('Ctrl Pts',(-0.0236251828733368,0.229216704495672,
-2.69865293583651E-16));
#30779=CARTESIAN_POINT('Ctrl Pts',(-0.0277781740641179,0.229043424833214,
-8.41623659136518E-17));
#30780=CARTESIAN_POINT('Ctrl Pts',(-0.031911729017349,0.22875596618419,
-8.84708972748172E-17));
#30781=CARTESIAN_POINT('Ctrl Pts',(-0.0422252418762031,0.228038736461434,
-9.92209886849774E-17));
#30782=CARTESIAN_POINT('Ctrl Pts',(-0.0524404675808494,0.226611656750976,
-3.83662481248865E-16));
#30783=CARTESIAN_POINT('Ctrl Pts',(-0.0624850909091108,0.224457085590244,
-3.83373888190874E-16));
#30784=CARTESIAN_POINT('Ctrl Pts',(-0.0721327246316351,0.222387668678475,
-3.83096701080181E-16));
#30785=CARTESIAN_POINT('Ctrl Pts',(-0.0816232357754141,0.219647153966434,
-9.52791738662464E-17));
#30786=CARTESIAN_POINT('Ctrl Pts',(-0.0909164539954311,0.216284339764173,
-1.27502175484295E-16));
#30787=CARTESIAN_POINT('Ctrl Pts',(-0.0960519283334126,0.214426033456255,
-1.45308751633104E-16));
#30788=CARTESIAN_POINT('Ctrl Pts',(-0.101127127636006,0.212377488573957,
2.08088708794294E-16));
#30789=CARTESIAN_POINT('Ctrl Pts',(-0.10613488128436,0.210145550644494,
2.45463371850718E-16));
#30790=CARTESIAN_POINT('Ctrl Pts',(-0.110154437304024,0.208354048871471,
2.754627612817E-16));
#30791=CARTESIAN_POINT('Ctrl Pts',(-0.11413142148668,0.206443620358008,
1.33107852961981E-16));
#30792=CARTESIAN_POINT('Ctrl Pts',(-0.118046763621651,0.204426094738635,
1.17093834628434E-16));
#30793=CARTESIAN_POINT('Ctrl Pts',(-0.131295948505429,0.197598959582277,
6.29037581755335E-17));
#30794=CARTESIAN_POINT('Ctrl Pts',(-0.143882118085797,0.189531964554253,
-2.12688715064594E-18));
#30795=CARTESIAN_POINT('Ctrl Pts',(-0.155672563194254,0.180388335621176,
-2.18575157973078E-16));
#30796=CARTESIAN_POINT('Ctrl Pts',(-0.161475748336318,0.175887897250879,
-3.25109676195897E-16));
#30797=CARTESIAN_POINT('Ctrl Pts',(-0.167085969791737,0.171125853649587,
-2.08309637886367E-16));
#30798=CARTESIAN_POINT('Ctrl Pts',(-0.172485522512255,0.166117669875527,
-1.88651178012478E-16));
#30799=CARTESIAN_POINT('Ctrl Pts',(-0.176399951057423,0.162486965900707,
-1.74399694516081E-16));
#30800=CARTESIAN_POINT('Ctrl Pts',(-0.18020363364379,0.158726847330799,
-2.2547246652764E-17));
#30801=CARTESIAN_POINT('Ctrl Pts',(-0.183889191084364,0.154842509473871,
-1.99493199737333E-17));
#30802=CARTESIAN_POINT('Ctrl Pts',(-0.187043738235936,0.151517821927989,
-1.77256991680701E-17));
#30803=CARTESIAN_POINT('Ctrl Pts',(-0.19010667756743,0.148107231803098,
-2.31285918917368E-16));
#30804=CARTESIAN_POINT('Ctrl Pts',(-0.193068825214573,0.1446211636127,-2.34621350125863E-16));
#30805=CARTESIAN_POINT('Ctrl Pts',(-0.203021696728538,0.132907909271241,
-2.45828461389825E-16));
#30806=CARTESIAN_POINT('Ctrl Pts',(-0.211858816472026,0.120324866147189,
-1.29773094504587E-16));
#30807=CARTESIAN_POINT('Ctrl Pts',(-0.219427486736791,0.107016492388279,
-1.84314369322536E-16));
#30808=CARTESIAN_POINT('Ctrl Pts',(-0.225471071905783,0.0963897524908907,
-2.27865591407372E-16));
#30809=CARTESIAN_POINT('Ctrl Pts',(-0.230705723677907,0.0852994432307312,
-6.22160315497662E-18));
#30810=CARTESIAN_POINT('Ctrl Pts',(-0.235034375322676,0.0738049111962042,
0.));
#30811=CARTESIAN_POINT('Origin',(0.429366365092022,-0.191166222245626,0.6));
#30812=CARTESIAN_POINT('',(0.429366365092022,-0.191166222245626,0.57));
#30813=CARTESIAN_POINT('',(0.4625355188348,-0.189897061104753,0.54));
#30814=CARTESIAN_POINT('Ctrl Pts',(0.429366365092022,-0.191166222245626,
0.57));
#30815=CARTESIAN_POINT('Ctrl Pts',(0.445438016905544,-0.190551267878399,
0.555567939963915));
#30816=CARTESIAN_POINT('Ctrl Pts',(0.4625355188348,-0.189897061104753,0.54));
#30817=CARTESIAN_POINT('',(0.429366365092022,-0.191166222245626,0.0200000000000001));
#30818=CARTESIAN_POINT('',(0.429366365092022,-0.191166222245626,0.6));
#30819=CARTESIAN_POINT('',(0.4625355188348,-0.189897061104753,0.05));
#30820=CARTESIAN_POINT('Ctrl Pts',(0.4625355188348,-0.189897061104753,0.05));
#30821=CARTESIAN_POINT('Ctrl Pts',(0.445438016905538,-0.190551267878399,
0.03443206003608));
#30822=CARTESIAN_POINT('Ctrl Pts',(0.429366365092022,-0.191166222245626,
0.0200000000000001));
#30823=CARTESIAN_POINT('',(0.4625355188348,-0.189897061104753,0.295));
#30824=CARTESIAN_POINT('Origin',(0.478549932784856,-0.250179858964726,0.6));
#30825=CARTESIAN_POINT('',(0.450617690513801,-0.216664941778795,0.54));
#30826=CARTESIAN_POINT('Ctrl Pts',(0.450617690513801,-0.216664941778795,
0.54));
#30827=CARTESIAN_POINT('Ctrl Pts',(0.439663399059283,-0.203521271916345,
0.555567939963915));
#30828=CARTESIAN_POINT('Ctrl Pts',(0.429366365092022,-0.191166222245626,
0.57));
#30829=CARTESIAN_POINT('',(0.450617690513801,-0.216664941778795,0.05));
#30830=CARTESIAN_POINT('',(0.450617690513801,-0.216664941778795,0.295));
#30831=CARTESIAN_POINT('Ctrl Pts',(0.429366365092022,-0.191166222245626,
0.0200000000000001));
#30832=CARTESIAN_POINT('Ctrl Pts',(0.439663399059267,-0.203521271916326,
0.0344320600360628));
#30833=CARTESIAN_POINT('Ctrl Pts',(0.450617690513801,-0.216664941778795,
0.0500000000000001));
#30834=CARTESIAN_POINT('Origin',(0.314491384988663,-0.349278067974375,0.6));
#30835=CARTESIAN_POINT('',(0.314491384988663,-0.349278067974375,0.57));
#30836=CARTESIAN_POINT('',(0.345309129066188,-0.361609741826117,0.54));
#30837=CARTESIAN_POINT('Ctrl Pts',(0.314491384988663,-0.349278067974375,
0.57));
#30838=CARTESIAN_POINT('Ctrl Pts',(0.329423693974679,-0.355253208912848,
0.555567939963926));
#30839=CARTESIAN_POINT('Ctrl Pts',(0.345309129066188,-0.361609741826117,
0.54));
#30840=CARTESIAN_POINT('',(0.314491384988663,-0.349278067974375,0.0200000000000001));
#30841=CARTESIAN_POINT('',(0.314491384988663,-0.349278067974375,0.6));
#30842=CARTESIAN_POINT('',(0.345309129066188,-0.361609741826117,0.05));
#30843=CARTESIAN_POINT('Ctrl Pts',(0.345309129066188,-0.361609741826117,
0.0500000000000001));
#30844=CARTESIAN_POINT('Ctrl Pts',(0.32942369397468,-0.355253208912848,
0.0344320600360752));
#30845=CARTESIAN_POINT('Ctrl Pts',(0.314491384988663,-0.349278067974375,
0.0200000000000001));
#30846=CARTESIAN_POINT('',(0.345309129066188,-0.361609741826117,0.295));
#30847=CARTESIAN_POINT('Origin',(0.335419801350288,-0.423194466955954,0.6));
#30848=CARTESIAN_POINT('',(0.323534173210961,-0.38121600014257,0.54));
#30849=CARTESIAN_POINT('Ctrl Pts',(0.323534173210961,-0.38121600014257,
0.54));
#30850=CARTESIAN_POINT('Ctrl Pts',(0.31887294216854,-0.364753148509481,
0.555567939963924));
#30851=CARTESIAN_POINT('Ctrl Pts',(0.314491384988663,-0.349278067974375,
0.57));
#30852=CARTESIAN_POINT('',(0.323534173210961,-0.38121600014257,0.05));
#30853=CARTESIAN_POINT('',(0.323534173210961,-0.38121600014257,0.295));
#30854=CARTESIAN_POINT('Ctrl Pts',(0.314491384988663,-0.349278067974375,
0.0200000000000001));
#30855=CARTESIAN_POINT('Ctrl Pts',(0.318872942168538,-0.364753148509474,
0.0344320600360705));
#30856=CARTESIAN_POINT('Ctrl Pts',(0.323534173210961,-0.38121600014257,
0.0500000000000001));
#30857=CARTESIAN_POINT('Origin',(0.145237987356225,-0.446996562658722,0.6));
#30858=CARTESIAN_POINT('',(0.145237987356225,-0.446996562658722,0.57));
#30859=CARTESIAN_POINT('',(0.168375653847077,-0.470796813064372,0.54));
#30860=CARTESIAN_POINT('Ctrl Pts',(0.145237987356225,-0.446996562658722,
0.57));
#30861=CARTESIAN_POINT('Ctrl Pts',(0.156449021635303,-0.458528642752187,
0.555567939963917));
#30862=CARTESIAN_POINT('Ctrl Pts',(0.168375653847077,-0.470796813064372,
0.54));
#30863=CARTESIAN_POINT('',(0.145237987356225,-0.446996562658722,0.0200000000000001));
#30864=CARTESIAN_POINT('',(0.145237987356225,-0.446996562658722,0.6));
#30865=CARTESIAN_POINT('',(0.168375653847077,-0.470796813064372,0.05));
#30866=CARTESIAN_POINT('Ctrl Pts',(0.168375653847077,-0.470796813064372,
0.05));
#30867=CARTESIAN_POINT('Ctrl Pts',(0.156449021635302,-0.458528642752186,
0.0344320600360816));
#30868=CARTESIAN_POINT('Ctrl Pts',(0.145237987356225,-0.446996562658722,
0.0200000000000001));
#30869=CARTESIAN_POINT('',(0.168375653847077,-0.470796813064372,0.295));
#30870=CARTESIAN_POINT('Origin',(0.134292539069021,-0.523034907009461,0.6));
#30871=CARTESIAN_POINT('',(0.140508658144255,-0.479851348843057,0.54));
#30872=CARTESIAN_POINT('Ctrl Pts',(0.140508658144255,-0.479851348843057,
0.54));
#30873=CARTESIAN_POINT('Ctrl Pts',(0.142946456707127,-0.462915892047004,
0.555567939963928));
#30874=CARTESIAN_POINT('Ctrl Pts',(0.145237987356225,-0.446996562658722,
0.57));
#30875=CARTESIAN_POINT('',(0.140508658144255,-0.479851348843057,0.05));
#30876=CARTESIAN_POINT('',(0.140508658144255,-0.479851348843057,0.295));
#30877=CARTESIAN_POINT('Ctrl Pts',(0.145237987356225,-0.446996562658722,
0.0200000000000001));
#30878=CARTESIAN_POINT('Ctrl Pts',(0.142946456707125,-0.46291589204702,
0.034432060036086));
#30879=CARTESIAN_POINT('Ctrl Pts',(0.140508658144255,-0.479851348843057,
0.05));
#30880=CARTESIAN_POINT('Origin',(-0.0491283777357971,-0.467425290823089,
0.6));
#30881=CARTESIAN_POINT('',(-0.0491283777357971,-0.467425290823089,0.57));
#30882=CARTESIAN_POINT('',(-0.0376715015669875,-0.498578838269023,0.54));
#30883=CARTESIAN_POINT('Ctrl Pts',(-0.0491283777357971,-0.467425290823089,
0.57));
#30884=CARTESIAN_POINT('Ctrl Pts',(-0.0435771078395689,-0.482520308657719,
0.555567939963922));
#30885=CARTESIAN_POINT('Ctrl Pts',(-0.0376715015669874,-0.498578838269023,
0.54));
#30886=CARTESIAN_POINT('',(-0.0491283777357971,-0.467425290823089,0.0200000000000001));
#30887=CARTESIAN_POINT('',(-0.0491283777357971,-0.467425290823089,0.6));
#30888=CARTESIAN_POINT('',(-0.0376715015669875,-0.498578838269023,0.05));
#30889=CARTESIAN_POINT('Ctrl Pts',(-0.0376715015669875,-0.498578838269023,
0.05));
#30890=CARTESIAN_POINT('Ctrl Pts',(-0.0435771078395687,-0.482520308657719,
0.0344320600360783));
#30891=CARTESIAN_POINT('Ctrl Pts',(-0.0491283777357971,-0.467425290823089,
0.0200000000000001));
#30892=CARTESIAN_POINT('',(-0.0376715015669875,-0.498578838269023,0.295));
#30893=CARTESIAN_POINT('Origin',(-0.0900551232266954,-0.532437860018073,
0.6));
#30894=CARTESIAN_POINT('',(-0.066812080396678,-0.495516040015929,0.54));
#30895=CARTESIAN_POINT('Ctrl Pts',(-0.066812080396678,-0.495516040015929,
0.54));
#30896=CARTESIAN_POINT('Ctrl Pts',(-0.0576967697467444,-0.481036272390762,
0.555567939963916));
#30897=CARTESIAN_POINT('Ctrl Pts',(-0.0491283777357971,-0.467425290823089,
0.57));
#30898=CARTESIAN_POINT('',(-0.066812080396678,-0.495516040015929,0.05));
#30899=CARTESIAN_POINT('',(-0.066812080396678,-0.495516040015929,0.295));
#30900=CARTESIAN_POINT('Ctrl Pts',(-0.0491283777357971,-0.467425290823089,
0.0200000000000001));
#30901=CARTESIAN_POINT('Ctrl Pts',(-0.057696769746745,-0.481036272390763,
0.0344320600360851));
#30902=CARTESIAN_POINT('Ctrl Pts',(-0.0668120803966779,-0.495516040015929,
0.05));
#30903=CARTESIAN_POINT('Origin',(-0.235,-0.407031939778686,0.6));
#30904=CARTESIAN_POINT('',(-0.235,-0.407031939778686,0.57));
#30905=CARTESIAN_POINT('',(-0.237204912125273,-0.440152052890409,0.54));
#30906=CARTESIAN_POINT('Ctrl Pts',(-0.235,-0.407031939778686,0.57));
#30907=CARTESIAN_POINT('Ctrl Pts',(-0.23606835948338,-0.423079829636952,
0.555567939963917));
#30908=CARTESIAN_POINT('Ctrl Pts',(-0.237204912125273,-0.440152052890409,
0.54));
#30909=CARTESIAN_POINT('',(-0.235,-0.407031939778686,0.0200000000000001));
#30910=CARTESIAN_POINT('',(-0.235,-0.407031939778686,0.6));
#30911=CARTESIAN_POINT('',(-0.237204912125273,-0.440152052890409,0.05));
#30912=CARTESIAN_POINT('Ctrl Pts',(-0.237204912125273,-0.440152052890409,
0.05));
#30913=CARTESIAN_POINT('Ctrl Pts',(-0.236068359483381,-0.423079829636958,
0.0344320600360886));
#30914=CARTESIAN_POINT('Ctrl Pts',(-0.235,-0.407031939778686,0.0200000000000001));
#30915=CARTESIAN_POINT('',(-0.237204912125273,-0.440152052890409,0.295));
#30916=CARTESIAN_POINT('Origin',(-0.298831436591406,-0.449777469983454,
0.6));
#30917=CARTESIAN_POINT('',(-0.26258040326833,-0.425501506248146,0.54));
#30918=CARTESIAN_POINT('Ctrl Pts',(-0.26258040326833,-0.425501506248146,
0.54));
#30919=CARTESIAN_POINT('Ctrl Pts',(-0.248363700552694,-0.415981111160794,
0.555567939963927));
#30920=CARTESIAN_POINT('Ctrl Pts',(-0.235,-0.407031939778686,0.57));
#30921=CARTESIAN_POINT('',(-0.26258040326833,-0.425501506248146,0.05));
#30922=CARTESIAN_POINT('',(-0.26258040326833,-0.425501506248146,0.295));
#30923=CARTESIAN_POINT('Ctrl Pts',(-0.235,-0.407031939778686,0.0200000000000001));
#30924=CARTESIAN_POINT('Ctrl Pts',(-0.248363700552699,-0.415981111160797,
0.0344320600360783));
#30925=CARTESIAN_POINT('Ctrl Pts',(-0.26258040326833,-0.425501506248146,
0.05));
#30926=CARTESIAN_POINT('Origin',(-0.380237987356225,-0.276259068577462,
0.6));
#30927=CARTESIAN_POINT('',(-0.380237987356225,-0.276259068577462,0.57));
#30928=CARTESIAN_POINT('',(-0.395723438438122,-0.305618978911176,0.54));
#30929=CARTESIAN_POINT('Ctrl Pts',(-0.380237987356225,-0.276259068577462,
0.57));
#30930=CARTESIAN_POINT('Ctrl Pts',(-0.387741247158797,-0.290485004512361,
0.555567939963918));
#30931=CARTESIAN_POINT('Ctrl Pts',(-0.395723438438122,-0.305618978911176,
0.54));
#30932=CARTESIAN_POINT('',(-0.380237987356225,-0.276259068577462,0.0200000000000001));
#30933=CARTESIAN_POINT('',(-0.380237987356225,-0.276259068577462,0.6));
#30934=CARTESIAN_POINT('',(-0.395723438438122,-0.305618978911176,0.05));
#30935=CARTESIAN_POINT('Ctrl Pts',(-0.395723438438122,-0.305618978911176,
0.0500000000000001));
#30936=CARTESIAN_POINT('Ctrl Pts',(-0.387741247158801,-0.290485004512368,
0.0344320600360894));
#30937=CARTESIAN_POINT('Ctrl Pts',(-0.380237987356225,-0.276259068577462,
0.0200000000000001));
#30938=CARTESIAN_POINT('',(-0.395723438438122,-0.305618978911176,0.295));
#30939=CARTESIAN_POINT('Origin',(-0.455937079771088,-0.289346469288658,
0.6));
#30940=CARTESIAN_POINT('',(-0.412946188946813,-0.281913896490228,0.54));
#30941=CARTESIAN_POINT('Ctrl Pts',(-0.412946188946813,-0.281913896490228,
0.54));
#30942=CARTESIAN_POINT('Ctrl Pts',(-0.39608629121971,-0.278999036741381,
0.555567939963921));
#30943=CARTESIAN_POINT('Ctrl Pts',(-0.380237987356225,-0.276259068577462,
0.57));
#30944=CARTESIAN_POINT('',(-0.412946188946813,-0.281913896490228,0.05));
#30945=CARTESIAN_POINT('',(-0.412946188946813,-0.281913896490228,0.295));
#30946=CARTESIAN_POINT('Ctrl Pts',(-0.380237987356225,-0.276259068577462,
0.0200000000000001));
#30947=CARTESIAN_POINT('Ctrl Pts',(-0.396086291219724,-0.278999036741383,
0.0344320600360921));
#30948=CARTESIAN_POINT('Ctrl Pts',(-0.412946188946813,-0.281913896490228,
0.05));
#30949=CARTESIAN_POINT('Origin',(-0.459729372344889,-0.097718494684347,
0.6));
#30950=CARTESIAN_POINT('',(-0.459729372344889,-0.097718494684347,0.57));
#30951=CARTESIAN_POINT('',(-0.485817787210443,-0.11824160701694,0.54));
#30952=CARTESIAN_POINT('Ctrl Pts',(-0.459729372344889,-0.097718494684347,
0.57));
#30953=CARTESIAN_POINT('Ctrl Pts',(-0.472370150681811,-0.107662683134163,
0.55556793996392));
#30954=CARTESIAN_POINT('Ctrl Pts',(-0.485817787210443,-0.11824160701694,
0.54));
#30955=CARTESIAN_POINT('',(-0.459729372344889,-0.097718494684347,0.0200000000000001));
#30956=CARTESIAN_POINT('',(-0.459729372344889,-0.097718494684347,0.6));
#30957=CARTESIAN_POINT('',(-0.485817787210443,-0.11824160701694,0.05));
#30958=CARTESIAN_POINT('Ctrl Pts',(-0.485817787210443,-0.11824160701694,
0.0500000000000001));
#30959=CARTESIAN_POINT('Ctrl Pts',(-0.472370150681806,-0.107662683134159,
0.0344320600360745));
#30960=CARTESIAN_POINT('Ctrl Pts',(-0.459729372344889,-0.097718494684347,
0.0200000000000001));
#30961=CARTESIAN_POINT('',(-0.485817787210443,-0.11824160701694,0.295));
#30962=CARTESIAN_POINT('Origin',(-0.534207059800014,-0.0788848354237023,
0.6));
#30963=CARTESIAN_POINT('',(-0.491909827058038,-0.0895808129218024,0.54));
#30964=CARTESIAN_POINT('Ctrl Pts',(-0.491909827058038,-0.0895808129218024,
0.54));
#30965=CARTESIAN_POINT('Ctrl Pts',(-0.475321963803841,-0.0937754942427008,
0.555567939963922));
#30966=CARTESIAN_POINT('Ctrl Pts',(-0.459729372344889,-0.097718494684347,
0.57));
#30967=CARTESIAN_POINT('',(-0.491909827058038,-0.0895808129218024,0.05));
#30968=CARTESIAN_POINT('',(-0.491909827058038,-0.0895808129218024,0.295));
#30969=CARTESIAN_POINT('Ctrl Pts',(-0.459729372344889,-0.097718494684347,
0.0200000000000001));
#30970=CARTESIAN_POINT('Ctrl Pts',(-0.475321963803826,-0.0937754942427046,
0.0344320600360648));
#30971=CARTESIAN_POINT('Ctrl Pts',(-0.491909827058038,-0.0895808129218024,
0.0500000000000001));
#30972=CARTESIAN_POINT('Origin',(0.47,0.,0.6));
#30973=CARTESIAN_POINT('',(0.47,0.,0.57));
#30974=CARTESIAN_POINT('',(0.499785315393603,0.0146505466422634,0.54));
#30975=CARTESIAN_POINT('Ctrl Pts',(0.47,0.,0.57));
#30976=CARTESIAN_POINT('Ctrl Pts',(0.484432060036079,0.00709871847614981,
0.555567939963921));
#30977=CARTESIAN_POINT('Ctrl Pts',(0.499785315393603,0.0146505466422635,
0.54));
#30978=CARTESIAN_POINT('',(0.47,0.,0.0200000000000001));
#30979=CARTESIAN_POINT('',(0.47,0.,0.6));
#30980=CARTESIAN_POINT('',(0.499785315393603,0.0146505466422634,0.05));
#30981=CARTESIAN_POINT('Ctrl Pts',(0.499785315393603,0.0146505466422634,
0.05));
#30982=CARTESIAN_POINT('Ctrl Pts',(0.484432060036085,0.00709871847615275,
0.0344320600360846));
#30983=CARTESIAN_POINT('Ctrl Pts',(0.47,0.,0.0200000000000001));
#30984=CARTESIAN_POINT('',(0.499785315393603,0.0146505466422634,0.295));
#30985=CARTESIAN_POINT('Origin',(0.538934433351267,-0.0339068805458292,
0.6));
#30986=CARTESIAN_POINT('',(0.499785315393603,-0.0146505466422634,0.54));
#30987=CARTESIAN_POINT('Ctrl Pts',(0.499785315393603,-0.0146505466422635,
0.54));
#30988=CARTESIAN_POINT('Ctrl Pts',(0.48443206003608,-0.00709871847615054,
0.55556793996392));
#30989=CARTESIAN_POINT('Ctrl Pts',(0.47,0.,0.57));
#30990=CARTESIAN_POINT('',(0.499785315393603,-0.0146505466422634,0.05));
#30991=CARTESIAN_POINT('',(0.499785315393603,-0.0146505466422634,0.295));
#30992=CARTESIAN_POINT('Ctrl Pts',(0.47,0.,0.0200000000000001));
#30993=CARTESIAN_POINT('Ctrl Pts',(0.484432060036087,-0.00709871847615401,
0.0344320600360872));
#30994=CARTESIAN_POINT('Ctrl Pts',(0.499785315393603,-0.0146505466422634,
0.05));
#30995=CARTESIAN_POINT('Origin',(-0.429366365092022,0.191166222245626,0.6));
#30996=CARTESIAN_POINT('',(-0.429366365092022,0.191166222245626,0.57));
#30997=CARTESIAN_POINT('',(-0.4625355188348,0.189897061104753,0.54));
#30998=CARTESIAN_POINT('Ctrl Pts',(-0.429366365092022,0.191166222245626,
0.57));
#30999=CARTESIAN_POINT('Ctrl Pts',(-0.445438016905526,0.190551267878399,
0.555567939963931));
#31000=CARTESIAN_POINT('Ctrl Pts',(-0.4625355188348,0.189897061104753,0.54));
#31001=CARTESIAN_POINT('',(-0.429366365092022,0.191166222245626,0.0200000000000001));
#31002=CARTESIAN_POINT('',(-0.429366365092022,0.191166222245626,0.6));
#31003=CARTESIAN_POINT('',(-0.4625355188348,0.189897061104753,0.05));
#31004=CARTESIAN_POINT('Ctrl Pts',(-0.4625355188348,0.189897061104753,0.05));
#31005=CARTESIAN_POINT('Ctrl Pts',(-0.445438016905521,0.1905512678784,0.0344320600360647));
#31006=CARTESIAN_POINT('Ctrl Pts',(-0.429366365092022,0.191166222245626,
0.0200000000000001));
#31007=CARTESIAN_POINT('',(-0.4625355188348,0.189897061104753,0.295));
#31008=CARTESIAN_POINT('Origin',(-0.478549932784856,0.250179858964725,0.6));
#31009=CARTESIAN_POINT('',(-0.450617690513801,0.216664941778795,0.54));
#31010=CARTESIAN_POINT('Ctrl Pts',(-0.450617690513801,0.216664941778795,
0.54));
#31011=CARTESIAN_POINT('Ctrl Pts',(-0.439663399059279,0.203521271916341,
0.55556793996392));
#31012=CARTESIAN_POINT('Ctrl Pts',(-0.429366365092022,0.191166222245626,
0.57));
#31013=CARTESIAN_POINT('',(-0.450617690513801,0.216664941778795,0.05));
#31014=CARTESIAN_POINT('',(-0.450617690513801,0.216664941778795,0.295));
#31015=CARTESIAN_POINT('Ctrl Pts',(-0.429366365092022,0.191166222245626,
0.0200000000000001));
#31016=CARTESIAN_POINT('Ctrl Pts',(-0.439663399059263,0.203521271916321,
0.0344320600360574));
#31017=CARTESIAN_POINT('Ctrl Pts',(-0.450617690513801,0.216664941778795,
0.0500000000000001));
#31018=CARTESIAN_POINT('Origin',(-0.314491384988663,0.349278067974375,0.6));
#31019=CARTESIAN_POINT('',(-0.314491384988663,0.349278067974375,0.57));
#31020=CARTESIAN_POINT('',(-0.345309129066188,0.361609741826117,0.54));
#31021=CARTESIAN_POINT('Ctrl Pts',(-0.314491384988663,0.349278067974375,
0.57));
#31022=CARTESIAN_POINT('Ctrl Pts',(-0.329423693974693,0.355253208912853,
0.555567939963912));
#31023=CARTESIAN_POINT('Ctrl Pts',(-0.345309129066188,0.361609741826117,
0.54));
#31024=CARTESIAN_POINT('',(-0.314491384988663,0.349278067974375,0.0200000000000001));
#31025=CARTESIAN_POINT('',(-0.314491384988663,0.349278067974375,0.6));
#31026=CARTESIAN_POINT('',(-0.345309129066188,0.361609741826117,0.05));
#31027=CARTESIAN_POINT('Ctrl Pts',(-0.345309129066188,0.361609741826117,
0.05));
#31028=CARTESIAN_POINT('Ctrl Pts',(-0.32942369397468,0.355253208912848,
0.0344320600360755));
#31029=CARTESIAN_POINT('Ctrl Pts',(-0.314491384988663,0.349278067974375,
0.0200000000000001));
#31030=CARTESIAN_POINT('',(-0.345309129066188,0.361609741826117,0.295));
#31031=CARTESIAN_POINT('Origin',(-0.335419801350288,0.423194466955954,0.6));
#31032=CARTESIAN_POINT('',(-0.323534173210961,0.38121600014257,0.54));
#31033=CARTESIAN_POINT('Ctrl Pts',(-0.323534173210961,0.38121600014257,
0.54));
#31034=CARTESIAN_POINT('Ctrl Pts',(-0.318872942168541,0.364753148509483,
0.555567939963922));
#31035=CARTESIAN_POINT('Ctrl Pts',(-0.314491384988663,0.349278067974375,
0.57));
#31036=CARTESIAN_POINT('',(-0.323534173210961,0.38121600014257,0.05));
#31037=CARTESIAN_POINT('',(-0.323534173210961,0.38121600014257,0.295));
#31038=CARTESIAN_POINT('Ctrl Pts',(-0.314491384988663,0.349278067974375,
0.0200000000000001));
#31039=CARTESIAN_POINT('Ctrl Pts',(-0.318872942168539,0.364753148509479,
0.0344320600360749));
#31040=CARTESIAN_POINT('Ctrl Pts',(-0.323534173210961,0.38121600014257,
0.0500000000000001));
#31041=CARTESIAN_POINT('Origin',(-0.145237987356225,0.446996562658722,0.6));
#31042=CARTESIAN_POINT('',(-0.145237987356225,0.446996562658722,0.57));
#31043=CARTESIAN_POINT('',(-0.168375653847077,0.470796813064372,0.54));
#31044=CARTESIAN_POINT('Ctrl Pts',(-0.145237987356225,0.446996562658722,
0.57));
#31045=CARTESIAN_POINT('Ctrl Pts',(-0.156449021635303,0.458528642752187,
0.555567939963918));
#31046=CARTESIAN_POINT('Ctrl Pts',(-0.168375653847077,0.470796813064372,
0.54));
#31047=CARTESIAN_POINT('',(-0.145237987356225,0.446996562658722,0.0200000000000001));
#31048=CARTESIAN_POINT('',(-0.145237987356225,0.446996562658722,0.6));
#31049=CARTESIAN_POINT('',(-0.168375653847077,0.470796813064372,0.05));
#31050=CARTESIAN_POINT('Ctrl Pts',(-0.168375653847077,0.470796813064372,
0.05));
#31051=CARTESIAN_POINT('Ctrl Pts',(-0.156449021635315,0.458528642752199,
0.0344320600360975));
#31052=CARTESIAN_POINT('Ctrl Pts',(-0.145237987356225,0.446996562658722,
0.0200000000000001));
#31053=CARTESIAN_POINT('',(-0.168375653847077,0.470796813064372,0.295));
#31054=CARTESIAN_POINT('Origin',(-0.134292539069022,0.523034907009461,0.6));
#31055=CARTESIAN_POINT('',(-0.140508658144256,0.479851348843057,0.54));
#31056=CARTESIAN_POINT('Ctrl Pts',(-0.140508658144256,0.479851348843057,
0.54));
#31057=CARTESIAN_POINT('Ctrl Pts',(-0.142946456707125,0.462915892047018,
0.555567939963916));
#31058=CARTESIAN_POINT('Ctrl Pts',(-0.145237987356225,0.446996562658722,
0.57));
#31059=CARTESIAN_POINT('',(-0.140508658144256,0.479851348843057,0.05));
#31060=CARTESIAN_POINT('',(-0.140508658144256,0.479851348843057,0.295));
#31061=CARTESIAN_POINT('Ctrl Pts',(-0.145237987356225,0.446996562658722,
0.0200000000000001));
#31062=CARTESIAN_POINT('Ctrl Pts',(-0.142946456707125,0.462915892047015,
0.034432060036082));
#31063=CARTESIAN_POINT('Ctrl Pts',(-0.140508658144256,0.479851348843057,
0.0500000000000001));
#31064=CARTESIAN_POINT('Origin',(0.0491283777357971,0.467425290823088,0.6));
#31065=CARTESIAN_POINT('',(0.0491283777357971,0.467425290823088,0.57));
#31066=CARTESIAN_POINT('',(0.0376715015669876,0.498578838269023,0.54));
#31067=CARTESIAN_POINT('Ctrl Pts',(0.0491283777357971,0.467425290823088,
0.57));
#31068=CARTESIAN_POINT('Ctrl Pts',(0.0435771078395701,0.482520308657716,
0.555567939963925));
#31069=CARTESIAN_POINT('Ctrl Pts',(0.0376715015669876,0.498578838269023,
0.54));
#31070=CARTESIAN_POINT('',(0.0491283777357971,0.467425290823088,0.02));
#31071=CARTESIAN_POINT('',(0.0491283777357971,0.467425290823088,0.6));
#31072=CARTESIAN_POINT('',(0.0376715015669876,0.498578838269023,0.05));
#31073=CARTESIAN_POINT('Ctrl Pts',(0.0376715015669877,0.498578838269023,
0.05));
#31074=CARTESIAN_POINT('Ctrl Pts',(0.0435771078395647,0.48252030865773,
0.0344320600360888));
#31075=CARTESIAN_POINT('Ctrl Pts',(0.0491283777357971,0.467425290823088,
0.02));
#31076=CARTESIAN_POINT('',(0.0376715015669876,0.498578838269023,0.295));
#31077=CARTESIAN_POINT('Origin',(0.0900551232266951,0.532437860018073,0.6));
#31078=CARTESIAN_POINT('',(0.0668120803966779,0.495516040015929,0.54));
#31079=CARTESIAN_POINT('Ctrl Pts',(0.0668120803966779,0.495516040015929,
0.54));
#31080=CARTESIAN_POINT('Ctrl Pts',(0.0576967697467487,0.481036272390768,
0.555567939963909));
#31081=CARTESIAN_POINT('Ctrl Pts',(0.0491283777357971,0.467425290823088,
0.57));
#31082=CARTESIAN_POINT('',(0.0668120803966779,0.495516040015929,0.05));
#31083=CARTESIAN_POINT('',(0.0668120803966779,0.495516040015929,0.295));
#31084=CARTESIAN_POINT('Ctrl Pts',(0.0491283777357971,0.467425290823088,
0.02));
#31085=CARTESIAN_POINT('Ctrl Pts',(0.0576967697467307,0.48103627239074,
0.034432060036061));
#31086=CARTESIAN_POINT('Ctrl Pts',(0.0668120803966779,0.495516040015929,
0.05));
#31087=CARTESIAN_POINT('Origin',(0.235,0.407031939778686,0.6));
#31088=CARTESIAN_POINT('',(0.235,0.407031939778686,0.57));
#31089=CARTESIAN_POINT('',(0.237204912125272,0.440152052890409,0.54));
#31090=CARTESIAN_POINT('Ctrl Pts',(0.235,0.407031939778686,0.57));
#31091=CARTESIAN_POINT('Ctrl Pts',(0.236068359483379,0.423079829636944,
0.555567939963924));
#31092=CARTESIAN_POINT('Ctrl Pts',(0.237204912125272,0.440152052890409,
0.54));
#31093=CARTESIAN_POINT('',(0.235,0.407031939778686,0.0200000000000001));
#31094=CARTESIAN_POINT('',(0.235,0.407031939778686,0.6));
#31095=CARTESIAN_POINT('',(0.237204912125272,0.440152052890409,0.05));
#31096=CARTESIAN_POINT('Ctrl Pts',(0.237204912125272,0.440152052890409,
0.05));
#31097=CARTESIAN_POINT('Ctrl Pts',(0.236068359483379,0.423079829636941,
0.0344320600360727));
#31098=CARTESIAN_POINT('Ctrl Pts',(0.235,0.407031939778686,0.0200000000000001));
#31099=CARTESIAN_POINT('',(0.237204912125272,0.440152052890409,0.295));
#31100=CARTESIAN_POINT('Origin',(0.298831436591406,0.449777469983454,0.6));
#31101=CARTESIAN_POINT('',(0.26258040326833,0.425501506248146,0.54));
#31102=CARTESIAN_POINT('Ctrl Pts',(0.26258040326833,0.425501506248146,0.54));
#31103=CARTESIAN_POINT('Ctrl Pts',(0.24836370055269,0.415981111160792,0.555567939963931));
#31104=CARTESIAN_POINT('Ctrl Pts',(0.235,0.407031939778686,0.57));
#31105=CARTESIAN_POINT('',(0.26258040326833,0.425501506248146,0.05));
#31106=CARTESIAN_POINT('',(0.26258040326833,0.425501506248146,0.295));
#31107=CARTESIAN_POINT('Ctrl Pts',(0.235,0.407031939778686,0.0200000000000001));
#31108=CARTESIAN_POINT('Ctrl Pts',(0.248363700552713,0.415981111160807,
0.0344320600360936));
#31109=CARTESIAN_POINT('Ctrl Pts',(0.26258040326833,0.425501506248146,0.05));
#31110=CARTESIAN_POINT('Origin',(0.380237987356225,0.276259068577462,0.6));
#31111=CARTESIAN_POINT('',(0.380237987356225,0.276259068577462,0.57));
#31112=CARTESIAN_POINT('',(0.395723438438122,0.305618978911176,0.54));
#31113=CARTESIAN_POINT('Ctrl Pts',(0.380237987356225,0.276259068577462,
0.57));
#31114=CARTESIAN_POINT('Ctrl Pts',(0.387741247158792,0.29048500451235,0.555567939963929));
#31115=CARTESIAN_POINT('Ctrl Pts',(0.395723438438122,0.305618978911176,
0.54));
#31116=CARTESIAN_POINT('',(0.380237987356225,0.276259068577462,0.0200000000000001));
#31117=CARTESIAN_POINT('',(0.380237987356225,0.276259068577462,0.6));
#31118=CARTESIAN_POINT('',(0.395723438438122,0.305618978911176,0.05));
#31119=CARTESIAN_POINT('Ctrl Pts',(0.395723438438122,0.305618978911176,
0.05));
#31120=CARTESIAN_POINT('Ctrl Pts',(0.387741247158797,0.290485004512361,
0.034432060036082));
#31121=CARTESIAN_POINT('Ctrl Pts',(0.380237987356225,0.276259068577462,
0.0200000000000001));
#31122=CARTESIAN_POINT('',(0.395723438438122,0.305618978911176,0.295));
#31123=CARTESIAN_POINT('Origin',(0.455937079771088,0.289346469288658,0.6));
#31124=CARTESIAN_POINT('',(0.412946188946813,0.281913896490228,0.54));
#31125=CARTESIAN_POINT('Ctrl Pts',(0.412946188946813,0.281913896490228,
0.54));
#31126=CARTESIAN_POINT('Ctrl Pts',(0.396086291219718,0.278999036741382,
0.555567939963914));
#31127=CARTESIAN_POINT('Ctrl Pts',(0.380237987356225,0.276259068577462,
0.57));
#31128=CARTESIAN_POINT('',(0.412946188946813,0.281913896490228,0.05));
#31129=CARTESIAN_POINT('',(0.412946188946813,0.281913896490228,0.295));
#31130=CARTESIAN_POINT('Ctrl Pts',(0.380237987356225,0.276259068577462,
0.0200000000000001));
#31131=CARTESIAN_POINT('Ctrl Pts',(0.396086291219722,0.278999036741383,
0.0344320600360903));
#31132=CARTESIAN_POINT('Ctrl Pts',(0.412946188946813,0.281913896490228,
0.05));
#31133=CARTESIAN_POINT('Origin',(0.459729372344889,0.0977184946843469,0.6));
#31134=CARTESIAN_POINT('',(0.459729372344889,0.0977184946843469,0.57));
#31135=CARTESIAN_POINT('',(0.485817787210443,0.11824160701694,0.54));
#31136=CARTESIAN_POINT('Ctrl Pts',(0.459729372344889,0.0977184946843469,
0.57));
#31137=CARTESIAN_POINT('Ctrl Pts',(0.472370150681809,0.107662683134161,
0.555567939963922));
#31138=CARTESIAN_POINT('Ctrl Pts',(0.485817787210443,0.11824160701694,0.54));
#31139=CARTESIAN_POINT('',(0.459729372344889,0.0977184946843469,0.0200000000000001));
#31140=CARTESIAN_POINT('',(0.459729372344889,0.0977184946843469,0.6));
#31141=CARTESIAN_POINT('',(0.485817787210443,0.11824160701694,0.05));
#31142=CARTESIAN_POINT('Ctrl Pts',(0.485817787210443,0.11824160701694,0.0500000000000001));
#31143=CARTESIAN_POINT('Ctrl Pts',(0.472370150681813,0.107662683134164,
0.034432060036082));
#31144=CARTESIAN_POINT('Ctrl Pts',(0.459729372344889,0.0977184946843469,
0.0200000000000001));
#31145=CARTESIAN_POINT('',(0.485817787210443,0.11824160701694,0.295));
#31146=CARTESIAN_POINT('Origin',(0.534207059800014,0.0788848354237023,0.6));
#31147=CARTESIAN_POINT('',(0.491909827058038,0.0895808129218023,0.54));
#31148=CARTESIAN_POINT('Ctrl Pts',(0.491909827058038,0.0895808129218023,
0.54));
#31149=CARTESIAN_POINT('Ctrl Pts',(0.475321963803841,0.0937754942427007,
0.555567939963922));
#31150=CARTESIAN_POINT('Ctrl Pts',(0.459729372344889,0.0977184946843469,
0.57));
#31151=CARTESIAN_POINT('',(0.491909827058038,0.0895808129218023,0.05));
#31152=CARTESIAN_POINT('',(0.491909827058038,0.0895808129218023,0.295));
#31153=CARTESIAN_POINT('Ctrl Pts',(0.459729372344889,0.0977184946843469,
0.0200000000000001));
#31154=CARTESIAN_POINT('Ctrl Pts',(0.475321963803834,0.0937754942427024,
0.0344320600360725));
#31155=CARTESIAN_POINT('Ctrl Pts',(0.491909827058038,0.0895808129218023,
0.05));
#31156=CARTESIAN_POINT('Origin',(0.429366365092022,0.191166222245626,0.6));
#31157=CARTESIAN_POINT('',(0.429366365092022,0.191166222245626,0.57));
#31158=CARTESIAN_POINT('',(0.450617690513801,0.216664941778795,0.54));
#31159=CARTESIAN_POINT('Ctrl Pts',(0.429366365092022,0.191166222245626,
0.57));
#31160=CARTESIAN_POINT('Ctrl Pts',(0.439663399059275,0.203521271916335,
0.555567939963926));
#31161=CARTESIAN_POINT('Ctrl Pts',(0.450617690513801,0.216664941778795,
0.54));
#31162=CARTESIAN_POINT('',(0.429366365092022,0.191166222245626,0.02));
#31163=CARTESIAN_POINT('',(0.429366365092022,0.191166222245626,0.6));
#31164=CARTESIAN_POINT('',(0.450617690513801,0.216664941778795,0.05));
#31165=CARTESIAN_POINT('Ctrl Pts',(0.450617690513801,0.216664941778795,
0.05));
#31166=CARTESIAN_POINT('Ctrl Pts',(0.439663399059281,0.203521271916343,
0.0344320600360824));
#31167=CARTESIAN_POINT('Ctrl Pts',(0.429366365092022,0.191166222245626,
0.02));
#31168=CARTESIAN_POINT('',(0.450617690513801,0.216664941778795,0.295));
#31169=CARTESIAN_POINT('Origin',(0.506132274325621,0.18822890555378,0.6));
#31170=CARTESIAN_POINT('',(0.4625355188348,0.189897061104753,0.54));
#31171=CARTESIAN_POINT('Ctrl Pts',(0.4625355188348,0.189897061104753,0.54));
#31172=CARTESIAN_POINT('Ctrl Pts',(0.445438016905532,0.190551267878399,
0.555567939963925));
#31173=CARTESIAN_POINT('Ctrl Pts',(0.429366365092022,0.191166222245626,
0.57));
#31174=CARTESIAN_POINT('',(0.4625355188348,0.189897061104753,0.05));
#31175=CARTESIAN_POINT('',(0.4625355188348,0.189897061104753,0.295));
#31176=CARTESIAN_POINT('Ctrl Pts',(0.429366365092022,0.191166222245626,
0.02));
#31177=CARTESIAN_POINT('Ctrl Pts',(0.445438016905514,0.1905512678784,0.0344320600360582));
#31178=CARTESIAN_POINT('Ctrl Pts',(0.4625355188348,0.189897061104753,0.05));
#31179=CARTESIAN_POINT('Origin',(0.314491384988663,0.349278067974375,0.6));
#31180=CARTESIAN_POINT('',(0.314491384988663,0.349278067974375,0.57));
#31181=CARTESIAN_POINT('',(0.323534173210961,0.38121600014257,0.54));
#31182=CARTESIAN_POINT('Ctrl Pts',(0.314491384988663,0.349278067974375,
0.57));
#31183=CARTESIAN_POINT('Ctrl Pts',(0.318872942168541,0.364753148509485,
0.55556793996392));
#31184=CARTESIAN_POINT('Ctrl Pts',(0.323534173210961,0.38121600014257,0.54));
#31185=CARTESIAN_POINT('',(0.314491384988663,0.349278067974375,0.0200000000000001));
#31186=CARTESIAN_POINT('',(0.314491384988663,0.349278067974375,0.6));
#31187=CARTESIAN_POINT('',(0.323534173210961,0.38121600014257,0.05));
#31188=CARTESIAN_POINT('Ctrl Pts',(0.323534173210961,0.38121600014257,0.05));
#31189=CARTESIAN_POINT('Ctrl Pts',(0.318872942168541,0.364753148509485,
0.03443206003608));
#31190=CARTESIAN_POINT('Ctrl Pts',(0.314491384988663,0.349278067974375,
0.0200000000000001));
#31191=CARTESIAN_POINT('',(0.323534173210961,0.38121600014257,0.295));
#31192=CARTESIAN_POINT('Origin',(0.385815247001714,0.377818203877217,0.6));
#31193=CARTESIAN_POINT('',(0.345309129066188,0.361609741826117,0.54));
#31194=CARTESIAN_POINT('Ctrl Pts',(0.345309129066188,0.361609741826117,
0.54));
#31195=CARTESIAN_POINT('Ctrl Pts',(0.32942369397469,0.355253208912852,0.555567939963916));
#31196=CARTESIAN_POINT('Ctrl Pts',(0.314491384988663,0.349278067974375,
0.57));
#31197=CARTESIAN_POINT('',(0.345309129066188,0.361609741826117,0.05));
#31198=CARTESIAN_POINT('',(0.345309129066188,0.361609741826117,0.295));
#31199=CARTESIAN_POINT('Ctrl Pts',(0.314491384988663,0.349278067974375,
0.0200000000000001));
#31200=CARTESIAN_POINT('Ctrl Pts',(0.329423693974684,0.355253208912849,
0.0344320600360788));
#31201=CARTESIAN_POINT('Ctrl Pts',(0.345309129066188,0.361609741826117,
0.0500000000000001));
#31202=CARTESIAN_POINT('Origin',(0.145237987356225,0.446996562658722,0.6));
#31203=CARTESIAN_POINT('',(0.145237987356225,0.446996562658722,0.57));
#31204=CARTESIAN_POINT('',(0.140508658144256,0.479851348843056,0.54));
#31205=CARTESIAN_POINT('Ctrl Pts',(0.145237987356225,0.446996562658722,
0.57));
#31206=CARTESIAN_POINT('Ctrl Pts',(0.142946456707127,0.462915892047007,
0.555567939963926));
#31207=CARTESIAN_POINT('Ctrl Pts',(0.140508658144256,0.479851348843057,
0.54));
#31208=CARTESIAN_POINT('',(0.145237987356225,0.446996562658722,0.0199999999999999));
#31209=CARTESIAN_POINT('',(0.145237987356225,0.446996562658722,0.6));
#31210=CARTESIAN_POINT('',(0.140508658144256,0.479851348843056,0.05));
#31211=CARTESIAN_POINT('Ctrl Pts',(0.140508658144256,0.479851348843057,
0.05));
#31212=CARTESIAN_POINT('Ctrl Pts',(0.142946456707125,0.462915892047022,
0.0344320600360881));
#31213=CARTESIAN_POINT('Ctrl Pts',(0.145237987356225,0.446996562658722,
0.0199999999999999));
#31214=CARTESIAN_POINT('',(0.140508658144256,0.479851348843056,0.295));
#31215=CARTESIAN_POINT('Origin',(0.198787258449726,0.502079302379656,0.6));
#31216=CARTESIAN_POINT('',(0.168375653847077,0.470796813064372,0.54));
#31217=CARTESIAN_POINT('Ctrl Pts',(0.168375653847077,0.470796813064372,
0.54));
#31218=CARTESIAN_POINT('Ctrl Pts',(0.156449021635289,0.458528642752173,
0.555567939963936));
#31219=CARTESIAN_POINT('Ctrl Pts',(0.145237987356225,0.446996562658722,
0.57));
#31220=CARTESIAN_POINT('',(0.168375653847077,0.470796813064372,0.05));
#31221=CARTESIAN_POINT('',(0.168375653847077,0.470796813064372,0.295));
#31222=CARTESIAN_POINT('Ctrl Pts',(0.145237987356225,0.446996562658722,
0.0199999999999999));
#31223=CARTESIAN_POINT('Ctrl Pts',(0.156449021635309,0.458528642752193,
0.0344320600360905));
#31224=CARTESIAN_POINT('Ctrl Pts',(0.168375653847077,0.470796813064372,
0.05));
#31225=CARTESIAN_POINT('Origin',(-0.0491283777357972,0.467425290823088,
0.6));
#31226=CARTESIAN_POINT('',(-0.0491283777357972,0.467425290823088,0.57));
#31227=CARTESIAN_POINT('',(-0.0668120803966779,0.495516040015929,0.54));
#31228=CARTESIAN_POINT('Ctrl Pts',(-0.0491283777357972,0.467425290823088,
0.57));
#31229=CARTESIAN_POINT('Ctrl Pts',(-0.0576967697467437,0.48103627239076,
0.555567939963917));
#31230=CARTESIAN_POINT('Ctrl Pts',(-0.0668120803966779,0.495516040015929,
0.54));
#31231=CARTESIAN_POINT('',(-0.0491283777357972,0.467425290823088,0.02));
#31232=CARTESIAN_POINT('',(-0.0491283777357972,0.467425290823088,0.6));
#31233=CARTESIAN_POINT('',(-0.0668120803966779,0.495516040015929,0.05));
#31234=CARTESIAN_POINT('Ctrl Pts',(-0.0668120803966779,0.495516040015929,
0.05));
#31235=CARTESIAN_POINT('Ctrl Pts',(-0.057696769746748,0.481036272390767,
0.0344320600360899));
#31236=CARTESIAN_POINT('Ctrl Pts',(-0.0491283777357972,0.467425290823088,
0.02));
#31237=CARTESIAN_POINT('',(-0.0668120803966779,0.495516040015929,0.295));
#31238=CARTESIAN_POINT('Origin',(-0.0226128530137678,0.539526328253384,
0.6));
#31239=CARTESIAN_POINT('',(-0.0376715015669876,0.498578838269023,0.54));
#31240=CARTESIAN_POINT('Ctrl Pts',(-0.0376715015669876,0.498578838269023,
0.54));
#31241=CARTESIAN_POINT('Ctrl Pts',(-0.0435771078395712,0.482520308657713,
0.555567939963928));
#31242=CARTESIAN_POINT('Ctrl Pts',(-0.0491283777357972,0.467425290823088,
0.57));
#31243=CARTESIAN_POINT('',(-0.0376715015669876,0.498578838269023,0.05));
#31244=CARTESIAN_POINT('',(-0.0376715015669876,0.498578838269023,0.295));
#31245=CARTESIAN_POINT('Ctrl Pts',(-0.0491283777357972,0.467425290823088,
0.02));
#31246=CARTESIAN_POINT('Ctrl Pts',(-0.0435771078395706,0.482520308657714,
0.0344320600360737));
#31247=CARTESIAN_POINT('Ctrl Pts',(-0.0376715015669877,0.498578838269023,
0.0500000000000001));
#31248=CARTESIAN_POINT('Origin',(-0.235,0.407031939778686,0.6));
#31249=CARTESIAN_POINT('',(-0.235,0.407031939778686,0.57));
#31250=CARTESIAN_POINT('',(-0.26258040326833,0.425501506248146,0.54));
#31251=CARTESIAN_POINT('Ctrl Pts',(-0.235,0.407031939778686,0.57));
#31252=CARTESIAN_POINT('Ctrl Pts',(-0.248363700552695,0.415981111160795,
0.555567939963926));
#31253=CARTESIAN_POINT('Ctrl Pts',(-0.26258040326833,0.425501506248146,
0.54));
#31254=CARTESIAN_POINT('',(-0.235,0.407031939778686,0.02));
#31255=CARTESIAN_POINT('',(-0.235,0.407031939778686,0.6));
#31256=CARTESIAN_POINT('',(-0.26258040326833,0.425501506248146,0.05));
#31257=CARTESIAN_POINT('Ctrl Pts',(-0.26258040326833,0.425501506248146,
0.05));
#31258=CARTESIAN_POINT('Ctrl Pts',(-0.248363700552693,0.415981111160794,
0.0344320600360725));
#31259=CARTESIAN_POINT('Ctrl Pts',(-0.235,0.407031939778686,0.02));
#31260=CARTESIAN_POINT('',(-0.26258040326833,0.425501506248146,0.295));
#31261=CARTESIAN_POINT('Origin',(-0.240102996759861,0.483684350529283,0.6));
#31262=CARTESIAN_POINT('',(-0.237204912125272,0.440152052890409,0.54));
#31263=CARTESIAN_POINT('Ctrl Pts',(-0.237204912125272,0.44015205289041,
0.54));
#31264=CARTESIAN_POINT('Ctrl Pts',(-0.23606835948338,0.423079829636946,
0.555567939963922));
#31265=CARTESIAN_POINT('Ctrl Pts',(-0.235,0.407031939778686,0.57));
#31266=CARTESIAN_POINT('',(-0.237204912125272,0.440152052890409,0.05));
#31267=CARTESIAN_POINT('',(-0.237204912125272,0.440152052890409,0.295));
#31268=CARTESIAN_POINT('Ctrl Pts',(-0.235,0.407031939778686,0.02));
#31269=CARTESIAN_POINT('Ctrl Pts',(-0.236068359483379,0.423079829636939,
0.034432060036071));
#31270=CARTESIAN_POINT('Ctrl Pts',(-0.237204912125272,0.440152052890409,
0.05));
#31271=CARTESIAN_POINT('Origin',(-0.380237987356225,0.276259068577462,0.6));
#31272=CARTESIAN_POINT('',(-0.380237987356225,0.276259068577462,0.57));
#31273=CARTESIAN_POINT('',(-0.412946188946813,0.281913896490228,0.54));
#31274=CARTESIAN_POINT('Ctrl Pts',(-0.380237987356225,0.276259068577462,
0.57));
#31275=CARTESIAN_POINT('Ctrl Pts',(-0.396086291219706,0.27899903674138,
0.555567939963925));
#31276=CARTESIAN_POINT('Ctrl Pts',(-0.412946188946813,0.281913896490228,
0.54));
#31277=CARTESIAN_POINT('',(-0.380237987356225,0.276259068577462,0.0200000000000001));
#31278=CARTESIAN_POINT('',(-0.380237987356225,0.276259068577462,0.6));
#31279=CARTESIAN_POINT('',(-0.412946188946813,0.281913896490228,0.05));
#31280=CARTESIAN_POINT('Ctrl Pts',(-0.412946188946813,0.281913896490228,
0.05));
#31281=CARTESIAN_POINT('Ctrl Pts',(-0.396086291219709,0.27899903674138,
0.0344320600360784));
#31282=CARTESIAN_POINT('Ctrl Pts',(-0.380237987356225,0.276259068577462,
0.0200000000000001));
#31283=CARTESIAN_POINT('',(-0.412946188946813,0.281913896490228,0.295));
#31284=CARTESIAN_POINT('Origin',(-0.416077151098926,0.344208954464292,0.6));
#31285=CARTESIAN_POINT('',(-0.395723438438122,0.305618978911176,0.54));
#31286=CARTESIAN_POINT('Ctrl Pts',(-0.395723438438122,0.305618978911176,
0.54));
#31287=CARTESIAN_POINT('Ctrl Pts',(-0.387741247158798,0.290485004512363,
0.555567939963916));
#31288=CARTESIAN_POINT('Ctrl Pts',(-0.380237987356225,0.276259068577462,
0.57));
#31289=CARTESIAN_POINT('',(-0.395723438438122,0.305618978911176,0.05));
#31290=CARTESIAN_POINT('',(-0.395723438438122,0.305618978911176,0.295));
#31291=CARTESIAN_POINT('Ctrl Pts',(-0.380237987356225,0.276259068577462,
0.0200000000000001));
#31292=CARTESIAN_POINT('Ctrl Pts',(-0.387741247158788,0.290485004512343,
0.0344320600360639));
#31293=CARTESIAN_POINT('Ctrl Pts',(-0.395723438438122,0.305618978911176,
0.05));
#31294=CARTESIAN_POINT('Origin',(-0.459729372344889,0.0977184946843469,
0.6));
#31295=CARTESIAN_POINT('',(-0.459729372344889,0.0977184946843469,0.57));
#31296=CARTESIAN_POINT('',(-0.491909827058038,0.0895808129218024,0.54));
#31297=CARTESIAN_POINT('Ctrl Pts',(-0.459729372344889,0.0977184946843469,
0.57));
#31298=CARTESIAN_POINT('Ctrl Pts',(-0.47532196380384,0.0937754942427011,
0.555567939963923));
#31299=CARTESIAN_POINT('Ctrl Pts',(-0.491909827058038,0.0895808129218025,
0.54));
#31300=CARTESIAN_POINT('',(-0.459729372344889,0.0977184946843469,0.0200000000000001));
#31301=CARTESIAN_POINT('',(-0.459729372344889,0.0977184946843469,0.6));
#31302=CARTESIAN_POINT('',(-0.491909827058038,0.0895808129218024,0.05));
#31303=CARTESIAN_POINT('Ctrl Pts',(-0.491909827058038,0.0895808129218025,
0.05));
#31304=CARTESIAN_POINT('Ctrl Pts',(-0.47532196380385,0.0937754942426984,
0.0344320600360872));
#31305=CARTESIAN_POINT('Ctrl Pts',(-0.459729372344889,0.0977184946843469,
0.0200000000000001));
#31306=CARTESIAN_POINT('',(-0.491909827058038,0.0895808129218024,0.295));
#31307=CARTESIAN_POINT('Origin',(-0.520107786070735,0.145216703132244,0.6));
#31308=CARTESIAN_POINT('',(-0.485817787210443,0.11824160701694,0.54));
#31309=CARTESIAN_POINT('Ctrl Pts',(-0.485817787210443,0.11824160701694,
0.54));
#31310=CARTESIAN_POINT('Ctrl Pts',(-0.47237015068181,0.107662683134162,
0.555567939963921));
#31311=CARTESIAN_POINT('Ctrl Pts',(-0.459729372344889,0.0977184946843469,
0.57));
#31312=CARTESIAN_POINT('',(-0.485817787210443,0.11824160701694,0.05));
#31313=CARTESIAN_POINT('',(-0.485817787210443,0.11824160701694,0.295));
#31314=CARTESIAN_POINT('Ctrl Pts',(-0.459729372344889,0.0977184946843469,
0.0200000000000001));
#31315=CARTESIAN_POINT('Ctrl Pts',(-0.472370150681809,0.107662683134161,
0.0344320600360776));
#31316=CARTESIAN_POINT('Ctrl Pts',(-0.485817787210443,0.11824160701694,
0.05));
#31317=CARTESIAN_POINT('Origin',(-0.47,5.75583995599256E-17,0.6));
#31318=CARTESIAN_POINT('',(-0.47,5.75583995599256E-17,0.57));
#31319=CARTESIAN_POINT('',(-0.499785315393603,-0.0146505466422634,0.54));
#31320=CARTESIAN_POINT('Ctrl Pts',(-0.47,5.75583995599256E-17,0.57));
#31321=CARTESIAN_POINT('Ctrl Pts',(-0.484432060036081,-0.0070987184761509,
0.555567939963919));
#31322=CARTESIAN_POINT('Ctrl Pts',(-0.499785315393603,-0.0146505466422634,
0.54));
#31323=CARTESIAN_POINT('',(-0.47,5.75583995599256E-17,0.0200000000000001));
#31324=CARTESIAN_POINT('',(-0.47,5.75583995599256E-17,0.6));
#31325=CARTESIAN_POINT('',(-0.499785315393603,-0.0146505466422634,0.05));
#31326=CARTESIAN_POINT('Ctrl Pts',(-0.499785315393603,-0.0146505466422634,
0.05));
#31327=CARTESIAN_POINT('Ctrl Pts',(-0.484432060036073,-0.00709871847614705,
0.0344320600360732));
#31328=CARTESIAN_POINT('Ctrl Pts',(-0.47,5.75583995599256E-17,0.0200000000000001));
#31329=CARTESIAN_POINT('',(-0.499785315393603,-0.0146505466422634,0.295));
#31330=CARTESIAN_POINT('Origin',(-0.538934433351267,0.0339068805458291,
0.6));
#31331=CARTESIAN_POINT('',(-0.499785315393603,0.0146505466422634,0.54));
#31332=CARTESIAN_POINT('Ctrl Pts',(-0.499785315393603,0.0146505466422635,
0.54));
#31333=CARTESIAN_POINT('Ctrl Pts',(-0.48443206003608,0.00709871847615045,
0.55556793996392));
#31334=CARTESIAN_POINT('Ctrl Pts',(-0.47,5.75583995599256E-17,0.57));
#31335=CARTESIAN_POINT('',(-0.499785315393603,0.0146505466422634,0.05));
#31336=CARTESIAN_POINT('',(-0.499785315393603,0.0146505466422634,0.295));
#31337=CARTESIAN_POINT('Ctrl Pts',(-0.47,5.75583995599256E-17,0.0200000000000001));
#31338=CARTESIAN_POINT('Ctrl Pts',(-0.484432060036083,0.007098718476152,
0.0344320600360831));
#31339=CARTESIAN_POINT('Ctrl Pts',(-0.499785315393603,0.0146505466422634,
0.05));
#31340=CARTESIAN_POINT('Origin',(-0.429366365092022,-0.191166222245626,
0.6));
#31341=CARTESIAN_POINT('',(-0.429366365092022,-0.191166222245626,0.57));
#31342=CARTESIAN_POINT('',(-0.450617690513801,-0.216664941778795,0.54));
#31343=CARTESIAN_POINT('Ctrl Pts',(-0.429366365092022,-0.191166222245626,
0.57));
#31344=CARTESIAN_POINT('Ctrl Pts',(-0.439663399059279,-0.20352127191634,
0.55556793996392));
#31345=CARTESIAN_POINT('Ctrl Pts',(-0.450617690513801,-0.216664941778795,
0.54));
#31346=CARTESIAN_POINT('',(-0.429366365092022,-0.191166222245626,0.02));
#31347=CARTESIAN_POINT('',(-0.429366365092022,-0.191166222245626,0.6));
#31348=CARTESIAN_POINT('',(-0.450617690513801,-0.216664941778795,0.05));
#31349=CARTESIAN_POINT('Ctrl Pts',(-0.450617690513801,-0.216664941778795,
0.05));
#31350=CARTESIAN_POINT('Ctrl Pts',(-0.439663399059269,-0.203521271916329,
0.0344320600360665));
#31351=CARTESIAN_POINT('Ctrl Pts',(-0.429366365092022,-0.191166222245626,
0.02));
#31352=CARTESIAN_POINT('',(-0.450617690513801,-0.216664941778795,0.295));
#31353=CARTESIAN_POINT('Origin',(-0.506132274325621,-0.18822890555378,0.6));
#31354=CARTESIAN_POINT('',(-0.4625355188348,-0.189897061104753,0.54));
#31355=CARTESIAN_POINT('Ctrl Pts',(-0.4625355188348,-0.189897061104753,
0.54));
#31356=CARTESIAN_POINT('Ctrl Pts',(-0.445438016905532,-0.190551267878399,
0.555567939963925));
#31357=CARTESIAN_POINT('Ctrl Pts',(-0.429366365092022,-0.191166222245626,
0.57));
#31358=CARTESIAN_POINT('',(-0.4625355188348,-0.189897061104753,0.05));
#31359=CARTESIAN_POINT('',(-0.4625355188348,-0.189897061104753,0.295));
#31360=CARTESIAN_POINT('Ctrl Pts',(-0.429366365092022,-0.191166222245626,
0.02));
#31361=CARTESIAN_POINT('Ctrl Pts',(-0.445438016905514,-0.1905512678784,
0.0344320600360582));
#31362=CARTESIAN_POINT('Ctrl Pts',(-0.4625355188348,-0.189897061104753,
0.05));
#31363=CARTESIAN_POINT('Origin',(-0.314491384988663,-0.349278067974375,
0.6));
#31364=CARTESIAN_POINT('',(-0.314491384988663,-0.349278067974375,0.57));
#31365=CARTESIAN_POINT('',(-0.323534173210961,-0.38121600014257,0.54));
#31366=CARTESIAN_POINT('Ctrl Pts',(-0.314491384988663,-0.349278067974375,
0.57));
#31367=CARTESIAN_POINT('Ctrl Pts',(-0.318872942168543,-0.364753148509492,
0.555567939963913));
#31368=CARTESIAN_POINT('Ctrl Pts',(-0.323534173210961,-0.38121600014257,
0.54));
#31369=CARTESIAN_POINT('',(-0.314491384988663,-0.349278067974375,0.0200000000000001));
#31370=CARTESIAN_POINT('',(-0.314491384988663,-0.349278067974375,0.6));
#31371=CARTESIAN_POINT('',(-0.323534173210961,-0.38121600014257,0.05));
#31372=CARTESIAN_POINT('Ctrl Pts',(-0.323534173210961,-0.38121600014257,
0.05));
#31373=CARTESIAN_POINT('Ctrl Pts',(-0.318872942168548,-0.364753148509509,
0.0344320600361024));
#31374=CARTESIAN_POINT('Ctrl Pts',(-0.314491384988663,-0.349278067974375,
0.0200000000000001));
#31375=CARTESIAN_POINT('',(-0.323534173210961,-0.38121600014257,0.295));
#31376=CARTESIAN_POINT('Origin',(-0.385815247001714,-0.377818203877217,
0.6));
#31377=CARTESIAN_POINT('',(-0.345309129066188,-0.361609741826117,0.54));
#31378=CARTESIAN_POINT('Ctrl Pts',(-0.345309129066188,-0.361609741826117,
0.54));
#31379=CARTESIAN_POINT('Ctrl Pts',(-0.32942369397469,-0.355253208912852,
0.555567939963916));
#31380=CARTESIAN_POINT('Ctrl Pts',(-0.314491384988663,-0.349278067974375,
0.57));
#31381=CARTESIAN_POINT('',(-0.345309129066188,-0.361609741826117,0.05));
#31382=CARTESIAN_POINT('',(-0.345309129066188,-0.361609741826117,0.295));
#31383=CARTESIAN_POINT('Ctrl Pts',(-0.314491384988663,-0.349278067974375,
0.0200000000000001));
#31384=CARTESIAN_POINT('Ctrl Pts',(-0.329423693974684,-0.355253208912849,
0.0344320600360788));
#31385=CARTESIAN_POINT('Ctrl Pts',(-0.345309129066188,-0.361609741826117,
0.0500000000000001));
#31386=CARTESIAN_POINT('Origin',(-0.145237987356225,-0.446996562658722,
0.6));
#31387=CARTESIAN_POINT('',(-0.145237987356225,-0.446996562658722,0.57));
#31388=CARTESIAN_POINT('',(-0.140508658144256,-0.479851348843057,0.54));
#31389=CARTESIAN_POINT('Ctrl Pts',(-0.145237987356225,-0.446996562658722,
0.57));
#31390=CARTESIAN_POINT('Ctrl Pts',(-0.142946456707126,-0.462915892047014,
0.555567939963919));
#31391=CARTESIAN_POINT('Ctrl Pts',(-0.140508658144256,-0.479851348843057,
0.54));
#31392=CARTESIAN_POINT('',(-0.145237987356225,-0.446996562658722,0.02));
#31393=CARTESIAN_POINT('',(-0.145237987356225,-0.446996562658722,0.6));
#31394=CARTESIAN_POINT('',(-0.140508658144256,-0.479851348843057,0.05));
#31395=CARTESIAN_POINT('Ctrl Pts',(-0.140508658144256,-0.479851348843057,
0.05));
#31396=CARTESIAN_POINT('Ctrl Pts',(-0.142946456707126,-0.462915892047012,
0.0344320600360792));
#31397=CARTESIAN_POINT('Ctrl Pts',(-0.145237987356225,-0.446996562658722,
0.02));
#31398=CARTESIAN_POINT('',(-0.140508658144256,-0.479851348843057,0.295));
#31399=CARTESIAN_POINT('Origin',(-0.198787258449726,-0.502079302379656,
0.6));
#31400=CARTESIAN_POINT('',(-0.168375653847077,-0.470796813064372,0.54));
#31401=CARTESIAN_POINT('Ctrl Pts',(-0.168375653847077,-0.470796813064372,
0.54));
#31402=CARTESIAN_POINT('Ctrl Pts',(-0.156449021635299,-0.458528642752182,
0.555567939963923));
#31403=CARTESIAN_POINT('Ctrl Pts',(-0.145237987356225,-0.446996562658722,
0.57));
#31404=CARTESIAN_POINT('',(-0.168375653847077,-0.470796813064372,0.05));
#31405=CARTESIAN_POINT('',(-0.168375653847077,-0.470796813064372,0.295));
#31406=CARTESIAN_POINT('Ctrl Pts',(-0.145237987356225,-0.446996562658722,
0.02));
#31407=CARTESIAN_POINT('Ctrl Pts',(-0.156449021635308,-0.458528642752192,
0.0344320600360887));
#31408=CARTESIAN_POINT('Ctrl Pts',(-0.168375653847077,-0.470796813064372,
0.05));
#31409=CARTESIAN_POINT('Origin',(0.0491283777357969,-0.467425290823089,
0.6));
#31410=CARTESIAN_POINT('',(0.0491283777357969,-0.467425290823089,0.57));
#31411=CARTESIAN_POINT('',(0.0668120803966778,-0.495516040015929,0.54));
#31412=CARTESIAN_POINT('Ctrl Pts',(0.0491283777357969,-0.467425290823089,
0.57));
#31413=CARTESIAN_POINT('Ctrl Pts',(0.0576967697467424,-0.481036272390759,
0.555567939963919));
#31414=CARTESIAN_POINT('Ctrl Pts',(0.0668120803966778,-0.495516040015929,
0.54));
#31415=CARTESIAN_POINT('',(0.0491283777357969,-0.467425290823089,0.0200000000000001));
#31416=CARTESIAN_POINT('',(0.0491283777357969,-0.467425290823089,0.6));
#31417=CARTESIAN_POINT('',(0.0668120803966778,-0.495516040015929,0.05));
#31418=CARTESIAN_POINT('Ctrl Pts',(0.0668120803966778,-0.495516040015929,
0.05));
#31419=CARTESIAN_POINT('Ctrl Pts',(0.0576967697467371,-0.48103627239075,
0.0344320600360721));
#31420=CARTESIAN_POINT('Ctrl Pts',(0.0491283777357969,-0.467425290823089,
0.0200000000000001));
#31421=CARTESIAN_POINT('',(0.0668120803966778,-0.495516040015929,0.295));
#31422=CARTESIAN_POINT('Origin',(0.0226128530137677,-0.539526328253384,
0.6));
#31423=CARTESIAN_POINT('',(0.0376715015669875,-0.498578838269023,0.54));
#31424=CARTESIAN_POINT('Ctrl Pts',(0.0376715015669875,-0.498578838269023,
0.54));
#31425=CARTESIAN_POINT('Ctrl Pts',(0.0435771078395709,-0.482520308657713,
0.555567939963928));
#31426=CARTESIAN_POINT('Ctrl Pts',(0.0491283777357969,-0.467425290823089,
0.57));
#31427=CARTESIAN_POINT('',(0.0376715015669875,-0.498578838269023,0.05));
#31428=CARTESIAN_POINT('',(0.0376715015669875,-0.498578838269023,0.295));
#31429=CARTESIAN_POINT('Ctrl Pts',(0.0491283777357969,-0.467425290823089,
0.0200000000000001));
#31430=CARTESIAN_POINT('Ctrl Pts',(0.0435771078395724,-0.482520308657709,
0.0344320600360687));
#31431=CARTESIAN_POINT('Ctrl Pts',(0.0376715015669875,-0.498578838269023,
0.0500000000000001));
#31432=CARTESIAN_POINT('Origin',(0.235,-0.407031939778686,0.6));
#31433=CARTESIAN_POINT('',(0.235,-0.407031939778686,0.57));
#31434=CARTESIAN_POINT('',(0.26258040326833,-0.425501506248146,0.54));
#31435=CARTESIAN_POINT('Ctrl Pts',(0.235,-0.407031939778686,0.57));
#31436=CARTESIAN_POINT('Ctrl Pts',(0.2483637005527,-0.415981111160798,0.555567939963921));
#31437=CARTESIAN_POINT('Ctrl Pts',(0.26258040326833,-0.425501506248146,
0.54));
#31438=CARTESIAN_POINT('',(0.235,-0.407031939778686,0.0200000000000001));
#31439=CARTESIAN_POINT('',(0.235,-0.407031939778686,0.6));
#31440=CARTESIAN_POINT('',(0.26258040326833,-0.425501506248146,0.05));
#31441=CARTESIAN_POINT('Ctrl Pts',(0.26258040326833,-0.425501506248146,
0.05));
#31442=CARTESIAN_POINT('Ctrl Pts',(0.248363700552693,-0.415981111160793,
0.0344320600360718));
#31443=CARTESIAN_POINT('Ctrl Pts',(0.235,-0.407031939778686,0.0200000000000001));
#31444=CARTESIAN_POINT('',(0.26258040326833,-0.425501506248146,0.295));
#31445=CARTESIAN_POINT('Origin',(0.240102996759861,-0.483684350529283,0.6));
#31446=CARTESIAN_POINT('',(0.237204912125272,-0.440152052890409,0.54));
#31447=CARTESIAN_POINT('Ctrl Pts',(0.237204912125272,-0.44015205289041,
0.54));
#31448=CARTESIAN_POINT('Ctrl Pts',(0.23606835948338,-0.423079829636952,
0.555567939963918));
#31449=CARTESIAN_POINT('Ctrl Pts',(0.235,-0.407031939778686,0.57));
#31450=CARTESIAN_POINT('',(0.237204912125272,-0.440152052890409,0.05));
#31451=CARTESIAN_POINT('',(0.237204912125272,-0.440152052890409,0.295));
#31452=CARTESIAN_POINT('Ctrl Pts',(0.235,-0.407031939778686,0.0200000000000001));
#31453=CARTESIAN_POINT('Ctrl Pts',(0.236068359483379,-0.423079829636935,
0.0344320600360673));
#31454=CARTESIAN_POINT('Ctrl Pts',(0.237204912125272,-0.440152052890409,
0.05));
#31455=CARTESIAN_POINT('Origin',(0.380237987356225,-0.276259068577463,0.6));
#31456=CARTESIAN_POINT('',(0.380237987356225,-0.276259068577463,0.57));
#31457=CARTESIAN_POINT('',(0.412946188946813,-0.281913896490228,0.54));
#31458=CARTESIAN_POINT('Ctrl Pts',(0.380237987356225,-0.276259068577463,
0.57));
#31459=CARTESIAN_POINT('Ctrl Pts',(0.3960862912197,-0.278999036741379,0.55556793996393));
#31460=CARTESIAN_POINT('Ctrl Pts',(0.412946188946813,-0.281913896490228,
0.54));
#31461=CARTESIAN_POINT('',(0.380237987356225,-0.276259068577462,0.0200000000000001));
#31462=CARTESIAN_POINT('',(0.380237987356225,-0.276259068577463,0.6));
#31463=CARTESIAN_POINT('',(0.412946188946813,-0.281913896490228,0.05));
#31464=CARTESIAN_POINT('Ctrl Pts',(0.412946188946813,-0.281913896490228,
0.05));
#31465=CARTESIAN_POINT('Ctrl Pts',(0.396086291219706,-0.27899903674138,
0.0344320600360757));
#31466=CARTESIAN_POINT('Ctrl Pts',(0.380237987356225,-0.276259068577462,
0.0200000000000001));
#31467=CARTESIAN_POINT('',(0.412946188946813,-0.281913896490228,0.295));
#31468=CARTESIAN_POINT('Origin',(0.416077151098926,-0.344208954464293,0.6));
#31469=CARTESIAN_POINT('',(0.395723438438122,-0.305618978911176,0.54));
#31470=CARTESIAN_POINT('Ctrl Pts',(0.395723438438122,-0.305618978911176,
0.54));
#31471=CARTESIAN_POINT('Ctrl Pts',(0.387741247158795,-0.290485004512358,
0.555567939963921));
#31472=CARTESIAN_POINT('Ctrl Pts',(0.380237987356225,-0.276259068577463,
0.57));
#31473=CARTESIAN_POINT('',(0.395723438438122,-0.305618978911176,0.05));
#31474=CARTESIAN_POINT('',(0.395723438438122,-0.305618978911176,0.295));
#31475=CARTESIAN_POINT('Ctrl Pts',(0.380237987356225,-0.276259068577462,
0.0200000000000001));
#31476=CARTESIAN_POINT('Ctrl Pts',(0.387741247158799,-0.290485004512365,
0.0344320600360857));
#31477=CARTESIAN_POINT('Ctrl Pts',(0.395723438438122,-0.305618978911176,
0.05));
#31478=CARTESIAN_POINT('Origin',(0.459729372344889,-0.0977184946843472,
0.6));
#31479=CARTESIAN_POINT('',(0.459729372344889,-0.0977184946843472,0.57));
#31480=CARTESIAN_POINT('',(0.491909827058038,-0.0895808129218025,0.54));
#31481=CARTESIAN_POINT('Ctrl Pts',(0.459729372344889,-0.0977184946843472,
0.57));
#31482=CARTESIAN_POINT('Ctrl Pts',(0.475321963803834,-0.0937754942427026,
0.555567939963928));
#31483=CARTESIAN_POINT('Ctrl Pts',(0.491909827058038,-0.0895808129218025,
0.54));
#31484=CARTESIAN_POINT('',(0.459729372344889,-0.0977184946843472,0.0200000000000001));
#31485=CARTESIAN_POINT('',(0.459729372344889,-0.0977184946843472,0.6));
#31486=CARTESIAN_POINT('',(0.491909827058038,-0.0895808129218025,0.05));
#31487=CARTESIAN_POINT('Ctrl Pts',(0.491909827058038,-0.0895808129218025,
0.05));
#31488=CARTESIAN_POINT('Ctrl Pts',(0.475321963803832,-0.0937754942427031,
0.034432060036071));
#31489=CARTESIAN_POINT('Ctrl Pts',(0.459729372344889,-0.0977184946843472,
0.0200000000000001));
#31490=CARTESIAN_POINT('',(0.491909827058038,-0.0895808129218025,0.295));
#31491=CARTESIAN_POINT('Origin',(0.520107786070735,-0.145216703132244,0.6));
#31492=CARTESIAN_POINT('',(0.485817787210443,-0.11824160701694,0.54));
#31493=CARTESIAN_POINT('Ctrl Pts',(0.485817787210443,-0.11824160701694,
0.54));
#31494=CARTESIAN_POINT('Ctrl Pts',(0.472370150681812,-0.107662683134164,
0.555567939963919));
#31495=CARTESIAN_POINT('Ctrl Pts',(0.459729372344889,-0.0977184946843472,
0.57));
#31496=CARTESIAN_POINT('',(0.485817787210443,-0.11824160701694,0.05));
#31497=CARTESIAN_POINT('',(0.485817787210443,-0.11824160701694,0.295));
#31498=CARTESIAN_POINT('Ctrl Pts',(0.459729372344889,-0.0977184946843472,
0.0200000000000001));
#31499=CARTESIAN_POINT('Ctrl Pts',(0.4723701506818,-0.107662683134155,0.0344320600360681));
#31500=CARTESIAN_POINT('Ctrl Pts',(0.485817787210443,-0.11824160701694,
0.05));
#31501=CARTESIAN_POINT('Origin',(0.,0.,0.295));
#31502=CARTESIAN_POINT('Origin',(0.,0.,0.05));
#31503=CARTESIAN_POINT('Origin',(0.,0.,0.54));
#31504=CARTESIAN_POINT('Origin',(0.,0.,0.295));
#31505=CARTESIAN_POINT('Origin',(0.,0.,0.05));
#31506=CARTESIAN_POINT('Origin',(0.,0.,0.54));
#31507=CARTESIAN_POINT('Origin',(0.,0.,0.295));
#31508=CARTESIAN_POINT('Origin',(0.,0.,0.54));
#31509=CARTESIAN_POINT('Origin',(0.,0.,0.05));
#31510=CARTESIAN_POINT('Origin',(0.,0.,0.295));
#31511=CARTESIAN_POINT('Origin',(0.,0.,0.05));
#31512=CARTESIAN_POINT('Origin',(0.,0.,0.54));
#31513=CARTESIAN_POINT('Origin',(0.,0.,0.295));
#31514=CARTESIAN_POINT('Origin',(0.,0.,0.54));
#31515=CARTESIAN_POINT('Origin',(0.,0.,0.05));
#31516=CARTESIAN_POINT('Origin',(0.,0.,0.295));
#31517=CARTESIAN_POINT('Origin',(0.,0.,0.05));
#31518=CARTESIAN_POINT('Origin',(0.,0.,0.54));
#31519=CARTESIAN_POINT('Origin',(0.,0.,0.295));
#31520=CARTESIAN_POINT('Origin',(0.,0.,0.54));
#31521=CARTESIAN_POINT('Origin',(0.,0.,0.05));
#31522=CARTESIAN_POINT('Origin',(0.,0.,0.295));
#31523=CARTESIAN_POINT('Origin',(0.,0.,0.05));
#31524=CARTESIAN_POINT('Origin',(0.,0.,0.54));
#31525=CARTESIAN_POINT('Origin',(0.,0.,0.295));
#31526=CARTESIAN_POINT('Origin',(0.,0.,0.54));
#31527=CARTESIAN_POINT('Origin',(0.,0.,0.05));
#31528=CARTESIAN_POINT('Origin',(0.,0.,0.295));
#31529=CARTESIAN_POINT('Origin',(0.,0.,0.05));
#31530=CARTESIAN_POINT('Origin',(0.,0.,0.54));
#31531=CARTESIAN_POINT('Origin',(0.,0.,0.295));
#31532=CARTESIAN_POINT('Origin',(0.,0.,0.54));
#31533=CARTESIAN_POINT('Origin',(0.,0.,0.05));
#31534=CARTESIAN_POINT('Origin',(0.,0.,0.295));
#31535=CARTESIAN_POINT('Origin',(0.,0.,0.05));
#31536=CARTESIAN_POINT('Origin',(0.,0.,0.54));
#31537=CARTESIAN_POINT('Origin',(0.,0.,0.295));
#31538=CARTESIAN_POINT('Origin',(0.,0.,0.54));
#31539=CARTESIAN_POINT('Origin',(0.,0.,0.05));
#31540=CARTESIAN_POINT('Origin',(0.,0.,0.295));
#31541=CARTESIAN_POINT('Origin',(0.,0.,0.05));
#31542=CARTESIAN_POINT('Origin',(0.,0.,0.54));
#31543=CARTESIAN_POINT('Origin',(0.,0.,0.295));
#31544=CARTESIAN_POINT('Origin',(0.,0.,0.54));
#31545=CARTESIAN_POINT('Origin',(0.,0.,0.05));
#31546=CARTESIAN_POINT('Origin',(0.,0.,0.295));
#31547=CARTESIAN_POINT('Origin',(0.,0.,0.05));
#31548=CARTESIAN_POINT('Origin',(0.,0.,0.54));
#31549=CARTESIAN_POINT('Origin',(0.,0.,0.295));
#31550=CARTESIAN_POINT('Origin',(0.,0.,0.54));
#31551=CARTESIAN_POINT('Origin',(0.,0.,0.05));
#31552=CARTESIAN_POINT('Origin',(0.,0.,0.295));
#31553=CARTESIAN_POINT('Origin',(0.,0.,0.05));
#31554=CARTESIAN_POINT('Origin',(0.,0.,0.54));
#31555=CARTESIAN_POINT('Origin',(0.,0.,0.295));
#31556=CARTESIAN_POINT('Origin',(0.,0.,0.54));
#31557=CARTESIAN_POINT('Origin',(0.,0.,0.05));
#31558=CARTESIAN_POINT('Origin',(0.,0.,0.295));
#31559=CARTESIAN_POINT('Origin',(0.,0.,0.05));
#31560=CARTESIAN_POINT('Origin',(0.,0.,0.54));
#31561=CARTESIAN_POINT('Origin',(0.,0.,0.295));
#31562=CARTESIAN_POINT('Origin',(0.,0.,0.54));
#31563=CARTESIAN_POINT('Origin',(0.,0.,0.05));
#31564=CARTESIAN_POINT('Origin',(0.,0.,0.295));
#31565=CARTESIAN_POINT('Origin',(0.,0.,0.05));
#31566=CARTESIAN_POINT('Origin',(0.,0.,0.54));
#31567=CARTESIAN_POINT('Origin',(0.,0.,0.295));
#31568=CARTESIAN_POINT('Origin',(0.,0.,0.54));
#31569=CARTESIAN_POINT('Origin',(0.,0.,0.05));
#31570=CARTESIAN_POINT('Origin',(0.,0.,0.295));
#31571=CARTESIAN_POINT('Origin',(0.,0.,0.05));
#31572=CARTESIAN_POINT('Origin',(0.,0.,0.54));
#31573=CARTESIAN_POINT('Origin',(0.,0.,0.295));
#31574=CARTESIAN_POINT('Origin',(0.,0.,0.54));
#31575=CARTESIAN_POINT('Origin',(0.,0.,0.05));
#31576=CARTESIAN_POINT('Origin',(0.,0.,0.295));
#31577=CARTESIAN_POINT('Origin',(0.,0.,0.05));
#31578=CARTESIAN_POINT('Origin',(0.,0.,0.54));
#31579=CARTESIAN_POINT('Origin',(0.,0.,0.295));
#31580=CARTESIAN_POINT('Origin',(0.,0.,0.54));
#31581=CARTESIAN_POINT('Origin',(0.,0.,0.05));
#31582=CARTESIAN_POINT('Origin',(0.,0.,0.295));
#31583=CARTESIAN_POINT('Origin',(0.,0.,0.05));
#31584=CARTESIAN_POINT('Origin',(0.,0.,0.54));
#31585=CARTESIAN_POINT('Origin',(0.,0.,0.295));
#31586=CARTESIAN_POINT('Origin',(0.,0.,0.54));
#31587=CARTESIAN_POINT('Origin',(0.,0.,0.05));
#31588=CARTESIAN_POINT('Origin',(0.,0.,0.295));
#31589=CARTESIAN_POINT('Origin',(0.,0.,0.05));
#31590=CARTESIAN_POINT('Origin',(0.,0.,0.54));
#31591=CARTESIAN_POINT('Origin',(0.,0.,0.025));
#31592=CARTESIAN_POINT('',(-0.45,-5.51091059616309E-17,2.42861286636753E-17));
#31593=CARTESIAN_POINT('',(-0.475,-5.81707229594993E-17,0.025));
#31594=CARTESIAN_POINT('Origin',(0.,0.,0.));
#31595=CARTESIAN_POINT('Origin',(0.21,0.,-1.2));
#31596=CARTESIAN_POINT('',(-0.21,-2.57175827820944E-17,-1.2));
#31597=CARTESIAN_POINT('Origin',(0.,0.,-1.2));
#31598=CARTESIAN_POINT('Origin',(0.,0.,-1.18));
#31599=CARTESIAN_POINT('',(-0.23,-2.81668763803891E-17,-1.18));
#31600=CARTESIAN_POINT('Origin',(0.,0.,-0.58));
#31601=CARTESIAN_POINT('Origin',(0.,0.,0.));
#31602=CARTESIAN_POINT('Origin',(0.45,0.,0.));
#31603=CARTESIAN_POINT('Origin',(0.,0.,0.57));
#31604=CARTESIAN_POINT('',(-0.44,-5.38844591624836E-17,0.6));
#31605=CARTESIAN_POINT('Origin',(0.,0.,0.6));
#31606=CARTESIAN_POINT('',(-0.47,-5.75583995599256E-17,0.57));
#31607=CARTESIAN_POINT('Origin',(0.,0.,0.6));
#38590=UNCERTAINTY_MEASURE_WITH_UNIT(LENGTH_MEASURE(0.001),#38612,
'DISTANCE_ACCURACY_VALUE',
'Maximum model space distance between geometric entities at asserted c
onnectivities');
#38595=UNCERTAINTY_MEASURE_WITH_UNIT(LENGTH_MEASURE(0.001),#38612,
'DISTANCE_ACCURACY_VALUE',
'Maximum model space distance between geometric entities at asserted c
onnectivities');
#38606=(
GEOMETRIC_REPRESENTATION_CONTEXT(3)
GLOBAL_UNCERTAINTY_ASSIGNED_CONTEXT((#38590))
GLOBAL_UNIT_ASSIGNED_CONTEXT((#38612,#38614,#38615))
REPRESENTATION_CONTEXT('','3D')
);
#38611=(
GEOMETRIC_REPRESENTATION_CONTEXT(3)
GLOBAL_UNCERTAINTY_ASSIGNED_CONTEXT((#38595))
GLOBAL_UNIT_ASSIGNED_CONTEXT((#38612,#38614,#38615))
REPRESENTATION_CONTEXT('','3D')
);
#38612=(
LENGTH_UNIT()
NAMED_UNIT(*)
SI_UNIT(.CENTI.,.METRE.)
);
#38614=(
NAMED_UNIT(*)
PLANE_ANGLE_UNIT()
SI_UNIT($,.RADIAN.)
);
#38615=(
NAMED_UNIT(*)
SI_UNIT($,.STERADIAN.)
SOLID_ANGLE_UNIT()
);
#38626=SHAPE_DEFINITION_REPRESENTATION(#38641,#38677);
#38641=PRODUCT_DEFINITION_SHAPE('',$,#38693);
#38677=SHAPE_REPRESENTATION('',(#17098),#38606);
#38682=PRODUCT_DEFINITION_CONTEXT('part definition',#38729,'design');
#38693=PRODUCT_DEFINITION('2026-10-19-02-31-37-420',
'08_Brass_Knurled_Fine_Adjust_Screw_M5x0.5x12',#38708,#38682);
#38708=PRODUCT_DEFINITION_FORMATION('',$,#38741);
#38729=APPLICATION_CONTEXT(
'Core Data for Automotive Mechanical Design Process');
#38730=PRODUCT_CONTEXT('part definition',#38729,'mechanical');
#38741=PRODUCT('2026-10-19-02-31-37-420',
'08_Brass_Knurled_Fine_Adjust_Screw_M5x0.5x12',$,(#38730));
#38879=COLOUR_RGB('Black',0.12,0.14,0.17);
#38880=FILL_AREA_STYLE_COLOUR('',#38879);
#38881=FILL_AREA_STYLE('',(#38880));
#38882=SURFACE_STYLE_FILL_AREA(#38881);
#38883=SURFACE_SIDE_STYLE('',(#38882));
#38884=SURFACE_STYLE_USAGE(.BOTH.,#38883);
#38885=PRESENTATION_STYLE_ASSIGNMENT((#38884));
ENDSEC;
END-ISO-10303-21;
